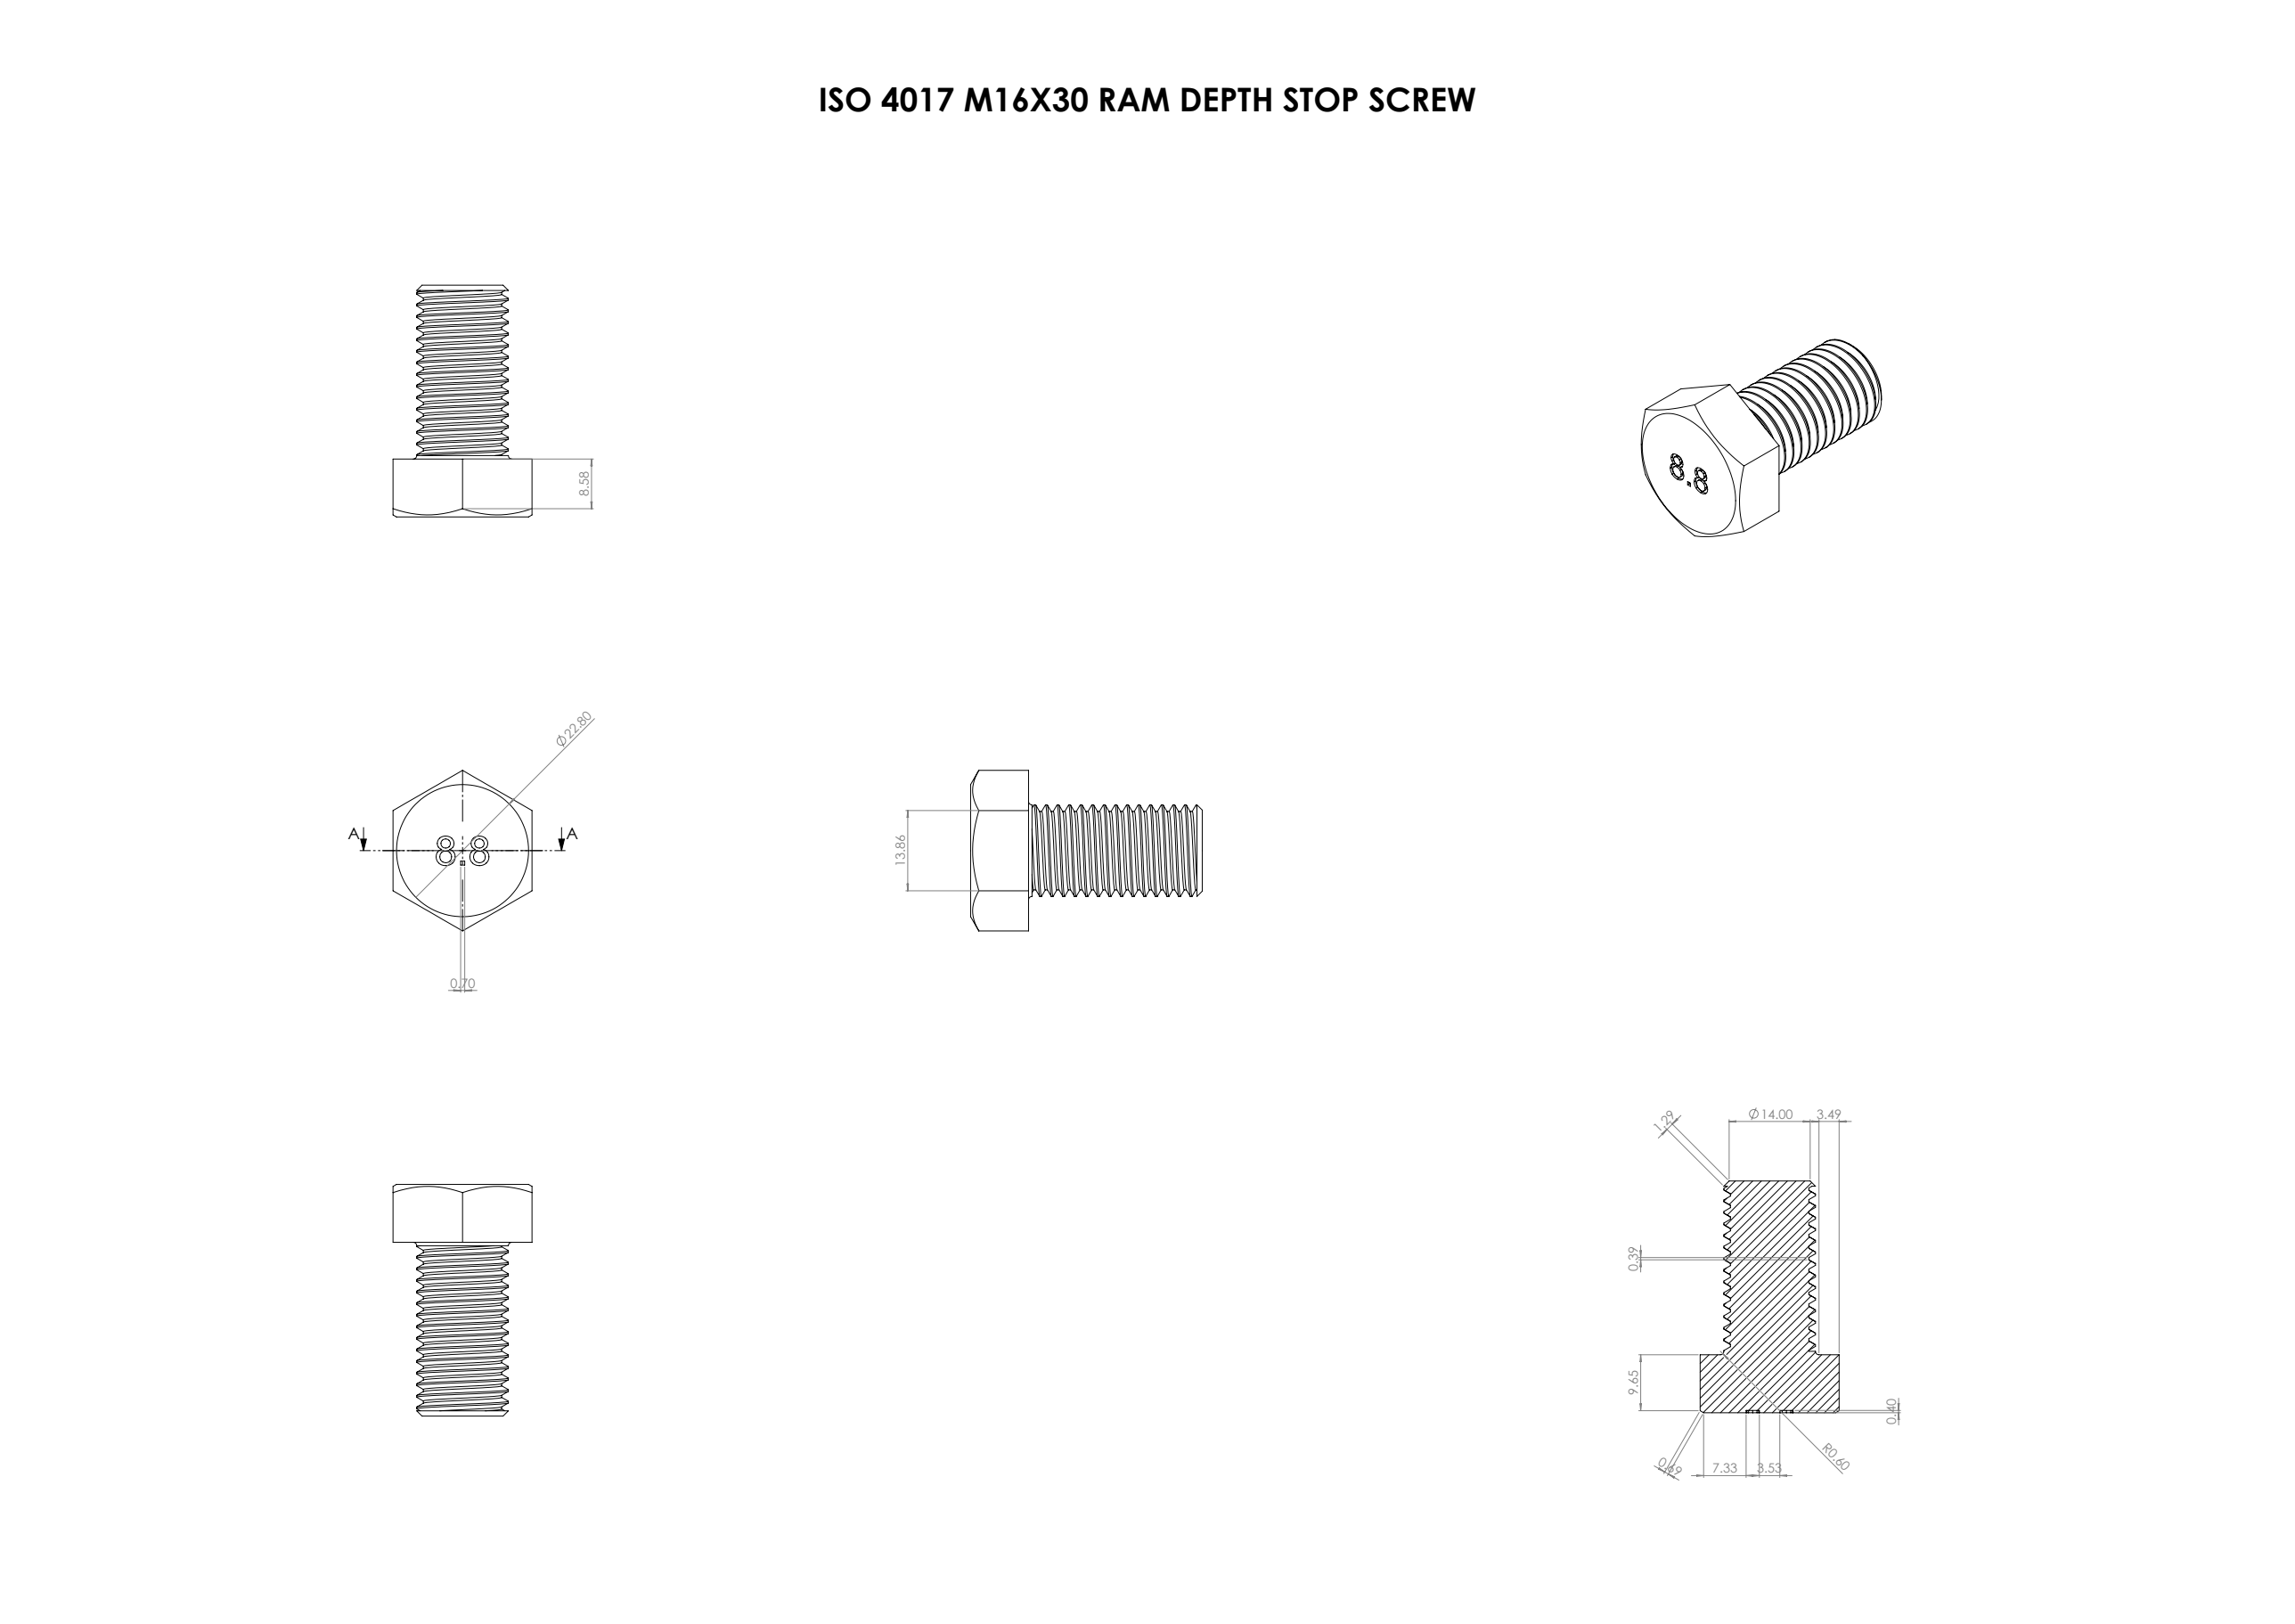
ISO-10303-21;
HEADER;
/* Generated by software containing ST-Developer
 * from STEP Tools, Inc. (www.steptools.com) 
 */

FILE_DESCRIPTION(
/* description */ (''),
/* implementation_level */ '2;1');

FILE_NAME(
/* name */ '13_ISO_4017_M16x30_Ram_Depth_Stop_Screw.step',
/* time_stamp */ '2026-10-19T23:58:09-07:00',
/* author */ (''),
/* organization */ (''),
/* preprocessor_version */ 'ST-DEVELOPER v20.2',
/* originating_system */ 'Autodesk Translation Framework v15.15.0.0',
/* authorisation */ '');

FILE_SCHEMA (('AP203_CONFIGURATION_CONTROLLED_3D_DESIGN_OF_MECHANICAL_PARTS_AND_ASSEMBLIES_MIM_LF { 1 0 10303 203 3 1 4 }',
'AUTOMOTIVE_DESIGN { 1 0 10303 214 3 1 1 }','INTEGRATED_CNC_SCHEMA','MODEL_BASED_INTEGRATED_MANUFACTURING_SCHEMA',
'PROCESS_PLANNING_SCHEMA','AP242_MANAGED_MODEL_BASED_3D_ENGINEERING_MIM_LF { 1 0 10303 442 3 1 4 }'));
ENDSEC;

DATA;
#10=MECHANICAL_DESIGN_GEOMETRIC_PRESENTATION_REPRESENTATION('',(#466),#70757);
#170=TOROIDAL_SURFACE('',#28944,0.8511,0.06);
#263=(
BOUNDED_CURVE()
B_SPLINE_CURVE(2,(#70654,#70655,#70656),.UNSPECIFIED.,.F.,.F.)
B_SPLINE_CURVE_WITH_KNOTS((3,3),(0.0830692064483412,1.5163968327409),
 .UNSPECIFIED.)
CURVE()
GEOMETRIC_REPRESENTATION_ITEM()
RATIONAL_B_SPLINE_CURVE((1.01933756729741,1.17702963774851,1.01933756729741))
REPRESENTATION_ITEM('')
);
#264=(
BOUNDED_CURVE()
B_SPLINE_CURVE(2,(#70658,#70659,#70660),.UNSPECIFIED.,.F.,.F.)
B_SPLINE_CURVE_WITH_KNOTS((3,3),(0.0830692064483407,1.5163968327409),
 .UNSPECIFIED.)
CURVE()
GEOMETRIC_REPRESENTATION_ITEM()
RATIONAL_B_SPLINE_CURVE((1.01933756729741,1.17702963774851,1.01933756729741))
REPRESENTATION_ITEM('')
);
#265=(
BOUNDED_CURVE()
B_SPLINE_CURVE(2,(#70662,#70663,#70664),.UNSPECIFIED.,.F.,.F.)
B_SPLINE_CURVE_WITH_KNOTS((3,3),(0.0830692064483414,1.5163968327409),
 .UNSPECIFIED.)
CURVE()
GEOMETRIC_REPRESENTATION_ITEM()
RATIONAL_B_SPLINE_CURVE((1.01933756729741,1.17702963774851,1.01933756729741))
REPRESENTATION_ITEM('')
);
#266=(
BOUNDED_CURVE()
B_SPLINE_CURVE(2,(#70666,#70667,#70668),.UNSPECIFIED.,.F.,.F.)
B_SPLINE_CURVE_WITH_KNOTS((3,3),(0.0830692064483412,1.5163968327409),
 .UNSPECIFIED.)
CURVE()
GEOMETRIC_REPRESENTATION_ITEM()
RATIONAL_B_SPLINE_CURVE((1.01933756729741,1.17702963774851,1.01933756729741))
REPRESENTATION_ITEM('')
);
#267=(
BOUNDED_CURVE()
B_SPLINE_CURVE(2,(#70670,#70671,#70672),.UNSPECIFIED.,.F.,.F.)
B_SPLINE_CURVE_WITH_KNOTS((3,3),(0.799733019594622,1.5163968327409),
 .UNSPECIFIED.)
CURVE()
GEOMETRIC_REPRESENTATION_ITEM()
RATIONAL_B_SPLINE_CURVE((1.09818360252296,1.09818360252296,1.01933756729741))
REPRESENTATION_ITEM('')
);
#268=(
BOUNDED_CURVE()
B_SPLINE_CURVE(2,(#70677,#70678,#70679),.UNSPECIFIED.,.F.,.F.)
B_SPLINE_CURVE_WITH_KNOTS((3,3),(0.083069206448341,0.799733019594622),
 .UNSPECIFIED.)
CURVE()
GEOMETRIC_REPRESENTATION_ITEM()
RATIONAL_B_SPLINE_CURVE((1.01933756729741,1.09818360252296,1.09818360252296))
REPRESENTATION_ITEM('')
);
#269=(
BOUNDED_CURVE()
B_SPLINE_CURVE(2,(#70680,#70681,#70682),.UNSPECIFIED.,.F.,.F.)
B_SPLINE_CURVE_WITH_KNOTS((3,3),(0.0830692064483408,1.5163968327409),
 .UNSPECIFIED.)
CURVE()
GEOMETRIC_REPRESENTATION_ITEM()
RATIONAL_B_SPLINE_CURVE((1.01933756729741,1.17702963774851,1.01933756729741))
REPRESENTATION_ITEM('')
);
#309=B_SPLINE_SURFACE_WITH_KNOTS('',2,1,((#67768,#67769),(#67770,#67771),
(#67772,#67773)),.UNSPECIFIED.,.F.,.F.,.F.,(3,3),(2,2),(0.,1.),(0.,0.04),
 .UNSPECIFIED.);
#310=B_SPLINE_SURFACE_WITH_KNOTS('',2,1,((#67786,#67787),(#67788,#67789),
(#67790,#67791)),.UNSPECIFIED.,.F.,.F.,.F.,(3,3),(2,2),(0.,1.),(0.,0.04),
 .UNSPECIFIED.);
#311=B_SPLINE_SURFACE_WITH_KNOTS('',2,1,((#67801,#67802),(#67803,#67804),
(#67805,#67806)),.UNSPECIFIED.,.F.,.F.,.F.,(3,3),(2,2),(0.,1.),(0.,0.04),
 .UNSPECIFIED.);
#312=B_SPLINE_SURFACE_WITH_KNOTS('',2,1,((#67816,#67817),(#67818,#67819),
(#67820,#67821)),.UNSPECIFIED.,.F.,.F.,.F.,(3,3),(2,2),(0.,1.),(0.,0.04),
 .UNSPECIFIED.);
#313=B_SPLINE_SURFACE_WITH_KNOTS('',2,1,((#67831,#67832),(#67833,#67834),
(#67835,#67836)),.UNSPECIFIED.,.F.,.F.,.F.,(3,3),(2,2),(0.,1.),(0.,0.04),
 .UNSPECIFIED.);
#314=B_SPLINE_SURFACE_WITH_KNOTS('',2,1,((#67846,#67847),(#67848,#67849),
(#67850,#67851)),.UNSPECIFIED.,.F.,.F.,.F.,(3,3),(2,2),(0.,1.),(0.,0.04),
 .UNSPECIFIED.);
#315=B_SPLINE_SURFACE_WITH_KNOTS('',2,1,((#67861,#67862),(#67863,#67864),
(#67865,#67866)),.UNSPECIFIED.,.F.,.F.,.F.,(3,3),(2,2),(0.,1.),(0.,0.04),
 .UNSPECIFIED.);
#316=B_SPLINE_SURFACE_WITH_KNOTS('',2,1,((#67876,#67877),(#67878,#67879),
(#67880,#67881)),.UNSPECIFIED.,.F.,.F.,.F.,(3,3),(2,2),(0.,1.),(0.,0.04),
 .UNSPECIFIED.);
#317=B_SPLINE_SURFACE_WITH_KNOTS('',2,1,((#67888,#67889),(#67890,#67891),
(#67892,#67893)),.UNSPECIFIED.,.F.,.F.,.F.,(3,3),(2,2),(0.,1.),(0.,0.04),
 .UNSPECIFIED.);
#318=B_SPLINE_SURFACE_WITH_KNOTS('',2,1,((#67906,#67907),(#67908,#67909),
(#67910,#67911)),.UNSPECIFIED.,.F.,.F.,.F.,(3,3),(2,2),(0.,1.),(0.,0.04),
 .UNSPECIFIED.);
#319=B_SPLINE_SURFACE_WITH_KNOTS('',2,1,((#67921,#67922),(#67923,#67924),
(#67925,#67926)),.UNSPECIFIED.,.F.,.F.,.F.,(3,3),(2,2),(0.,1.),(0.,0.04),
 .UNSPECIFIED.);
#320=B_SPLINE_SURFACE_WITH_KNOTS('',2,1,((#67936,#67937),(#67938,#67939),
(#67940,#67941)),.UNSPECIFIED.,.F.,.F.,.F.,(3,3),(2,2),(0.,1.),(0.,0.04),
 .UNSPECIFIED.);
#321=B_SPLINE_SURFACE_WITH_KNOTS('',2,1,((#67951,#67952),(#67953,#67954),
(#67955,#67956)),.UNSPECIFIED.,.F.,.F.,.F.,(3,3),(2,2),(0.,1.),(0.,0.04),
 .UNSPECIFIED.);
#322=B_SPLINE_SURFACE_WITH_KNOTS('',2,1,((#67966,#67967),(#67968,#67969),
(#67970,#67971)),.UNSPECIFIED.,.F.,.F.,.F.,(3,3),(2,2),(0.,1.),(0.,0.04),
 .UNSPECIFIED.);
#323=B_SPLINE_SURFACE_WITH_KNOTS('',2,1,((#67981,#67982),(#67983,#67984),
(#67985,#67986)),.UNSPECIFIED.,.F.,.F.,.F.,(3,3),(2,2),(0.,1.),(0.,0.04),
 .UNSPECIFIED.);
#324=B_SPLINE_SURFACE_WITH_KNOTS('',2,1,((#67996,#67997),(#67998,#67999),
(#68000,#68001)),.UNSPECIFIED.,.F.,.F.,.F.,(3,3),(2,2),(0.,1.),(0.,0.04),
 .UNSPECIFIED.);
#325=B_SPLINE_SURFACE_WITH_KNOTS('',2,1,((#68011,#68012),(#68013,#68014),
(#68015,#68016)),.UNSPECIFIED.,.F.,.F.,.F.,(3,3),(2,2),(0.,1.),(0.,0.04),
 .UNSPECIFIED.);
#326=B_SPLINE_SURFACE_WITH_KNOTS('',2,1,((#68023,#68024),(#68025,#68026),
(#68027,#68028)),.UNSPECIFIED.,.F.,.F.,.F.,(3,3),(2,2),(0.,1.),(0.,0.04),
 .UNSPECIFIED.);
#327=B_SPLINE_SURFACE_WITH_KNOTS('',2,1,((#68041,#68042),(#68043,#68044),
(#68045,#68046)),.UNSPECIFIED.,.F.,.F.,.F.,(3,3),(2,2),(0.,1.),(0.,0.04),
 .UNSPECIFIED.);
#328=B_SPLINE_SURFACE_WITH_KNOTS('',2,1,((#68056,#68057),(#68058,#68059),
(#68060,#68061)),.UNSPECIFIED.,.F.,.F.,.F.,(3,3),(2,2),(0.,1.),(0.,0.04),
 .UNSPECIFIED.);
#329=B_SPLINE_SURFACE_WITH_KNOTS('',2,1,((#68071,#68072),(#68073,#68074),
(#68075,#68076)),.UNSPECIFIED.,.F.,.F.,.F.,(3,3),(2,2),(0.,1.),(0.,0.04),
 .UNSPECIFIED.);
#330=B_SPLINE_SURFACE_WITH_KNOTS('',2,1,((#68086,#68087),(#68088,#68089),
(#68090,#68091)),.UNSPECIFIED.,.F.,.F.,.F.,(3,3),(2,2),(0.,1.),(0.,0.04),
 .UNSPECIFIED.);
#331=B_SPLINE_SURFACE_WITH_KNOTS('',2,1,((#68101,#68102),(#68103,#68104),
(#68105,#68106)),.UNSPECIFIED.,.F.,.F.,.F.,(3,3),(2,2),(0.,1.),(0.,0.04),
 .UNSPECIFIED.);
#332=B_SPLINE_SURFACE_WITH_KNOTS('',2,1,((#68116,#68117),(#68118,#68119),
(#68120,#68121)),.UNSPECIFIED.,.F.,.F.,.F.,(3,3),(2,2),(0.,1.),(0.,0.04),
 .UNSPECIFIED.);
#333=B_SPLINE_SURFACE_WITH_KNOTS('',2,1,((#68131,#68132),(#68133,#68134),
(#68135,#68136)),.UNSPECIFIED.,.F.,.F.,.F.,(3,3),(2,2),(0.,1.),(0.,0.04),
 .UNSPECIFIED.);
#334=B_SPLINE_SURFACE_WITH_KNOTS('',2,1,((#68146,#68147),(#68148,#68149),
(#68150,#68151)),.UNSPECIFIED.,.F.,.F.,.F.,(3,3),(2,2),(0.,1.),(0.,0.04),
 .UNSPECIFIED.);
#335=B_SPLINE_SURFACE_WITH_KNOTS('',2,1,((#68161,#68162),(#68163,#68164),
(#68165,#68166)),.UNSPECIFIED.,.F.,.F.,.F.,(3,3),(2,2),(0.,1.),(0.,0.04),
 .UNSPECIFIED.);
#336=B_SPLINE_SURFACE_WITH_KNOTS('',2,1,((#68176,#68177),(#68178,#68179),
(#68180,#68181)),.UNSPECIFIED.,.F.,.F.,.F.,(3,3),(2,2),(0.,1.),(0.,0.04),
 .UNSPECIFIED.);
#337=B_SPLINE_SURFACE_WITH_KNOTS('',2,1,((#68191,#68192),(#68193,#68194),
(#68195,#68196)),.UNSPECIFIED.,.F.,.F.,.F.,(3,3),(2,2),(0.,1.),(0.,0.04),
 .UNSPECIFIED.);
#338=B_SPLINE_SURFACE_WITH_KNOTS('',2,1,((#68206,#68207),(#68208,#68209),
(#68210,#68211)),.UNSPECIFIED.,.F.,.F.,.F.,(3,3),(2,2),(0.,1.),(0.,0.04),
 .UNSPECIFIED.);
#339=B_SPLINE_SURFACE_WITH_KNOTS('',2,1,((#68221,#68222),(#68223,#68224),
(#68225,#68226)),.UNSPECIFIED.,.F.,.F.,.F.,(3,3),(2,2),(0.,1.),(0.,0.04),
 .UNSPECIFIED.);
#340=B_SPLINE_SURFACE_WITH_KNOTS('',2,1,((#68236,#68237),(#68238,#68239),
(#68240,#68241)),.UNSPECIFIED.,.F.,.F.,.F.,(3,3),(2,2),(0.,1.),(0.,0.04),
 .UNSPECIFIED.);
#341=B_SPLINE_SURFACE_WITH_KNOTS('',2,1,((#68251,#68252),(#68253,#68254),
(#68255,#68256)),.UNSPECIFIED.,.F.,.F.,.F.,(3,3),(2,2),(0.,1.),(0.,0.04),
 .UNSPECIFIED.);
#342=B_SPLINE_SURFACE_WITH_KNOTS('',2,1,((#68289,#68290),(#68291,#68292),
(#68293,#68294)),.UNSPECIFIED.,.F.,.F.,.F.,(3,3),(2,2),(0.,1.),(0.,0.04),
 .UNSPECIFIED.);
#343=B_SPLINE_SURFACE_WITH_KNOTS('',2,1,((#68307,#68308),(#68309,#68310),
(#68311,#68312)),.UNSPECIFIED.,.F.,.F.,.F.,(3,3),(2,2),(0.,1.),(0.,0.04),
 .UNSPECIFIED.);
#344=B_SPLINE_SURFACE_WITH_KNOTS('',2,1,((#68322,#68323),(#68324,#68325),
(#68326,#68327)),.UNSPECIFIED.,.F.,.F.,.F.,(3,3),(2,2),(0.,1.),(0.,0.04),
 .UNSPECIFIED.);
#345=B_SPLINE_SURFACE_WITH_KNOTS('',2,1,((#68337,#68338),(#68339,#68340),
(#68341,#68342)),.UNSPECIFIED.,.F.,.F.,.F.,(3,3),(2,2),(0.,1.),(0.,0.04),
 .UNSPECIFIED.);
#346=B_SPLINE_SURFACE_WITH_KNOTS('',2,1,((#68352,#68353),(#68354,#68355),
(#68356,#68357)),.UNSPECIFIED.,.F.,.F.,.F.,(3,3),(2,2),(0.,1.),(0.,0.04),
 .UNSPECIFIED.);
#347=B_SPLINE_SURFACE_WITH_KNOTS('',2,1,((#68367,#68368),(#68369,#68370),
(#68371,#68372)),.UNSPECIFIED.,.F.,.F.,.F.,(3,3),(2,2),(0.,1.),(0.,0.04),
 .UNSPECIFIED.);
#348=B_SPLINE_SURFACE_WITH_KNOTS('',2,1,((#68382,#68383),(#68384,#68385),
(#68386,#68387)),.UNSPECIFIED.,.F.,.F.,.F.,(3,3),(2,2),(0.,1.),(0.,0.04),
 .UNSPECIFIED.);
#349=B_SPLINE_SURFACE_WITH_KNOTS('',2,1,((#68397,#68398),(#68399,#68400),
(#68401,#68402)),.UNSPECIFIED.,.F.,.F.,.F.,(3,3),(2,2),(0.,1.),(0.,0.04),
 .UNSPECIFIED.);
#350=B_SPLINE_SURFACE_WITH_KNOTS('',2,1,((#68409,#68410),(#68411,#68412),
(#68413,#68414)),.UNSPECIFIED.,.F.,.F.,.F.,(3,3),(2,2),(0.,1.),(0.,0.04),
 .UNSPECIFIED.);
#351=B_SPLINE_SURFACE_WITH_KNOTS('',2,1,((#68427,#68428),(#68429,#68430),
(#68431,#68432)),.UNSPECIFIED.,.F.,.F.,.F.,(3,3),(2,2),(0.,1.),(0.,0.04),
 .UNSPECIFIED.);
#352=B_SPLINE_SURFACE_WITH_KNOTS('',2,1,((#68442,#68443),(#68444,#68445),
(#68446,#68447)),.UNSPECIFIED.,.F.,.F.,.F.,(3,3),(2,2),(0.,1.),(0.,0.04),
 .UNSPECIFIED.);
#353=B_SPLINE_SURFACE_WITH_KNOTS('',2,1,((#68457,#68458),(#68459,#68460),
(#68461,#68462)),.UNSPECIFIED.,.F.,.F.,.F.,(3,3),(2,2),(0.,1.),(0.,0.04),
 .UNSPECIFIED.);
#354=B_SPLINE_SURFACE_WITH_KNOTS('',2,1,((#68472,#68473),(#68474,#68475),
(#68476,#68477)),.UNSPECIFIED.,.F.,.F.,.F.,(3,3),(2,2),(0.,1.),(0.,0.04),
 .UNSPECIFIED.);
#355=B_SPLINE_SURFACE_WITH_KNOTS('',2,1,((#68487,#68488),(#68489,#68490),
(#68491,#68492)),.UNSPECIFIED.,.F.,.F.,.F.,(3,3),(2,2),(0.,1.),(0.,0.04),
 .UNSPECIFIED.);
#356=B_SPLINE_SURFACE_WITH_KNOTS('',2,1,((#68502,#68503),(#68504,#68505),
(#68506,#68507)),.UNSPECIFIED.,.F.,.F.,.F.,(3,3),(2,2),(0.,1.),(0.,0.04),
 .UNSPECIFIED.);
#357=B_SPLINE_SURFACE_WITH_KNOTS('',2,1,((#68517,#68518),(#68519,#68520),
(#68521,#68522)),.UNSPECIFIED.,.F.,.F.,.F.,(3,3),(2,2),(0.,1.),(0.,0.04),
 .UNSPECIFIED.);
#358=B_SPLINE_SURFACE_WITH_KNOTS('',2,1,((#68532,#68533),(#68534,#68535),
(#68536,#68537)),.UNSPECIFIED.,.F.,.F.,.F.,(3,3),(2,2),(0.,1.),(0.,0.04),
 .UNSPECIFIED.);
#359=B_SPLINE_SURFACE_WITH_KNOTS('',2,1,((#68544,#68545),(#68546,#68547),
(#68548,#68549)),.UNSPECIFIED.,.F.,.F.,.F.,(3,3),(2,2),(0.,1.),(0.,0.04),
 .UNSPECIFIED.);
#360=B_SPLINE_SURFACE_WITH_KNOTS('',2,1,((#68562,#68563),(#68564,#68565),
(#68566,#68567)),.UNSPECIFIED.,.F.,.F.,.F.,(3,3),(2,2),(0.,1.),(0.,0.04),
 .UNSPECIFIED.);
#361=B_SPLINE_SURFACE_WITH_KNOTS('',2,1,((#68577,#68578),(#68579,#68580),
(#68581,#68582)),.UNSPECIFIED.,.F.,.F.,.F.,(3,3),(2,2),(0.,1.),(0.,0.04),
 .UNSPECIFIED.);
#362=B_SPLINE_SURFACE_WITH_KNOTS('',2,1,((#68592,#68593),(#68594,#68595),
(#68596,#68597)),.UNSPECIFIED.,.F.,.F.,.F.,(3,3),(2,2),(0.,1.),(0.,0.04),
 .UNSPECIFIED.);
#363=B_SPLINE_SURFACE_WITH_KNOTS('',2,1,((#68607,#68608),(#68609,#68610),
(#68611,#68612)),.UNSPECIFIED.,.F.,.F.,.F.,(3,3),(2,2),(0.,1.),(0.,0.04),
 .UNSPECIFIED.);
#364=B_SPLINE_SURFACE_WITH_KNOTS('',2,1,((#68622,#68623),(#68624,#68625),
(#68626,#68627)),.UNSPECIFIED.,.F.,.F.,.F.,(3,3),(2,2),(0.,1.),(0.,0.04),
 .UNSPECIFIED.);
#365=B_SPLINE_SURFACE_WITH_KNOTS('',2,1,((#68637,#68638),(#68639,#68640),
(#68641,#68642)),.UNSPECIFIED.,.F.,.F.,.F.,(3,3),(2,2),(0.,1.),(0.,0.04),
 .UNSPECIFIED.);
#366=B_SPLINE_SURFACE_WITH_KNOTS('',2,1,((#68652,#68653),(#68654,#68655),
(#68656,#68657)),.UNSPECIFIED.,.F.,.F.,.F.,(3,3),(2,2),(0.,1.),(0.,0.04),
 .UNSPECIFIED.);
#367=B_SPLINE_SURFACE_WITH_KNOTS('',2,1,((#68667,#68668),(#68669,#68670),
(#68671,#68672)),.UNSPECIFIED.,.F.,.F.,.F.,(3,3),(2,2),(0.,1.),(0.,0.04),
 .UNSPECIFIED.);
#368=B_SPLINE_SURFACE_WITH_KNOTS('',2,1,((#68682,#68683),(#68684,#68685),
(#68686,#68687)),.UNSPECIFIED.,.F.,.F.,.F.,(3,3),(2,2),(0.,1.),(0.,0.04),
 .UNSPECIFIED.);
#369=B_SPLINE_SURFACE_WITH_KNOTS('',2,1,((#68697,#68698),(#68699,#68700),
(#68701,#68702)),.UNSPECIFIED.,.F.,.F.,.F.,(3,3),(2,2),(0.,1.),(0.,0.04),
 .UNSPECIFIED.);
#370=B_SPLINE_SURFACE_WITH_KNOTS('',2,1,((#68712,#68713),(#68714,#68715),
(#68716,#68717)),.UNSPECIFIED.,.F.,.F.,.F.,(3,3),(2,2),(0.,1.),(0.,0.04),
 .UNSPECIFIED.);
#371=B_SPLINE_SURFACE_WITH_KNOTS('',2,1,((#68727,#68728),(#68729,#68730),
(#68731,#68732)),.UNSPECIFIED.,.F.,.F.,.F.,(3,3),(2,2),(0.,1.),(0.,0.04),
 .UNSPECIFIED.);
#372=B_SPLINE_SURFACE_WITH_KNOTS('',2,1,((#68742,#68743),(#68744,#68745),
(#68746,#68747)),.UNSPECIFIED.,.F.,.F.,.F.,(3,3),(2,2),(0.,1.),(0.,0.04),
 .UNSPECIFIED.);
#373=B_SPLINE_SURFACE_WITH_KNOTS('',2,1,((#68757,#68758),(#68759,#68760),
(#68761,#68762)),.UNSPECIFIED.,.F.,.F.,.F.,(3,3),(2,2),(0.,1.),(0.,0.04),
 .UNSPECIFIED.);
#374=B_SPLINE_SURFACE_WITH_KNOTS('',2,1,((#68772,#68773),(#68774,#68775),
(#68776,#68777)),.UNSPECIFIED.,.F.,.F.,.F.,(3,3),(2,2),(0.,1.),(0.,0.04),
 .UNSPECIFIED.);
#375=B_SPLINE_SURFACE_WITH_KNOTS('',3,3,((#68946,#68947,#68948,#68949,#68950,
#68951,#68952,#68953,#68954,#68955,#68956,#68957,#68958,#68959,#68960,#68961,
#68962,#68963,#68964,#68965,#68966,#68967,#68968,#68969,#68970,#68971,#68972,
#68973,#68974,#68975,#68976,#68977,#68978,#68979,#68980,#68981,#68982,#68983,
#68984,#68985,#68986,#68987,#68988,#68989,#68990,#68991,#68992,#68993,#68994,
#68995,#68996,#68997,#68998,#68999,#69000,#69001,#69002,#69003,#69004,#69005,
#69006,#69007,#69008,#69009,#69010,#69011,#69012,#69013,#69014,#69015,#69016,
#69017,#69018,#69019,#69020,#69021,#69022,#69023,#69024,#69025,#69026,#69027,
#69028,#69029,#69030,#69031,#69032,#69033,#69034,#69035,#69036,#69037,#69038,
#69039,#69040,#69041,#69042,#69043,#69044,#69045,#69046,#69047,#69048,#69049,
#69050,#69051,#69052,#69053,#69054,#69055,#69056,#69057,#69058,#69059,#69060,
#69061,#69062,#69063,#69064,#69065,#69066,#69067,#69068,#69069,#69070,#69071,
#69072,#69073,#69074,#69075,#69076,#69077,#69078,#69079,#69080,#69081,#69082,
#69083,#69084,#69085,#69086,#69087,#69088,#69089,#69090,#69091,#69092,#69093,
#69094,#69095,#69096,#69097,#69098,#69099,#69100,#69101,#69102,#69103,#69104,
#69105,#69106,#69107,#69108,#69109,#69110,#69111,#69112,#69113,#69114,#69115,
#69116,#69117,#69118,#69119,#69120,#69121,#69122,#69123,#69124,#69125,#69126,
#69127,#69128,#69129,#69130,#69131,#69132),(#69133,#69134,#69135,#69136,
#69137,#69138,#69139,#69140,#69141,#69142,#69143,#69144,#69145,#69146,#69147,
#69148,#69149,#69150,#69151,#69152,#69153,#69154,#69155,#69156,#69157,#69158,
#69159,#69160,#69161,#69162,#69163,#69164,#69165,#69166,#69167,#69168,#69169,
#69170,#69171,#69172,#69173,#69174,#69175,#69176,#69177,#69178,#69179,#69180,
#69181,#69182,#69183,#69184,#69185,#69186,#69187,#69188,#69189,#69190,#69191,
#69192,#69193,#69194,#69195,#69196,#69197,#69198,#69199,#69200,#69201,#69202,
#69203,#69204,#69205,#69206,#69207,#69208,#69209,#69210,#69211,#69212,#69213,
#69214,#69215,#69216,#69217,#69218,#69219,#69220,#69221,#69222,#69223,#69224,
#69225,#69226,#69227,#69228,#69229,#69230,#69231,#69232,#69233,#69234,#69235,
#69236,#69237,#69238,#69239,#69240,#69241,#69242,#69243,#69244,#69245,#69246,
#69247,#69248,#69249,#69250,#69251,#69252,#69253,#69254,#69255,#69256,#69257,
#69258,#69259,#69260,#69261,#69262,#69263,#69264,#69265,#69266,#69267,#69268,
#69269,#69270,#69271,#69272,#69273,#69274,#69275,#69276,#69277,#69278,#69279,
#69280,#69281,#69282,#69283,#69284,#69285,#69286,#69287,#69288,#69289,#69290,
#69291,#69292,#69293,#69294,#69295,#69296,#69297,#69298,#69299,#69300,#69301,
#69302,#69303,#69304,#69305,#69306,#69307,#69308,#69309,#69310,#69311,#69312,
#69313,#69314,#69315,#69316,#69317,#69318,#69319),(#69320,#69321,#69322,
#69323,#69324,#69325,#69326,#69327,#69328,#69329,#69330,#69331,#69332,#69333,
#69334,#69335,#69336,#69337,#69338,#69339,#69340,#69341,#69342,#69343,#69344,
#69345,#69346,#69347,#69348,#69349,#69350,#69351,#69352,#69353,#69354,#69355,
#69356,#69357,#69358,#69359,#69360,#69361,#69362,#69363,#69364,#69365,#69366,
#69367,#69368,#69369,#69370,#69371,#69372,#69373,#69374,#69375,#69376,#69377,
#69378,#69379,#69380,#69381,#69382,#69383,#69384,#69385,#69386,#69387,#69388,
#69389,#69390,#69391,#69392,#69393,#69394,#69395,#69396,#69397,#69398,#69399,
#69400,#69401,#69402,#69403,#69404,#69405,#69406,#69407,#69408,#69409,#69410,
#69411,#69412,#69413,#69414,#69415,#69416,#69417,#69418,#69419,#69420,#69421,
#69422,#69423,#69424,#69425,#69426,#69427,#69428,#69429,#69430,#69431,#69432,
#69433,#69434,#69435,#69436,#69437,#69438,#69439,#69440,#69441,#69442,#69443,
#69444,#69445,#69446,#69447,#69448,#69449,#69450,#69451,#69452,#69453,#69454,
#69455,#69456,#69457,#69458,#69459,#69460,#69461,#69462,#69463,#69464,#69465,
#69466,#69467,#69468,#69469,#69470,#69471,#69472,#69473,#69474,#69475,#69476,
#69477,#69478,#69479,#69480,#69481,#69482,#69483,#69484,#69485,#69486,#69487,
#69488,#69489,#69490,#69491,#69492,#69493,#69494,#69495,#69496,#69497,#69498,
#69499,#69500,#69501,#69502,#69503,#69504,#69505,#69506),(#69507,#69508,
#69509,#69510,#69511,#69512,#69513,#69514,#69515,#69516,#69517,#69518,#69519,
#69520,#69521,#69522,#69523,#69524,#69525,#69526,#69527,#69528,#69529,#69530,
#69531,#69532,#69533,#69534,#69535,#69536,#69537,#69538,#69539,#69540,#69541,
#69542,#69543,#69544,#69545,#69546,#69547,#69548,#69549,#69550,#69551,#69552,
#69553,#69554,#69555,#69556,#69557,#69558,#69559,#69560,#69561,#69562,#69563,
#69564,#69565,#69566,#69567,#69568,#69569,#69570,#69571,#69572,#69573,#69574,
#69575,#69576,#69577,#69578,#69579,#69580,#69581,#69582,#69583,#69584,#69585,
#69586,#69587,#69588,#69589,#69590,#69591,#69592,#69593,#69594,#69595,#69596,
#69597,#69598,#69599,#69600,#69601,#69602,#69603,#69604,#69605,#69606,#69607,
#69608,#69609,#69610,#69611,#69612,#69613,#69614,#69615,#69616,#69617,#69618,
#69619,#69620,#69621,#69622,#69623,#69624,#69625,#69626,#69627,#69628,#69629,
#69630,#69631,#69632,#69633,#69634,#69635,#69636,#69637,#69638,#69639,#69640,
#69641,#69642,#69643,#69644,#69645,#69646,#69647,#69648,#69649,#69650,#69651,
#69652,#69653,#69654,#69655,#69656,#69657,#69658,#69659,#69660,#69661,#69662,
#69663,#69664,#69665,#69666,#69667,#69668,#69669,#69670,#69671,#69672,#69673,
#69674,#69675,#69676,#69677,#69678,#69679,#69680,#69681,#69682,#69683,#69684,
#69685,#69686,#69687,#69688,#69689,#69690,#69691,#69692,#69693)),
 .UNSPECIFIED.,.F.,.F.,.F.,(4,4),(4,1,1,1,1,1,1,1,1,1,1,1,1,1,1,1,1,1,1,
1,1,1,1,1,1,1,1,1,1,1,1,1,1,1,1,1,1,1,1,1,1,1,1,1,1,1,1,1,1,1,1,1,1,1,1,
1,1,1,1,1,1,1,1,1,1,1,1,1,1,1,1,1,1,1,1,1,1,1,1,1,1,1,1,1,1,1,1,1,1,1,1,
1,1,1,1,1,1,1,1,1,1,1,1,1,1,1,1,1,1,1,1,1,1,1,1,1,1,1,1,1,1,1,1,1,1,1,1,
1,1,1,1,1,1,1,1,1,1,1,1,1,1,1,1,1,1,1,1,1,1,1,1,1,1,1,1,1,1,1,1,1,1,1,1,
1,1,1,1,1,1,1,1,1,1,1,1,1,1,1,1,1,1,1,1,1,4),(0.,0.132097741590586),(8.30112925462619,
8.79882392626099,9.29651859789579,9.79421326953059,10.2919079411654,10.7896026128002,
11.287297284435,11.7849919560698,12.2826866277046,12.7803812993394,13.2780759709742,
13.775770642609,14.2734653142438,14.7711599858786,15.2688546575134,15.7665493291482,
16.264244000783,16.7619386724178,17.2596333440526,17.7573280156874,18.2550226873222,
18.752717358957,19.2504120305918,19.7481067022266,20.2458013738614,20.7434960454962,
21.241190717131,21.7388853887658,22.2365800604006,22.7342747320354,23.2319694036702,
23.7296640753051,24.2273587469399,24.7250534185747,25.2227480902095,25.7204427618443,
26.2181374334791,26.7158321051139,27.2135267767487,27.7112214483835,28.2089161200183,
28.7066107916531,29.2043054632879,29.7020001349227,30.1996948065575,30.6973894781923,
31.1950841498271,31.6927788214619,32.1904734930967,32.6881681647315,33.1858628363663,
33.6835575080011,34.1812521796359,34.6789468512707,35.1766415229055,35.6743361945403,
36.1720308661751,36.6697255378099,37.1674202094447,37.6651148810795,38.1628095527143,
38.6605042243491,39.1581988959839,39.6558935676187,40.1535882392535,40.6512829108883,
41.1489775825231,41.6466722541579,42.1443669257927,42.6420615974275,43.1397562690623,
43.6374509406971,44.1351456123319,44.6328402839667,45.1305349556015,45.6282296272363,
46.1259242988711,46.6236189705059,47.1213136421407,47.6190083137756,48.1167029854104,
48.6143976570452,49.11209232868,49.6097870003148,50.1074816719496,50.6051763435844,
51.1028710152192,51.600565686854,52.0982603584888,52.5959550301236,53.0936497017584,
53.5913443733932,54.089039045028,54.5867337166628,55.0844283882976,55.5821230599324,
56.0798177315672,56.577512403202,57.0752070748368,57.5729017464716,58.0705964181064,
58.5682910897412,59.065985761376,59.5636804330108,60.0613751046456,60.5590697762804,
61.0567644479152,61.55445911955,62.0521537911848,62.5498484628196,63.0475431344544,
63.5452378060892,64.042932477724,64.5406271493588,65.0383218209936,65.5360164926284,
66.0337111642632,66.531405835898,67.0291005075328,67.5267951791676,68.0244898508024,
68.5221845224372,69.019879194072,69.5175738657069,70.0152685373416,70.5129632089764,
71.0106578806112,71.5083525522461,72.0060472238809,72.5037418955157,73.0014365671505,
73.4991312387853,73.9968259104201,74.4945205820549,74.9922152536897,75.4899099253245,
75.9876045969593,76.4852992685941,76.9829939402289,77.4806886118637,77.9783832834985,
78.4760779551333,78.9737726267681,79.4714672984029,79.9691619700377,80.4668566416725,
80.9645513133073,81.4622459849421,81.9599406565769,82.4576353282117,82.9553299998465,
83.4530246714813,83.9507193431161,84.4484140147509,84.9461086863857,85.4438033580205,
85.9414980296553,86.4391927012901,86.9368873729249,87.4345820445597,87.9322767161945,
88.4299713878293,88.9276660594641,89.4253607310989,89.9230554027337,90.4207500743685,
90.9184447460033,91.4161394176381,91.9138340892729,92.4115287609077,92.9092234325425,
93.4069181041774,93.9046127758121,94.4023074474469,94.9000021190817,95.3976967907166,
95.8953914623514,96.3930861339862,96.890780805621,97.3884754772558,97.8861701488906,
98.3838648205254,98.8815594921602,99.379254163795,99.8769488354298),
 .UNSPECIFIED.);
#376=B_SPLINE_SURFACE_WITH_KNOTS('',3,3,((#69884,#69885,#69886,#69887,#69888,
#69889,#69890,#69891,#69892,#69893,#69894,#69895,#69896,#69897,#69898,#69899,
#69900,#69901,#69902,#69903,#69904,#69905,#69906,#69907,#69908,#69909,#69910,
#69911,#69912,#69913,#69914,#69915,#69916,#69917,#69918,#69919,#69920,#69921,
#69922,#69923,#69924,#69925,#69926,#69927,#69928,#69929,#69930,#69931,#69932,
#69933,#69934,#69935,#69936,#69937,#69938,#69939,#69940,#69941,#69942,#69943,
#69944,#69945,#69946,#69947,#69948,#69949,#69950,#69951,#69952,#69953,#69954,
#69955,#69956,#69957,#69958,#69959,#69960,#69961,#69962,#69963,#69964,#69965,
#69966,#69967,#69968,#69969,#69970,#69971,#69972,#69973,#69974,#69975,#69976,
#69977,#69978,#69979,#69980,#69981,#69982,#69983,#69984,#69985,#69986,#69987,
#69988,#69989,#69990,#69991,#69992,#69993,#69994,#69995,#69996,#69997,#69998,
#69999,#70000,#70001,#70002,#70003,#70004,#70005,#70006,#70007,#70008,#70009,
#70010,#70011,#70012,#70013,#70014,#70015,#70016,#70017,#70018,#70019,#70020,
#70021,#70022,#70023,#70024,#70025,#70026,#70027,#70028,#70029,#70030,#70031,
#70032,#70033,#70034,#70035,#70036,#70037,#70038,#70039,#70040,#70041,#70042,
#70043,#70044,#70045,#70046,#70047,#70048,#70049,#70050,#70051,#70052,#70053,
#70054,#70055,#70056,#70057,#70058,#70059,#70060,#70061,#70062,#70063,#70064,
#70065,#70066,#70067,#70068,#70069,#70070),(#70071,#70072,#70073,#70074,
#70075,#70076,#70077,#70078,#70079,#70080,#70081,#70082,#70083,#70084,#70085,
#70086,#70087,#70088,#70089,#70090,#70091,#70092,#70093,#70094,#70095,#70096,
#70097,#70098,#70099,#70100,#70101,#70102,#70103,#70104,#70105,#70106,#70107,
#70108,#70109,#70110,#70111,#70112,#70113,#70114,#70115,#70116,#70117,#70118,
#70119,#70120,#70121,#70122,#70123,#70124,#70125,#70126,#70127,#70128,#70129,
#70130,#70131,#70132,#70133,#70134,#70135,#70136,#70137,#70138,#70139,#70140,
#70141,#70142,#70143,#70144,#70145,#70146,#70147,#70148,#70149,#70150,#70151,
#70152,#70153,#70154,#70155,#70156,#70157,#70158,#70159,#70160,#70161,#70162,
#70163,#70164,#70165,#70166,#70167,#70168,#70169,#70170,#70171,#70172,#70173,
#70174,#70175,#70176,#70177,#70178,#70179,#70180,#70181,#70182,#70183,#70184,
#70185,#70186,#70187,#70188,#70189,#70190,#70191,#70192,#70193,#70194,#70195,
#70196,#70197,#70198,#70199,#70200,#70201,#70202,#70203,#70204,#70205,#70206,
#70207,#70208,#70209,#70210,#70211,#70212,#70213,#70214,#70215,#70216,#70217,
#70218,#70219,#70220,#70221,#70222,#70223,#70224,#70225,#70226,#70227,#70228,
#70229,#70230,#70231,#70232,#70233,#70234,#70235,#70236,#70237,#70238,#70239,
#70240,#70241,#70242,#70243,#70244,#70245,#70246,#70247,#70248,#70249,#70250,
#70251,#70252,#70253,#70254,#70255,#70256,#70257),(#70258,#70259,#70260,
#70261,#70262,#70263,#70264,#70265,#70266,#70267,#70268,#70269,#70270,#70271,
#70272,#70273,#70274,#70275,#70276,#70277,#70278,#70279,#70280,#70281,#70282,
#70283,#70284,#70285,#70286,#70287,#70288,#70289,#70290,#70291,#70292,#70293,
#70294,#70295,#70296,#70297,#70298,#70299,#70300,#70301,#70302,#70303,#70304,
#70305,#70306,#70307,#70308,#70309,#70310,#70311,#70312,#70313,#70314,#70315,
#70316,#70317,#70318,#70319,#70320,#70321,#70322,#70323,#70324,#70325,#70326,
#70327,#70328,#70329,#70330,#70331,#70332,#70333,#70334,#70335,#70336,#70337,
#70338,#70339,#70340,#70341,#70342,#70343,#70344,#70345,#70346,#70347,#70348,
#70349,#70350,#70351,#70352,#70353,#70354,#70355,#70356,#70357,#70358,#70359,
#70360,#70361,#70362,#70363,#70364,#70365,#70366,#70367,#70368,#70369,#70370,
#70371,#70372,#70373,#70374,#70375,#70376,#70377,#70378,#70379,#70380,#70381,
#70382,#70383,#70384,#70385,#70386,#70387,#70388,#70389,#70390,#70391,#70392,
#70393,#70394,#70395,#70396,#70397,#70398,#70399,#70400,#70401,#70402,#70403,
#70404,#70405,#70406,#70407,#70408,#70409,#70410,#70411,#70412,#70413,#70414,
#70415,#70416,#70417,#70418,#70419,#70420,#70421,#70422,#70423,#70424,#70425,
#70426,#70427,#70428,#70429,#70430,#70431,#70432,#70433,#70434,#70435,#70436,
#70437,#70438,#70439,#70440,#70441,#70442,#70443,#70444),(#70445,#70446,
#70447,#70448,#70449,#70450,#70451,#70452,#70453,#70454,#70455,#70456,#70457,
#70458,#70459,#70460,#70461,#70462,#70463,#70464,#70465,#70466,#70467,#70468,
#70469,#70470,#70471,#70472,#70473,#70474,#70475,#70476,#70477,#70478,#70479,
#70480,#70481,#70482,#70483,#70484,#70485,#70486,#70487,#70488,#70489,#70490,
#70491,#70492,#70493,#70494,#70495,#70496,#70497,#70498,#70499,#70500,#70501,
#70502,#70503,#70504,#70505,#70506,#70507,#70508,#70509,#70510,#70511,#70512,
#70513,#70514,#70515,#70516,#70517,#70518,#70519,#70520,#70521,#70522,#70523,
#70524,#70525,#70526,#70527,#70528,#70529,#70530,#70531,#70532,#70533,#70534,
#70535,#70536,#70537,#70538,#70539,#70540,#70541,#70542,#70543,#70544,#70545,
#70546,#70547,#70548,#70549,#70550,#70551,#70552,#70553,#70554,#70555,#70556,
#70557,#70558,#70559,#70560,#70561,#70562,#70563,#70564,#70565,#70566,#70567,
#70568,#70569,#70570,#70571,#70572,#70573,#70574,#70575,#70576,#70577,#70578,
#70579,#70580,#70581,#70582,#70583,#70584,#70585,#70586,#70587,#70588,#70589,
#70590,#70591,#70592,#70593,#70594,#70595,#70596,#70597,#70598,#70599,#70600,
#70601,#70602,#70603,#70604,#70605,#70606,#70607,#70608,#70609,#70610,#70611,
#70612,#70613,#70614,#70615,#70616,#70617,#70618,#70619,#70620,#70621,#70622,
#70623,#70624,#70625,#70626,#70627,#70628,#70629,#70630,#70631)),
 .UNSPECIFIED.,.F.,.F.,.F.,(4,4),(4,1,1,1,1,1,1,1,1,1,1,1,1,1,1,1,1,1,1,
1,1,1,1,1,1,1,1,1,1,1,1,1,1,1,1,1,1,1,1,1,1,1,1,1,1,1,1,1,1,1,1,1,1,1,1,
1,1,1,1,1,1,1,1,1,1,1,1,1,1,1,1,1,1,1,1,1,1,1,1,1,1,1,1,1,1,1,1,1,1,1,1,
1,1,1,1,1,1,1,1,1,1,1,1,1,1,1,1,1,1,1,1,1,1,1,1,1,1,1,1,1,1,1,1,1,1,1,1,
1,1,1,1,1,1,1,1,1,1,1,1,1,1,1,1,1,1,1,1,1,1,1,1,1,1,1,1,1,1,1,1,1,1,1,1,
1,1,1,1,1,1,1,1,1,1,1,1,1,1,1,1,1,1,1,1,1,4),(0.,0.132097741590586),(11.6150328478182,
12.112727519453,12.6104221910878,13.1081168627226,13.6058115343574,14.1035062059922,
14.601200877627,15.0988955492618,15.5965902208966,16.0942848925314,16.5919795641662,
17.089674235801,17.5873689074358,18.0850635790706,18.5827582507054,19.0804529223402,
19.5781475939751,20.0758422656099,20.5735369372447,21.0712316088795,21.5689262805143,
22.0666209521491,22.5643156237839,23.0620102954187,23.5597049670535,24.0573996386883,
24.5550943103231,25.0527889819579,25.5504836535927,26.0481783252275,26.5458729968623,
27.0435676684971,27.5412623401319,28.0389570117667,28.5366516834015,29.0343463550363,
29.5320410266711,30.0297356983059,30.5274303699407,31.0251250415755,31.5228197132103,
32.0205143848451,32.5182090564799,33.0159037281147,33.5135983997495,34.0112930713843,
34.5089877430191,35.0066824146539,35.5043770862887,36.0020717579235,36.4997664295583,
36.9974611011931,37.4951557728279,37.9928504444627,38.4905451160975,38.9882397877323,
39.4859344593671,39.9836291310019,40.4813238026367,40.9790184742715,41.4767131459063,
41.9744078175411,42.472102489176,42.9697971608108,43.4674918324456,43.9651865040804,
44.4628811757152,44.96057584735,45.4582705189848,45.9559651906196,46.4536598622544,
46.9513545338892,47.449049205524,47.9467438771588,48.4444385487936,48.9421332204284,
49.4398278920632,49.937522563698,50.4352172353328,50.9329119069676,51.4306065786024,
51.9283012502372,52.425995921872,52.9236905935068,53.4213852651416,53.9190799367764,
54.4167746084112,54.914469280046,55.4121639516808,55.9098586233156,56.4075532949504,
56.9052479665852,57.40294263822,57.9006373098548,58.3983319814896,58.8960266531244,
59.3937213247592,59.891415996394,60.3891106680288,60.8868053396636,61.3845000112984,
61.8821946829332,62.379889354568,62.8775840262028,63.3752786978376,63.8729733694724,
64.3706680411072,64.868362712742,65.3660573843768,65.8637520560116,66.3614467276465,
66.8591413992813,67.3568360709161,67.8545307425508,68.3522254141857,68.8499200858205,
69.3476147574553,69.8453094290901,70.3430041007249,70.8406987723597,71.3383934439945,
71.8360881156293,72.3337827872641,72.8314774588989,73.3291721305337,73.8268668021685,
74.3245614738033,74.8222561454381,75.3199508170729,75.8176454887077,76.3153401603425,
76.8130348319773,77.3107295036121,77.8084241752469,78.3061188468817,78.8038135185165,
79.3015081901513,79.7992028617861,80.2968975334209,80.7945922050557,81.2922868766905,
81.7899815483253,82.2876762199601,82.7853708915949,83.2830655632297,83.7807602348645,
84.2784549064993,84.7761495781341,85.2738442497689,85.7715389214037,86.2692335930385,
86.7669282646733,87.2646229363081,87.7623176079429,88.2600122795777,88.7577069512125,
89.2554016228473,89.7530962944821,90.250790966117,90.7484856377518,91.2461803093866,
91.7438749810213,92.2415696526562,92.739264324291,93.2369589959258,93.7346536675606,
94.2323483391954,94.7300430108302,95.227737682465,95.7254323540998,96.2231270257346,
96.7208216973694,97.2185163690042,97.716211040639,98.2139057122738,98.7116003839086,
99.2092950555434,99.7069897271782,100.204684398813,100.702379070448,101.200073742083,
101.697768413717,102.195463085352,102.693157756987,103.190852428622),
 .UNSPECIFIED.);
#391=SHAPE_REPRESENTATION_RELATIONSHIP('SRR','None',#70832,#406);
#406=ADVANCED_BREP_SHAPE_REPRESENTATION('',(#481),#70756);
#466=STYLED_ITEM('',(#71054),#481);
#481=MANIFOLD_SOLID_BREP('Bolt',#26886);
#814=CYLINDRICAL_SURFACE('',#28893,0.7911);
#815=CYLINDRICAL_SURFACE('',#28895,0.7911);
#816=CYLINDRICAL_SURFACE('',#28896,0.7911);
#817=CYLINDRICAL_SURFACE('',#28897,0.7911);
#818=CYLINDRICAL_SURFACE('',#28898,0.7911);
#819=CYLINDRICAL_SURFACE('',#28899,0.7911);
#820=CYLINDRICAL_SURFACE('',#28900,0.7911);
#821=CYLINDRICAL_SURFACE('',#28901,0.7911);
#822=CYLINDRICAL_SURFACE('',#28902,0.7911);
#823=CYLINDRICAL_SURFACE('',#28903,0.7911);
#824=CYLINDRICAL_SURFACE('',#28904,0.7911);
#825=CYLINDRICAL_SURFACE('',#28905,0.7911);
#826=CYLINDRICAL_SURFACE('',#28906,0.7911);
#827=CYLINDRICAL_SURFACE('',#28907,0.7911);
#828=CYLINDRICAL_SURFACE('',#28908,0.7911);
#829=CYLINDRICAL_SURFACE('',#28910,0.6767);
#830=CYLINDRICAL_SURFACE('',#28912,0.6767);
#831=CYLINDRICAL_SURFACE('',#28913,0.6767);
#832=CYLINDRICAL_SURFACE('',#28914,0.6767);
#833=CYLINDRICAL_SURFACE('',#28915,0.6767);
#834=CYLINDRICAL_SURFACE('',#28916,0.6767);
#835=CYLINDRICAL_SURFACE('',#28917,0.6767);
#836=CYLINDRICAL_SURFACE('',#28918,0.6767);
#837=CYLINDRICAL_SURFACE('',#28919,0.6767);
#838=CYLINDRICAL_SURFACE('',#28920,0.6767);
#839=CYLINDRICAL_SURFACE('',#28921,0.6767);
#840=CYLINDRICAL_SURFACE('',#28922,0.6767);
#841=CYLINDRICAL_SURFACE('',#28923,0.6767);
#842=CYLINDRICAL_SURFACE('',#28924,0.6767);
#843=CYLINDRICAL_SURFACE('',#28943,0.6767);
#844=CYLINDRICAL_SURFACE('',#28949,0.7911);
#919=FACE_BOUND('',#5561,.T.);
#920=FACE_BOUND('',#5562,.T.);
#921=FACE_BOUND('',#5602,.T.);
#922=FACE_BOUND('',#5603,.T.);
#923=FACE_BOUND('',#5615,.T.);
#924=FACE_BOUND('',#5625,.T.);
#925=FACE_BOUND('',#5626,.T.);
#926=FACE_BOUND('',#5627,.T.);
#1483=B_SPLINE_CURVE_WITH_KNOTS('',3,(#66006,#66007,#66008,#66009,#66010,
#66011,#66012,#66013,#66014,#66015,#66016,#66017,#66018,#66019,#66020,#66021),
 .UNSPECIFIED.,.F.,.F.,(4,3,3,3,3,4),(-4.09293042013066,-3.98155737307842,
-3.48386270144362,-2.98616802980881,-2.48847335817401,-2.07498647268397),
 .UNSPECIFIED.);
#1484=B_SPLINE_CURVE_WITH_KNOTS('',3,(#66024,#66025,#66026,#66027,#66028,
#66029,#66030,#66031,#66032,#66033),.UNSPECIFIED.,.F.,.F.,(4,3,3,4),(0.,
0.497694671634796,0.995389343269607,1.12364870614303),.UNSPECIFIED.);
#1485=B_SPLINE_CURVE_WITH_KNOTS('',3,(#66038,#66039,#66040,#66041,#66042,
#66043,#66044,#66045,#66046,#66047,#66048,#66049,#66050,#66051,#66052,#66053,
#66054,#66055,#66056,#66057,#66058,#66059,#66060,#66061,#66062,#66063,#66064,
#66065,#66066,#66067,#66068,#66069,#66070,#66071,#66072,#66073,#66074,#66075,
#66076,#66077),.UNSPECIFIED.,.F.,.F.,(4,3,3,3,3,3,3,3,3,3,3,3,3,4),(-10.3761157273103,
-9.95389343269604,-9.45619876106124,-8.95850408942644,-8.46080941779164,
-7.96311474615684,-7.46542007452203,-6.96772540288723,-6.47003073125243,
-5.97233605961763,-5.47464138798282,-4.97694671634802,-4.47925204471322,
-4.09293042013066),.UNSPECIFIED.);
#1486=B_SPLINE_CURVE_WITH_KNOTS('',3,(#66078,#66079,#66080,#66081,#66082,
#66083,#66084,#66085,#66086,#66087,#66088,#66089,#66090,#66091,#66092,#66093,
#66094,#66095,#66096,#66097,#66098,#66099,#66100,#66101,#66102,#66103,#66104,
#66105,#66106,#66107,#66108,#66109,#66110,#66111,#66112,#66113,#66114,#66115,
#66116,#66117),.UNSPECIFIED.,.F.,.F.,(4,3,3,3,3,3,3,3,3,3,3,3,3,4),(1.12364870614303,
1.49308401490441,1.99077868653921,2.48847335817401,2.98616802980882,3.48386270144362,
3.98155737307842,4.47925204471322,4.97694671634802,5.47464138798283,5.97233605961763,
6.47003073125243,6.96772540288723,7.40683401332262),.UNSPECIFIED.);
#1487=B_SPLINE_CURVE_WITH_KNOTS('',3,(#66122,#66123,#66124,#66125,#66126,
#66127,#66128,#66129,#66130,#66131,#66132,#66133,#66134,#66135,#66136,#66137,
#66138,#66139,#66140,#66141,#66142,#66143,#66144,#66145,#66146,#66147,#66148,
#66149,#66150,#66151,#66152,#66153,#66154,#66155,#66156,#66157,#66158,#66159,
#66160,#66161,#66162,#66163,#66164),.UNSPECIFIED.,.F.,.F.,(4,3,3,3,3,3,
3,3,3,3,3,3,3,3,4),(-16.6593010344898,-16.4239241639485,-15.9262294923137,
-15.4285348206789,-14.9308401490441,-14.4331454774093,-13.9354508057745,
-13.4377561341397,-12.9400614625049,-12.4423667908701,-11.9446721192353,
-11.4469774476004,-10.9492827759657,-10.4515881043308,-10.3761157273103),
 .UNSPECIFIED.);
#1488=B_SPLINE_CURVE_WITH_KNOTS('',3,(#66165,#66166,#66167,#66168,#66169,
#66170,#66171,#66172,#66173,#66174,#66175,#66176,#66177,#66178,#66179,#66180,
#66181,#66182,#66183,#66184,#66185,#66186,#66187,#66188,#66189,#66190,#66191,
#66192,#66193,#66194,#66195,#66196,#66197,#66198,#66199,#66200,#66201,#66202,
#66203,#66204,#66205,#66206,#66207),.UNSPECIFIED.,.F.,.F.,(4,3,3,3,3,3,
3,3,3,3,3,3,3,3,4),(7.40683401332262,7.46542007452203,7.96311474615683,
8.46080941779163,8.95850408942644,9.45619876106124,9.95389343269604,10.4515881043308,
10.9492827759656,11.4469774476004,11.9446721192352,12.44236679087,12.9400614625048,
13.4377561341397,13.6900193205022),.UNSPECIFIED.);
#1489=B_SPLINE_CURVE_WITH_KNOTS('',3,(#66212,#66213,#66214,#66215,#66216,
#66217,#66218,#66219,#66220,#66221,#66222,#66223,#66224,#66225,#66226,#66227,
#66228,#66229,#66230,#66231,#66232,#66233,#66234,#66235,#66236,#66237,#66238,
#66239,#66240,#66241,#66242,#66243,#66244,#66245,#66246,#66247,#66248,#66249,
#66250,#66251,#66252,#66253,#66254),.UNSPECIFIED.,.F.,.F.,(4,3,3,3,3,3,
3,3,3,3,3,3,3,3,4),(-22.9424863416694,-22.8939548952009,-22.3962602235661,
-21.8985655519313,-21.4008708802965,-20.9031762086617,-20.4054815370269,
-19.9077868653921,-19.4100921937573,-18.9123975221225,-18.4147028504877,
-17.9170081788529,-17.4193135072181,-16.9216188355833,-16.6593010344898),
 .UNSPECIFIED.);
#1490=B_SPLINE_CURVE_WITH_KNOTS('',3,(#66255,#66256,#66257,#66258,#66259,
#66260,#66261,#66262,#66263,#66264,#66265,#66266,#66267,#66268,#66269,#66270,
#66271,#66272,#66273,#66274,#66275,#66276,#66277,#66278,#66279,#66280,#66281,
#66282,#66283,#66284,#66285,#66286,#66287,#66288,#66289,#66290,#66291,#66292,
#66293,#66294,#66295,#66296,#66297),.UNSPECIFIED.,.F.,.F.,(4,3,3,3,3,3,
3,3,3,3,3,3,3,3,4),(13.6900193205022,13.9354508057745,14.4331454774093,
14.9308401490441,15.4285348206789,15.9262294923137,16.4239241639485,16.9216188355833,
17.4193135072181,17.9170081788529,18.4147028504877,18.9123975221225,19.4100921937573,
19.9077868653921,19.9732046276818),.UNSPECIFIED.);
#1491=B_SPLINE_CURVE_WITH_KNOTS('',3,(#66302,#66303,#66304,#66305,#66306,
#66307,#66308,#66309,#66310,#66311,#66312,#66313,#66314,#66315,#66316,#66317,
#66318,#66319,#66320,#66321,#66322,#66323,#66324,#66325,#66326,#66327,#66328,
#66329,#66330,#66331,#66332,#66333,#66334,#66335,#66336,#66337,#66338,#66339,
#66340,#66341),.UNSPECIFIED.,.F.,.F.,(4,3,3,3,3,3,3,3,3,3,3,3,3,4),(-29.225671648849,
-28.8662909548185,-28.3685962831837,-27.8709016115489,-27.3732069399141,
-26.8755122682793,-26.3778175966445,-25.8801229250097,-25.3824282533749,
-24.8847335817401,-24.3870389101053,-23.8893442384705,-23.3916495668357,
-22.9424863416694),.UNSPECIFIED.);
#1492=B_SPLINE_CURVE_WITH_KNOTS('',3,(#66342,#66343,#66344,#66345,#66346,
#66347,#66348,#66349,#66350,#66351,#66352,#66353,#66354,#66355,#66356,#66357,
#66358,#66359,#66360,#66361,#66362,#66363,#66364,#66365,#66366,#66367,#66368,
#66369,#66370,#66371,#66372,#66373,#66374,#66375,#66376,#66377,#66378,#66379,
#66380,#66381),.UNSPECIFIED.,.F.,.F.,(4,3,3,3,3,3,3,3,3,3,3,3,3,4),(19.9732046276818,
20.4054815370269,20.9031762086617,21.4008708802965,21.8985655519313,22.3962602235661,
22.8939548952009,23.3916495668357,23.8893442384705,24.3870389101053,24.8847335817401,
25.3824282533749,25.8801229250097,26.2563899348614),.UNSPECIFIED.);
#1493=B_SPLINE_CURVE_WITH_KNOTS('',3,(#66386,#66387,#66388,#66389,#66390,
#66391,#66392,#66393,#66394,#66395,#66396,#66397,#66398,#66399,#66400,#66401,
#66402,#66403,#66404,#66405,#66406,#66407,#66408,#66409,#66410,#66411,#66412,
#66413,#66414,#66415,#66416,#66417,#66418,#66419,#66420,#66421,#66422,#66423,
#66424,#66425,#66426,#66427,#66428),.UNSPECIFIED.,.F.,.F.,(4,3,3,3,3,3,
3,3,3,3,3,3,3,3,4),(-35.5088569560286,-35.336321686071,-34.8386270144361,
-34.3409323428013,-33.8432376711666,-33.3455429995317,-32.8478483278969,
-32.3501536562621,-31.8524589846273,-31.3547643129925,-30.8570696413577,
-30.3593749697229,-29.8616802980881,-29.3639856264533,-29.225671648849),
 .UNSPECIFIED.);
#1494=B_SPLINE_CURVE_WITH_KNOTS('',3,(#66429,#66430,#66431,#66432,#66433,
#66434,#66435,#66436,#66437,#66438,#66439,#66440,#66441,#66442,#66443,#66444,
#66445,#66446,#66447,#66448,#66449,#66450,#66451,#66452,#66453,#66454,#66455,
#66456,#66457,#66458,#66459,#66460,#66461,#66462,#66463,#66464,#66465,#66466,
#66467,#66468,#66469,#66470,#66471),.UNSPECIFIED.,.F.,.F.,(4,3,3,3,3,3,
3,3,3,3,3,3,3,3,4),(26.2563899348614,26.3778175966445,26.8755122682793,
27.3732069399141,27.8709016115489,28.3685962831837,28.8662909548185,29.3639856264533,
29.8616802980881,30.3593749697229,30.8570696413577,31.3547643129925,31.8524589846273,
32.3501536562621,32.539575242041),.UNSPECIFIED.);
#1495=B_SPLINE_CURVE_WITH_KNOTS('',3,(#66476,#66477,#66478,#66479,#66480,
#66481,#66482,#66483,#66484,#66485,#66486,#66487,#66488,#66489,#66490,#66491,
#66492,#66493,#66494,#66495,#66496,#66497,#66498,#66499,#66500,#66501,#66502,
#66503,#66504,#66505,#66506,#66507,#66508,#66509,#66510,#66511,#66512,#66513,
#66514,#66515),.UNSPECIFIED.,.F.,.F.,(4,3,3,3,3,3,3,3,3,3,3,3,3,4),(-41.7920422632082,
-41.3086577456886,-40.8109630740538,-40.313268402419,-39.8155737307842,
-39.3178790591494,-38.8201843875146,-38.3224897158798,-37.824795044245,
-37.3271003726102,-36.8294057009754,-36.3317110293406,-35.8340163577058,
-35.5088569560286),.UNSPECIFIED.);
#1496=B_SPLINE_CURVE_WITH_KNOTS('',3,(#66516,#66517,#66518,#66519,#66520,
#66521,#66522,#66523,#66524,#66525,#66526,#66527,#66528,#66529,#66530,#66531,
#66532,#66533,#66534,#66535,#66536,#66537,#66538,#66539,#66540,#66541,#66542,
#66543,#66544,#66545,#66546,#66547,#66548,#66549,#66550,#66551,#66552,#66553,
#66554,#66555,#66556,#66557,#66558),.UNSPECIFIED.,.F.,.F.,(4,3,3,3,3,3,
3,3,3,3,3,3,3,3,4),(32.539575242041,32.8478483278969,33.3455429995317,33.8432376711665,
34.3409323428013,34.8386270144361,35.336321686071,35.8340163577058,36.3317110293406,
36.8294057009754,37.3271003726102,37.824795044245,38.3224897158798,38.8201843875146,
38.8227605492206),.UNSPECIFIED.);
#1497=B_SPLINE_CURVE_WITH_KNOTS('',3,(#66563,#66564,#66565,#66566,#66567,
#66568,#66569,#66570,#66571,#66572,#66573,#66574,#66575,#66576,#66577,#66578,
#66579,#66580,#66581,#66582,#66583,#66584,#66585,#66586,#66587,#66588,#66589,
#66590,#66591,#66592,#66593,#66594,#66595,#66596,#66597,#66598,#66599,#66600,
#66601,#66602,#66603,#66604,#66605),.UNSPECIFIED.,.F.,.F.,(4,3,3,3,3,3,
3,3,3,3,3,3,3,3,4),(-48.0752275703878,-47.778688476941,-47.2809938053062,
-46.7832991336714,-46.2856044620366,-45.7879097904018,-45.290215118767,
-44.7925204471322,-44.2948257754974,-43.7971311038626,-43.2994364322278,
-42.801741760593,-42.3040470889582,-41.8063524173234,-41.7920422632082),
 .UNSPECIFIED.);
#1498=B_SPLINE_CURVE_WITH_KNOTS('',3,(#66606,#66607,#66608,#66609,#66610,
#66611,#66612,#66613,#66614,#66615,#66616,#66617,#66618,#66619,#66620,#66621,
#66622,#66623,#66624,#66625,#66626,#66627,#66628,#66629,#66630,#66631,#66632,
#66633,#66634,#66635,#66636,#66637,#66638,#66639,#66640,#66641,#66642,#66643,
#66644,#66645),.UNSPECIFIED.,.F.,.F.,(4,3,3,3,3,3,3,3,3,3,3,3,3,4),(38.8227605492206,
39.3178790591494,39.8155737307842,40.313268402419,40.8109630740538,41.3086577456886,
41.8063524173234,42.3040470889582,42.801741760593,43.2994364322278,43.7971311038626,
44.2948257754974,44.7925204471322,45.1059458564002),.UNSPECIFIED.);
#1499=B_SPLINE_CURVE_WITH_KNOTS('',3,(#66650,#66651,#66652,#66653,#66654,
#66655,#66656,#66657,#66658,#66659,#66660,#66661,#66662,#66663,#66664,#66665,
#66666,#66667,#66668,#66669,#66670,#66671,#66672,#66673,#66674,#66675,#66676,
#66677,#66678,#66679,#66680,#66681,#66682,#66683,#66684,#66685,#66686,#66687,
#66688,#66689,#66690,#66691,#66692),.UNSPECIFIED.,.F.,.F.,(4,3,3,3,3,3,
3,3,3,3,3,3,3,3,4),(-54.3584128775674,-54.2487192081934,-53.7510245365586,
-53.2533298649238,-52.755635193289,-52.2579405216542,-51.7602458500194,
-51.2625511783846,-50.7648565067498,-50.267161835115,-49.7694671634802,
-49.2717724918454,-48.7740778202106,-48.2763831485758,-48.0752275703878),
 .UNSPECIFIED.);
#1500=B_SPLINE_CURVE_WITH_KNOTS('',3,(#66693,#66694,#66695,#66696,#66697,
#66698,#66699,#66700,#66701,#66702,#66703,#66704,#66705,#66706,#66707,#66708,
#66709,#66710,#66711,#66712,#66713,#66714,#66715,#66716,#66717,#66718,#66719,
#66720,#66721,#66722,#66723,#66724,#66725,#66726,#66727,#66728,#66729,#66730,
#66731,#66732,#66733,#66734,#66735),.UNSPECIFIED.,.F.,.F.,(4,3,3,3,3,3,
3,3,3,3,3,3,3,3,4),(45.1059458564002,45.290215118767,45.7879097904018,46.2856044620366,
46.7832991336714,47.2809938053062,47.778688476941,48.2763831485758,48.7740778202106,
49.2717724918454,49.7694671634802,50.267161835115,50.7648565067498,51.2625511783846,
51.3891311635797),.UNSPECIFIED.);
#1501=B_SPLINE_CURVE_WITH_KNOTS('',3,(#66740,#66741,#66742,#66743,#66744,
#66745,#66746,#66747,#66748,#66749,#66750,#66751,#66752,#66753,#66754,#66755,
#66756,#66757,#66758,#66759,#66760,#66761,#66762,#66763,#66764,#66765,#66766,
#66767,#66768,#66769,#66770,#66771,#66772,#66773,#66774,#66775,#66776,#66777,
#66778,#66779),.UNSPECIFIED.,.F.,.F.,(4,3,3,3,3,3,3,3,3,3,3,3,3,4),(-60.641598184747,
-60.2210552678111,-59.7233605961763,-59.2256659245415,-58.7279712529067,
-58.2302765812719,-57.732581909637,-57.2348872380022,-56.7371925663674,
-56.2394978947326,-55.7418032230978,-55.244108551463,-54.7464138798282,
-54.3584128775674),.UNSPECIFIED.);
#1502=B_SPLINE_CURVE_WITH_KNOTS('',3,(#66780,#66781,#66782,#66783,#66784,
#66785,#66786,#66787,#66788,#66789,#66790,#66791,#66792,#66793,#66794,#66795,
#66796,#66797,#66798,#66799,#66800,#66801,#66802,#66803,#66804,#66805,#66806,
#66807,#66808,#66809,#66810,#66811,#66812,#66813,#66814,#66815,#66816,#66817,
#66818,#66819),.UNSPECIFIED.,.F.,.F.,(4,3,3,3,3,3,3,3,3,3,3,3,3,4),(51.3891311635797,
51.7602458500194,52.2579405216542,52.755635193289,53.2533298649238,53.7510245365586,
54.2487192081934,54.7464138798282,55.244108551463,55.7418032230979,56.2394978947326,
56.7371925663674,57.2348872380022,57.6723164707593),.UNSPECIFIED.);
#1503=B_SPLINE_CURVE_WITH_KNOTS('',3,(#66824,#66825,#66826,#66827,#66828,
#66829,#66830,#66831,#66832,#66833,#66834,#66835,#66836,#66837,#66838,#66839,
#66840,#66841,#66842,#66843,#66844,#66845,#66846,#66847,#66848,#66849,#66850,
#66851,#66852,#66853,#66854,#66855,#66856,#66857,#66858,#66859,#66860,#66861,
#66862,#66863,#66864,#66865,#66866),.UNSPECIFIED.,.F.,.F.,(4,3,3,3,3,3,
3,3,3,3,3,3,3,3,4),(-66.9247834919266,-66.6910859990635,-66.1933913274287,
-65.6956966557939,-65.1980019841591,-64.7003073125243,-64.2026126408895,
-63.7049179692547,-63.2072232976199,-62.7095286259851,-62.2118339543503,
-61.7141392827155,-61.2164446110807,-60.7187499394459,-60.641598184747),
 .UNSPECIFIED.);
#1504=B_SPLINE_CURVE_WITH_KNOTS('',3,(#66867,#66868,#66869,#66870,#66871,
#66872,#66873,#66874,#66875,#66876,#66877,#66878,#66879,#66880,#66881,#66882,
#66883,#66884,#66885,#66886,#66887,#66888,#66889,#66890,#66891,#66892,#66893,
#66894,#66895,#66896,#66897,#66898,#66899,#66900,#66901,#66902,#66903,#66904,
#66905,#66906,#66907,#66908,#66909),.UNSPECIFIED.,.F.,.F.,(4,3,3,3,3,3,
3,3,3,3,3,3,3,3,4),(57.6723164707593,57.732581909637,58.2302765812718,58.7279712529066,
59.2256659245415,59.7233605961763,60.2210552678111,60.7187499394459,61.2164446110807,
61.7141392827155,62.2118339543503,62.7095286259851,63.2072232976199,63.7049179692547,
63.9555017779389),.UNSPECIFIED.);
#1505=B_SPLINE_CURVE_WITH_KNOTS('',3,(#66914,#66915,#66916,#66917,#66918,
#66919,#66920,#66921,#66922,#66923,#66924,#66925,#66926,#66927,#66928,#66929,
#66930,#66931,#66932,#66933,#66934,#66935,#66936,#66937,#66938,#66939,#66940,
#66941,#66942,#66943,#66944,#66945,#66946,#66947,#66948,#66949,#66950,#66951,
#66952,#66953,#66954,#66955,#66956),.UNSPECIFIED.,.F.,.F.,(4,3,3,3,3,3,
3,3,3,3,3,3,3,3,4),(-73.2079687991062,-73.1611167303159,-72.6634220586811,
-72.1657273870463,-71.6680327154115,-71.1703380437767,-70.6726433721419,
-70.1749487005071,-69.6772540288723,-69.1795593572375,-68.6818646856027,
-68.1841700139679,-67.6864753423331,-67.1887806706983,-66.9247834919266),
 .UNSPECIFIED.);
#1506=B_SPLINE_CURVE_WITH_KNOTS('',3,(#66957,#66958,#66959,#66960,#66961,
#66962,#66963,#66964,#66965,#66966,#66967,#66968,#66969,#66970,#66971,#66972,
#66973,#66974,#66975,#66976,#66977,#66978,#66979,#66980,#66981,#66982,#66983,
#66984,#66985,#66986,#66987,#66988,#66989,#66990,#66991,#66992,#66993,#66994,
#66995,#66996,#66997,#66998,#66999),.UNSPECIFIED.,.F.,.F.,(4,3,3,3,3,3,
3,3,3,3,3,3,3,3,4),(63.9555017779389,64.2026126408895,64.7003073125243,
65.1980019841591,65.6956966557939,66.1933913274287,66.6910859990635,67.1887806706983,
67.6864753423331,68.1841700139679,68.6818646856027,69.1795593572375,69.6772540288723,
70.1749487005071,70.2386870851185),.UNSPECIFIED.);
#1507=B_SPLINE_CURVE_WITH_KNOTS('',3,(#67004,#67005,#67006,#67007,#67008,
#67009,#67010,#67011,#67012,#67013,#67014,#67015,#67016,#67017,#67018,#67019,
#67020,#67021,#67022,#67023,#67024,#67025,#67026,#67027,#67028,#67029,#67030,
#67031,#67032,#67033,#67034,#67035,#67036,#67037,#67038,#67039,#67040,#67041,
#67042,#67043),.UNSPECIFIED.,.F.,.F.,(4,3,3,3,3,3,3,3,3,3,3,3,3,4),(-79.4911541062858,
-79.1334527899335,-78.6357581182987,-78.1380634466639,-77.6403687750291,
-77.1426741033943,-76.6449794317595,-76.1472847601247,-75.6495900884899,
-75.1518954168551,-74.6542007452203,-74.1565060735855,-73.6588114019507,
-73.2079687991062),.UNSPECIFIED.);
#1508=B_SPLINE_CURVE_WITH_KNOTS('',3,(#67044,#67045,#67046,#67047,#67048,
#67049,#67050,#67051,#67052,#67053,#67054,#67055,#67056,#67057,#67058,#67059,
#67060,#67061,#67062,#67063,#67064,#67065,#67066,#67067,#67068,#67069,#67070,
#67071,#67072,#67073,#67074,#67075,#67076,#67077,#67078,#67079,#67080,#67081,
#67082,#67083),.UNSPECIFIED.,.F.,.F.,(4,3,3,3,3,3,3,3,3,3,3,3,3,4),(70.2386870851185,
70.6726433721419,71.1703380437767,71.6680327154115,72.1657273870463,72.6634220586811,
73.1611167303159,73.6588114019507,74.1565060735855,74.6542007452203,75.1518954168551,
75.6495900884899,76.1472847601247,76.5218723922981),.UNSPECIFIED.);
#1509=B_SPLINE_CURVE_WITH_KNOTS('',3,(#67088,#67089,#67090,#67091,#67092,
#67093,#67094,#67095,#67096,#67097,#67098,#67099,#67100,#67101,#67102,#67103,
#67104,#67105,#67106,#67107,#67108,#67109,#67110,#67111,#67112,#67113,#67114,
#67115,#67116,#67117,#67118,#67119,#67120,#67121,#67122,#67123,#67124,#67125,
#67126,#67127,#67128,#67129,#67130),.UNSPECIFIED.,.F.,.F.,(4,3,3,3,3,3,
3,3,3,3,3,3,3,3,4),(-85.7743394134654,-85.603483521186,-85.1057888495512,
-84.6080941779164,-84.1103995062816,-83.6127048346468,-83.115010163012,
-82.6173154913772,-82.1196208197424,-81.6219261481075,-81.1242314764727,
-80.6265368048379,-80.1288421332031,-79.6311474615683,-79.4911541062858),
 .UNSPECIFIED.);
#1510=B_SPLINE_CURVE_WITH_KNOTS('',3,(#67131,#67132,#67133,#67134,#67135,
#67136,#67137,#67138,#67139,#67140,#67141,#67142,#67143,#67144,#67145,#67146,
#67147,#67148,#67149,#67150,#67151,#67152,#67153,#67154,#67155,#67156,#67157,
#67158,#67159,#67160,#67161,#67162,#67163,#67164,#67165,#67166,#67167,#67168,
#67169,#67170,#67171,#67172,#67173),.UNSPECIFIED.,.F.,.F.,(4,3,3,3,3,3,
3,3,3,3,3,3,3,3,4),(76.5218723922981,76.6449794317595,77.1426741033943,
77.6403687750291,78.1380634466639,78.6357581182987,79.1334527899335,79.6311474615683,
80.1288421332031,80.6265368048379,81.1242314764728,81.6219261481075,82.1196208197423,
82.6173154913771,82.8050576994777),.UNSPECIFIED.);
#1511=B_SPLINE_CURVE_WITH_KNOTS('',3,(#67180,#67181,#67182,#67183,#67184,
#67185,#67186,#67187,#67188,#67189,#67190,#67191,#67192,#67193,#67194,#67195,
#67196,#67197,#67198,#67199,#67200,#67201,#67202,#67203,#67204,#67205,#67206,
#67207,#67208,#67209,#67210,#67211,#67212,#67213,#67214,#67215,#67216),
 .UNSPECIFIED.,.F.,.F.,(4,3,3,3,3,3,3,3,3,3,3,3,4),(-91.5758195808036,-91.0781249091688,
-90.580430237534,-90.0827355658992,-89.5850408942644,-89.0873462226296,
-88.5896515509948,-88.09195687936,-87.5942622077252,-87.0965675360904,-86.5988728644556,
-86.1011781928208,-85.7743394134654),.UNSPECIFIED.);
#1512=B_SPLINE_CURVE_WITH_KNOTS('',3,(#67217,#67218,#67219,#67220,#67221,
#67222,#67223,#67224,#67225,#67226,#67227,#67228,#67229,#67230,#67231,#67232,
#67233,#67234,#67235,#67236,#67237,#67238,#67239,#67240,#67241,#67242,#67243,
#67244,#67245,#67246,#67247,#67248,#67249,#67250,#67251,#67252,#67253,#67254,
#67255,#67256),.UNSPECIFIED.,.F.,.F.,(4,3,3,3,3,3,3,3,3,3,3,3,3,4),(82.8050576994777,
83.1150101630119,83.6127048346467,84.1103995062816,84.6080941779164,85.1057888495512,
85.603483521186,86.1011781928208,86.5988728644556,87.0965675360904,87.5942622077252,
88.09195687936,88.5896515509948,89.0882430066573),.UNSPECIFIED.);
#1513=B_SPLINE_CURVE_WITH_KNOTS('',3,(#67262,#67263,#67264,#67265,#67266,
#67267,#67268,#67269,#67270,#67271,#67272),.UNSPECIFIED.,.F.,.F.,(4,1,1,
1,1,1,1,1,4),(97.3893722612836,97.716211040639,98.2139057122738,98.7116003839086,
99.2092950555434,99.7069897271782,100.204684398813,100.702379070448,101.115865955938),
 .UNSPECIFIED.);
#1514=B_SPLINE_CURVE_WITH_KNOTS('',3,(#67275,#67276,#67277,#67278,#67279,
#67280,#67281,#67282),.UNSPECIFIED.,.F.,.F.,(4,1,1,1,1,4),(97.3893722612836,
97.8861701488906,98.3838648205254,98.8815594921602,99.379254163795,99.8769488354298),
 .UNSPECIFIED.);
#1515=B_SPLINE_CURVE_WITH_KNOTS('',3,(#67287,#67288,#67289,#67290,#67291,
#67292,#67293,#67294,#67295,#67296,#67297,#67298,#67299,#67300,#67301,#67302,
#67303),.UNSPECIFIED.,.F.,.F.,(4,1,1,1,1,1,1,1,1,1,1,1,1,1,4),(91.106186954104,
91.2461803093866,91.7438749810213,92.2415696526562,92.739264324291,93.2369589959258,
93.7346536675606,94.2323483391954,94.7300430108302,95.227737682465,95.7254323540998,
96.2231270257346,96.7208216973694,97.2185163690042,97.3893722612836),
 .UNSPECIFIED.);
#1516=B_SPLINE_CURVE_WITH_KNOTS('',3,(#67304,#67305,#67306,#67307,#67308,
#67309,#67310,#67311,#67312,#67313,#67314,#67315,#67316,#67317,#67318,#67319,
#67320),.UNSPECIFIED.,.F.,.F.,(4,1,1,1,1,1,1,1,1,1,1,1,1,1,4),(91.106186954104,
91.4161394176381,91.9138340892729,92.4115287609077,92.9092234325425,93.4069181041774,
93.9046127758121,94.4023074474469,94.9000021190817,95.3976967907166,95.8953914623514,
96.3930861339862,96.890780805621,97.3884754772558,97.3893722612836),
 .UNSPECIFIED.);
#1517=B_SPLINE_CURVE_WITH_KNOTS('',3,(#67325,#67326,#67327,#67328,#67329,
#67330,#67331,#67332,#67333,#67334,#67335,#67336,#67337,#67338,#67339,#67340),
 .UNSPECIFIED.,.F.,.F.,(4,1,1,1,1,1,1,1,1,1,1,1,1,4),(84.8230016469244,
85.2738442497689,85.7715389214037,86.2692335930385,86.7669282646733,87.2646229363081,
87.7623176079429,88.2600122795777,88.7577069512125,89.2554016228473,89.7530962944821,
90.250790966117,90.7484856377518,91.106186954104),.UNSPECIFIED.);
#1518=B_SPLINE_CURVE_WITH_KNOTS('',3,(#67341,#67342,#67343,#67344,#67345,
#67346,#67347,#67348,#67349,#67350,#67351,#67352,#67353,#67354,#67355,#67356,
#67357),.UNSPECIFIED.,.F.,.F.,(4,1,1,1,1,1,1,1,1,1,1,1,1,1,4),(84.8230016469244,
84.9461086863857,85.4438033580205,85.9414980296553,86.4391927012901,86.9368873729249,
87.4345820445597,87.9322767161945,88.4299713878293,88.9276660594641,89.4253607310989,
89.9230554027337,90.4207500743685,90.9184447460033,91.106186954104),
 .UNSPECIFIED.);
#1519=B_SPLINE_CURVE_WITH_KNOTS('',3,(#67362,#67363,#67364,#67365,#67366,
#67367,#67368,#67369,#67370,#67371,#67372,#67373,#67374,#67375,#67376,#67377,
#67378),.UNSPECIFIED.,.F.,.F.,(4,1,1,1,1,1,1,1,1,1,1,1,1,1,4),(78.5398163397448,
78.8038135185165,79.3015081901513,79.7992028617861,80.2968975334209,80.7945922050557,
81.2922868766905,81.7899815483253,82.2876762199601,82.7853708915949,83.2830655632297,
83.7807602348645,84.2784549064993,84.7761495781341,84.8230016469244),
 .UNSPECIFIED.);
#1520=B_SPLINE_CURVE_WITH_KNOTS('',3,(#67379,#67380,#67381,#67382,#67383,
#67384,#67385,#67386,#67387,#67388,#67389,#67390,#67391,#67392,#67393,#67394),
 .UNSPECIFIED.,.F.,.F.,(4,1,1,1,1,1,1,1,1,1,1,1,1,4),(78.5398163397448,
78.9737726267681,79.4714672984029,79.9691619700377,80.4668566416725,80.9645513133073,
81.4622459849421,81.9599406565769,82.4576353282117,82.9553299998465,83.4530246714813,
83.9507193431161,84.4484140147509,84.8230016469244),.UNSPECIFIED.);
#1521=B_SPLINE_CURVE_WITH_KNOTS('',3,(#67399,#67400,#67401,#67402,#67403,
#67404,#67405,#67406,#67407,#67408,#67409,#67410,#67411,#67412,#67413,#67414,
#67415),.UNSPECIFIED.,.F.,.F.,(4,1,1,1,1,1,1,1,1,1,1,1,1,1,4),(72.2566310325652,
72.3337827872641,72.8314774588989,73.3291721305337,73.8268668021685,74.3245614738033,
74.8222561454381,75.3199508170729,75.8176454887077,76.3153401603425,76.8130348319773,
77.3107295036121,77.8084241752469,78.3061188468817,78.5398163397448),
 .UNSPECIFIED.);
#1522=B_SPLINE_CURVE_WITH_KNOTS('',3,(#67416,#67417,#67418,#67419,#67420,
#67421,#67422,#67423,#67424,#67425,#67426,#67427,#67428,#67429,#67430,#67431,
#67432),.UNSPECIFIED.,.F.,.F.,(4,1,1,1,1,1,1,1,1,1,1,1,1,1,4),(72.2566310325652,
72.5037418955157,73.0014365671505,73.4991312387853,73.9968259104201,74.4945205820549,
74.9922152536897,75.4899099253245,75.9876045969593,76.4852992685941,76.9829939402289,
77.4806886118637,77.9783832834985,78.4760779551333,78.5398163397448),
 .UNSPECIFIED.);
#1523=B_SPLINE_CURVE_WITH_KNOTS('',3,(#67437,#67438,#67439,#67440,#67441,
#67442,#67443,#67444,#67445,#67446,#67447,#67448,#67449,#67450,#67451,#67452),
 .UNSPECIFIED.,.F.,.F.,(4,1,1,1,1,1,1,1,1,1,1,1,1,4),(65.9734457253856,
66.3614467276465,66.8591413992813,67.3568360709161,67.8545307425508,68.3522254141857,
68.8499200858205,69.3476147574553,69.8453094290901,70.3430041007249,70.8406987723597,
71.3383934439945,71.8360881156293,72.2566310325652),.UNSPECIFIED.);
#1524=B_SPLINE_CURVE_WITH_KNOTS('',3,(#67453,#67454,#67455,#67456,#67457,
#67458,#67459,#67460,#67461,#67462,#67463,#67464,#67465,#67466,#67467,#67468,
#67469),.UNSPECIFIED.,.F.,.F.,(4,1,1,1,1,1,1,1,1,1,1,1,1,1,4),(65.9734457253856,
66.0337111642632,66.531405835898,67.0291005075328,67.5267951791676,68.0244898508024,
68.5221845224372,69.019879194072,69.5175738657069,70.0152685373416,70.5129632089764,
71.0106578806112,71.5083525522461,72.0060472238809,72.2566310325652),
 .UNSPECIFIED.);
#1525=B_SPLINE_CURVE_WITH_KNOTS('',3,(#67474,#67475,#67476,#67477,#67478,
#67479,#67480,#67481,#67482,#67483,#67484,#67485,#67486,#67487,#67488,#67489,
#67490),.UNSPECIFIED.,.F.,.F.,(4,1,1,1,1,1,1,1,1,1,1,1,1,1,4),(59.690260418206,
59.891415996394,60.3891106680288,60.8868053396636,61.3845000112984,61.8821946829332,
62.379889354568,62.8775840262028,63.3752786978376,63.8729733694724,64.3706680411072,
64.868362712742,65.3660573843768,65.8637520560116,65.9734457253856),
 .UNSPECIFIED.);
#1526=B_SPLINE_CURVE_WITH_KNOTS('',3,(#67491,#67492,#67493,#67494,#67495,
#67496,#67497,#67498,#67499,#67500,#67501,#67502,#67503,#67504,#67505,#67506),
 .UNSPECIFIED.,.F.,.F.,(4,1,1,1,1,1,1,1,1,1,1,1,1,4),(59.690260418206,60.0613751046456,
60.5590697762804,61.0567644479152,61.55445911955,62.0521537911848,62.5498484628196,
63.0475431344544,63.5452378060892,64.042932477724,64.5406271493588,65.0383218209936,
65.5360164926284,65.9734457253856),.UNSPECIFIED.);
#1527=B_SPLINE_CURVE_WITH_KNOTS('',3,(#67511,#67512,#67513,#67514,#67515,
#67516,#67517,#67518,#67519,#67520,#67521,#67522,#67523,#67524,#67525,#67526,
#67527),.UNSPECIFIED.,.F.,.F.,(4,1,1,1,1,1,1,1,1,1,1,1,1,1,4),(53.4070751110264,
53.4213852651416,53.9190799367764,54.4167746084112,54.914469280046,55.4121639516808,
55.9098586233156,56.4075532949504,56.9052479665852,57.40294263822,57.9006373098548,
58.3983319814896,58.8960266531244,59.3937213247592,59.690260418206),
 .UNSPECIFIED.);
#1528=B_SPLINE_CURVE_WITH_KNOTS('',3,(#67528,#67529,#67530,#67531,#67532,
#67533,#67534,#67535,#67536,#67537,#67538,#67539,#67540,#67541,#67542,#67543,
#67544),.UNSPECIFIED.,.F.,.F.,(4,1,1,1,1,1,1,1,1,1,1,1,1,1,4),(53.4070751110264,
53.5913443733932,54.089039045028,54.5867337166628,55.0844283882976,55.5821230599324,
56.0798177315672,56.577512403202,57.0752070748368,57.5729017464716,58.0705964181064,
58.5682910897412,59.065985761376,59.5636804330108,59.690260418206),
 .UNSPECIFIED.);
#1529=B_SPLINE_CURVE_WITH_KNOTS('',3,(#67549,#67550,#67551,#67552,#67553,
#67554,#67555,#67556,#67557,#67558,#67559,#67560,#67561,#67562,#67563,#67564),
 .UNSPECIFIED.,.F.,.F.,(4,1,1,1,1,1,1,1,1,1,1,1,1,4),(47.1238898038468,
47.449049205524,47.9467438771588,48.4444385487936,48.9421332204284,49.4398278920632,
49.937522563698,50.4352172353328,50.9329119069676,51.4306065786024,51.9283012502372,
52.425995921872,52.9236905935068,53.4070751110264),.UNSPECIFIED.);
#1530=B_SPLINE_CURVE_WITH_KNOTS('',3,(#67565,#67566,#67567,#67568,#67569,
#67570,#67571,#67572,#67573,#67574,#67575,#67576,#67577,#67578,#67579,#67580),
 .UNSPECIFIED.,.F.,.F.,(4,1,1,1,1,1,1,1,1,1,1,1,1,4),(47.1238898038468,
47.6190083137756,48.1167029854104,48.6143976570452,49.11209232868,49.6097870003148,
50.1074816719496,50.6051763435844,51.1028710152192,51.600565686854,52.0982603584888,
52.5959550301236,53.0936497017584,53.4070751110264),.UNSPECIFIED.);
#1531=B_SPLINE_CURVE_WITH_KNOTS('',3,(#67585,#67586,#67587,#67588,#67589,
#67590,#67591,#67592,#67593,#67594,#67595,#67596,#67597,#67598,#67599,#67600,
#67601),.UNSPECIFIED.,.F.,.F.,(4,1,1,1,1,1,1,1,1,1,1,1,1,1,4),(40.8407044966673,
40.9790184742715,41.4767131459063,41.9744078175411,42.472102489176,42.9697971608108,
43.4674918324456,43.9651865040804,44.4628811757152,44.96057584735,45.4582705189848,
45.9559651906196,46.4536598622544,46.9513545338892,47.1238898038468),
 .UNSPECIFIED.);
#1532=B_SPLINE_CURVE_WITH_KNOTS('',3,(#67602,#67603,#67604,#67605,#67606,
#67607,#67608,#67609,#67610,#67611,#67612,#67613,#67614,#67615,#67616,#67617,
#67618),.UNSPECIFIED.,.F.,.F.,(4,1,1,1,1,1,1,1,1,1,1,1,1,1,4),(40.8407044966672,
41.1489775825231,41.6466722541579,42.1443669257927,42.6420615974275,43.1397562690623,
43.6374509406971,44.1351456123319,44.6328402839667,45.1305349556015,45.6282296272363,
46.1259242988711,46.6236189705059,47.1213136421407,47.1238898038468),
 .UNSPECIFIED.);
#1533=B_SPLINE_CURVE_WITH_KNOTS('',3,(#67623,#67624,#67625,#67626,#67627,
#67628,#67629,#67630,#67631,#67632,#67633,#67634,#67635,#67636,#67637,#67638),
 .UNSPECIFIED.,.F.,.F.,(4,1,1,1,1,1,1,1,1,1,1,1,1,4),(34.5575191894877,
35.0066824146539,35.5043770862887,36.0020717579235,36.4997664295583,36.9974611011931,
37.4951557728279,37.9928504444627,38.4905451160975,38.9882397877323,39.4859344593671,
39.9836291310019,40.4813238026367,40.8407044966673),.UNSPECIFIED.);
#1534=B_SPLINE_CURVE_WITH_KNOTS('',3,(#67639,#67640,#67641,#67642,#67643,
#67644,#67645,#67646,#67647,#67648,#67649,#67650,#67651,#67652,#67653,#67654,
#67655),.UNSPECIFIED.,.F.,.F.,(4,1,1,1,1,1,1,1,1,1,1,1,1,1,4),(34.5575191894876,
34.6789468512707,35.1766415229055,35.6743361945403,36.1720308661751,36.6697255378099,
37.1674202094447,37.6651148810795,38.1628095527143,38.6605042243491,39.1581988959839,
39.6558935676187,40.1535882392535,40.6512829108883,40.8407044966672),
 .UNSPECIFIED.);
#1535=B_SPLINE_CURVE_WITH_KNOTS('',3,(#67660,#67661,#67662,#67663,#67664,
#67665,#67666,#67667,#67668,#67669,#67670,#67671,#67672,#67673,#67674,#67675,
#67676),.UNSPECIFIED.,.F.,.F.,(4,1,1,1,1,1,1,1,1,1,1,1,1,1,4),(28.2743338823081,
28.5366516834015,29.0343463550363,29.5320410266711,30.0297356983059,30.5274303699407,
31.0251250415755,31.5228197132103,32.0205143848451,32.5182090564799,33.0159037281147,
33.5135983997495,34.0112930713843,34.5089877430191,34.5575191894877),
 .UNSPECIFIED.);
#1536=B_SPLINE_CURVE_WITH_KNOTS('',3,(#67677,#67678,#67679,#67680,#67681,
#67682,#67683,#67684,#67685,#67686,#67687,#67688,#67689,#67690,#67691,#67692),
 .UNSPECIFIED.,.F.,.F.,(4,1,1,1,1,1,1,1,1,1,1,1,1,4),(28.2743338823081,
28.7066107916531,29.2043054632879,29.7020001349227,30.1996948065575,30.6973894781923,
31.1950841498271,31.6927788214619,32.1904734930967,32.6881681647315,33.1858628363663,
33.6835575080011,34.1812521796359,34.5575191894876),.UNSPECIFIED.);
#1537=B_SPLINE_CURVE_WITH_KNOTS('',3,(#67697,#67698,#67699,#67700,#67701,
#67702,#67703,#67704,#67705,#67706,#67707,#67708,#67709,#67710,#67711,#67712,
#67713),.UNSPECIFIED.,.F.,.F.,(4,1,1,1,1,1,1,1,1,1,1,1,1,1,4),(21.9911485751285,
22.0666209521491,22.5643156237839,23.0620102954187,23.5597049670535,24.0573996386883,
24.5550943103231,25.0527889819579,25.5504836535927,26.0481783252275,26.5458729968623,
27.0435676684971,27.5412623401319,28.0389570117667,28.2743338823081),
 .UNSPECIFIED.);
#1538=B_SPLINE_CURVE_WITH_KNOTS('',3,(#67714,#67715,#67716,#67717,#67718,
#67719,#67720,#67721,#67722,#67723,#67724,#67725,#67726,#67727,#67728,#67729,
#67730),.UNSPECIFIED.,.F.,.F.,(4,1,1,1,1,1,1,1,1,1,1,1,1,1,4),(21.9911485751285,
22.2365800604006,22.7342747320354,23.2319694036702,23.7296640753051,24.2273587469399,
24.7250534185747,25.2227480902095,25.7204427618443,26.2181374334791,26.7158321051139,
27.2135267767487,27.7112214483835,28.2089161200183,28.2743338823081),
 .UNSPECIFIED.);
#1539=B_SPLINE_CURVE_WITH_KNOTS('',3,(#67735,#67736,#67737,#67738,#67739,
#67740,#67741,#67742,#67743,#67744,#67745,#67746,#67747,#67748,#67749,#67750),
 .UNSPECIFIED.,.F.,.F.,(4,1,1,1,1,1,1,1,1,1,1,1,1,4),(15.7079632679489,
16.0942848925314,16.5919795641662,17.089674235801,17.5873689074358,18.0850635790706,
18.5827582507054,19.0804529223402,19.5781475939751,20.0758422656099,20.5735369372447,
21.0712316088795,21.5689262805143,21.9911485751285),.UNSPECIFIED.);
#1540=B_SPLINE_CURVE_WITH_KNOTS('',3,(#67751,#67752,#67753,#67754,#67755,
#67756,#67757,#67758,#67759,#67760,#67761,#67762,#67763,#67764,#67765,#67766,
#67767),.UNSPECIFIED.,.F.,.F.,(4,1,1,1,1,1,1,1,1,1,1,1,1,1,4),(15.7079632679489,
15.7665493291482,16.264244000783,16.7619386724178,17.2596333440526,17.7573280156874,
18.2550226873222,18.752717358957,19.2504120305918,19.7481067022266,20.2458013738614,
20.7434960454962,21.241190717131,21.7388853887658,21.9911485751285),
 .UNSPECIFIED.);
#1541=B_SPLINE_CURVE_WITH_KNOTS('',2,(#67776,#67777,#67778),
 .UNSPECIFIED.,.F.,.F.,(3,3),(0.,1.),.UNSPECIFIED.);
#1542=B_SPLINE_CURVE_WITH_KNOTS('',2,(#67782,#67783,#67784),
 .UNSPECIFIED.,.F.,.F.,(3,3),(0.,1.),.UNSPECIFIED.);
#1543=B_SPLINE_CURVE_WITH_KNOTS('',2,(#67793,#67794,#67795),
 .UNSPECIFIED.,.F.,.F.,(3,3),(0.,1.),.UNSPECIFIED.);
#1544=B_SPLINE_CURVE_WITH_KNOTS('',2,(#67798,#67799,#67800),
 .UNSPECIFIED.,.F.,.F.,(3,3),(0.,1.),.UNSPECIFIED.);
#1545=B_SPLINE_CURVE_WITH_KNOTS('',2,(#67808,#67809,#67810),
 .UNSPECIFIED.,.F.,.F.,(3,3),(0.,1.),.UNSPECIFIED.);
#1546=B_SPLINE_CURVE_WITH_KNOTS('',2,(#67813,#67814,#67815),
 .UNSPECIFIED.,.F.,.F.,(3,3),(0.,1.),.UNSPECIFIED.);
#1547=B_SPLINE_CURVE_WITH_KNOTS('',2,(#67823,#67824,#67825),
 .UNSPECIFIED.,.F.,.F.,(3,3),(0.,1.),.UNSPECIFIED.);
#1548=B_SPLINE_CURVE_WITH_KNOTS('',2,(#67828,#67829,#67830),
 .UNSPECIFIED.,.F.,.F.,(3,3),(0.,1.),.UNSPECIFIED.);
#1549=B_SPLINE_CURVE_WITH_KNOTS('',2,(#67838,#67839,#67840),
 .UNSPECIFIED.,.F.,.F.,(3,3),(0.,1.),.UNSPECIFIED.);
#1550=B_SPLINE_CURVE_WITH_KNOTS('',2,(#67843,#67844,#67845),
 .UNSPECIFIED.,.F.,.F.,(3,3),(0.,1.),.UNSPECIFIED.);
#1551=B_SPLINE_CURVE_WITH_KNOTS('',2,(#67853,#67854,#67855),
 .UNSPECIFIED.,.F.,.F.,(3,3),(0.,1.),.UNSPECIFIED.);
#1552=B_SPLINE_CURVE_WITH_KNOTS('',2,(#67858,#67859,#67860),
 .UNSPECIFIED.,.F.,.F.,(3,3),(0.,1.),.UNSPECIFIED.);
#1553=B_SPLINE_CURVE_WITH_KNOTS('',2,(#67868,#67869,#67870),
 .UNSPECIFIED.,.F.,.F.,(3,3),(0.,1.),.UNSPECIFIED.);
#1554=B_SPLINE_CURVE_WITH_KNOTS('',2,(#67873,#67874,#67875),
 .UNSPECIFIED.,.F.,.F.,(3,3),(0.,1.),.UNSPECIFIED.);
#1555=B_SPLINE_CURVE_WITH_KNOTS('',2,(#67882,#67883,#67884),
 .UNSPECIFIED.,.F.,.F.,(3,3),(0.,1.),.UNSPECIFIED.);
#1556=B_SPLINE_CURVE_WITH_KNOTS('',2,(#67885,#67886,#67887),
 .UNSPECIFIED.,.F.,.F.,(3,3),(0.,1.),.UNSPECIFIED.);
#1557=B_SPLINE_CURVE_WITH_KNOTS('',2,(#67896,#67897,#67898),
 .UNSPECIFIED.,.F.,.F.,(3,3),(0.,1.),.UNSPECIFIED.);
#1558=B_SPLINE_CURVE_WITH_KNOTS('',2,(#67902,#67903,#67904),
 .UNSPECIFIED.,.F.,.F.,(3,3),(0.,1.),.UNSPECIFIED.);
#1559=B_SPLINE_CURVE_WITH_KNOTS('',2,(#67913,#67914,#67915),
 .UNSPECIFIED.,.F.,.F.,(3,3),(0.,1.),.UNSPECIFIED.);
#1560=B_SPLINE_CURVE_WITH_KNOTS('',2,(#67918,#67919,#67920),
 .UNSPECIFIED.,.F.,.F.,(3,3),(0.,1.),.UNSPECIFIED.);
#1561=B_SPLINE_CURVE_WITH_KNOTS('',2,(#67928,#67929,#67930),
 .UNSPECIFIED.,.F.,.F.,(3,3),(0.,1.),.UNSPECIFIED.);
#1562=B_SPLINE_CURVE_WITH_KNOTS('',2,(#67933,#67934,#67935),
 .UNSPECIFIED.,.F.,.F.,(3,3),(0.,1.),.UNSPECIFIED.);
#1563=B_SPLINE_CURVE_WITH_KNOTS('',2,(#67943,#67944,#67945),
 .UNSPECIFIED.,.F.,.F.,(3,3),(0.,1.),.UNSPECIFIED.);
#1564=B_SPLINE_CURVE_WITH_KNOTS('',2,(#67948,#67949,#67950),
 .UNSPECIFIED.,.F.,.F.,(3,3),(0.,1.),.UNSPECIFIED.);
#1565=B_SPLINE_CURVE_WITH_KNOTS('',2,(#67958,#67959,#67960),
 .UNSPECIFIED.,.F.,.F.,(3,3),(0.,1.),.UNSPECIFIED.);
#1566=B_SPLINE_CURVE_WITH_KNOTS('',2,(#67963,#67964,#67965),
 .UNSPECIFIED.,.F.,.F.,(3,3),(0.,1.),.UNSPECIFIED.);
#1567=B_SPLINE_CURVE_WITH_KNOTS('',2,(#67973,#67974,#67975),
 .UNSPECIFIED.,.F.,.F.,(3,3),(0.,1.),.UNSPECIFIED.);
#1568=B_SPLINE_CURVE_WITH_KNOTS('',2,(#67978,#67979,#67980),
 .UNSPECIFIED.,.F.,.F.,(3,3),(0.,1.),.UNSPECIFIED.);
#1569=B_SPLINE_CURVE_WITH_KNOTS('',2,(#67988,#67989,#67990),
 .UNSPECIFIED.,.F.,.F.,(3,3),(0.,1.),.UNSPECIFIED.);
#1570=B_SPLINE_CURVE_WITH_KNOTS('',2,(#67993,#67994,#67995),
 .UNSPECIFIED.,.F.,.F.,(3,3),(0.,1.),.UNSPECIFIED.);
#1571=B_SPLINE_CURVE_WITH_KNOTS('',2,(#68003,#68004,#68005),
 .UNSPECIFIED.,.F.,.F.,(3,3),(0.,1.),.UNSPECIFIED.);
#1572=B_SPLINE_CURVE_WITH_KNOTS('',2,(#68008,#68009,#68010),
 .UNSPECIFIED.,.F.,.F.,(3,3),(0.,1.),.UNSPECIFIED.);
#1573=B_SPLINE_CURVE_WITH_KNOTS('',2,(#68017,#68018,#68019),
 .UNSPECIFIED.,.F.,.F.,(3,3),(0.,1.),.UNSPECIFIED.);
#1574=B_SPLINE_CURVE_WITH_KNOTS('',2,(#68020,#68021,#68022),
 .UNSPECIFIED.,.F.,.F.,(3,3),(0.,1.),.UNSPECIFIED.);
#1575=B_SPLINE_CURVE_WITH_KNOTS('',2,(#68031,#68032,#68033),
 .UNSPECIFIED.,.F.,.F.,(3,3),(0.,1.),.UNSPECIFIED.);
#1576=B_SPLINE_CURVE_WITH_KNOTS('',2,(#68037,#68038,#68039),
 .UNSPECIFIED.,.F.,.F.,(3,3),(0.,1.),.UNSPECIFIED.);
#1577=B_SPLINE_CURVE_WITH_KNOTS('',2,(#68048,#68049,#68050),
 .UNSPECIFIED.,.F.,.F.,(3,3),(0.,1.),.UNSPECIFIED.);
#1578=B_SPLINE_CURVE_WITH_KNOTS('',2,(#68053,#68054,#68055),
 .UNSPECIFIED.,.F.,.F.,(3,3),(0.,1.),.UNSPECIFIED.);
#1579=B_SPLINE_CURVE_WITH_KNOTS('',2,(#68063,#68064,#68065),
 .UNSPECIFIED.,.F.,.F.,(3,3),(0.,1.),.UNSPECIFIED.);
#1580=B_SPLINE_CURVE_WITH_KNOTS('',2,(#68068,#68069,#68070),
 .UNSPECIFIED.,.F.,.F.,(3,3),(0.,1.),.UNSPECIFIED.);
#1581=B_SPLINE_CURVE_WITH_KNOTS('',2,(#68078,#68079,#68080),
 .UNSPECIFIED.,.F.,.F.,(3,3),(0.,1.),.UNSPECIFIED.);
#1582=B_SPLINE_CURVE_WITH_KNOTS('',2,(#68083,#68084,#68085),
 .UNSPECIFIED.,.F.,.F.,(3,3),(0.,1.),.UNSPECIFIED.);
#1583=B_SPLINE_CURVE_WITH_KNOTS('',2,(#68093,#68094,#68095),
 .UNSPECIFIED.,.F.,.F.,(3,3),(0.,1.),.UNSPECIFIED.);
#1584=B_SPLINE_CURVE_WITH_KNOTS('',2,(#68098,#68099,#68100),
 .UNSPECIFIED.,.F.,.F.,(3,3),(0.,1.),.UNSPECIFIED.);
#1585=B_SPLINE_CURVE_WITH_KNOTS('',2,(#68108,#68109,#68110),
 .UNSPECIFIED.,.F.,.F.,(3,3),(0.,1.),.UNSPECIFIED.);
#1586=B_SPLINE_CURVE_WITH_KNOTS('',2,(#68113,#68114,#68115),
 .UNSPECIFIED.,.F.,.F.,(3,3),(0.,1.),.UNSPECIFIED.);
#1587=B_SPLINE_CURVE_WITH_KNOTS('',2,(#68123,#68124,#68125),
 .UNSPECIFIED.,.F.,.F.,(3,3),(0.,1.),.UNSPECIFIED.);
#1588=B_SPLINE_CURVE_WITH_KNOTS('',2,(#68128,#68129,#68130),
 .UNSPECIFIED.,.F.,.F.,(3,3),(0.,1.),.UNSPECIFIED.);
#1589=B_SPLINE_CURVE_WITH_KNOTS('',2,(#68138,#68139,#68140),
 .UNSPECIFIED.,.F.,.F.,(3,3),(0.,1.),.UNSPECIFIED.);
#1590=B_SPLINE_CURVE_WITH_KNOTS('',2,(#68143,#68144,#68145),
 .UNSPECIFIED.,.F.,.F.,(3,3),(0.,1.),.UNSPECIFIED.);
#1591=B_SPLINE_CURVE_WITH_KNOTS('',2,(#68153,#68154,#68155),
 .UNSPECIFIED.,.F.,.F.,(3,3),(0.,1.),.UNSPECIFIED.);
#1592=B_SPLINE_CURVE_WITH_KNOTS('',2,(#68158,#68159,#68160),
 .UNSPECIFIED.,.F.,.F.,(3,3),(0.,1.),.UNSPECIFIED.);
#1593=B_SPLINE_CURVE_WITH_KNOTS('',2,(#68168,#68169,#68170),
 .UNSPECIFIED.,.F.,.F.,(3,3),(0.,1.),.UNSPECIFIED.);
#1594=B_SPLINE_CURVE_WITH_KNOTS('',2,(#68173,#68174,#68175),
 .UNSPECIFIED.,.F.,.F.,(3,3),(0.,1.),.UNSPECIFIED.);
#1595=B_SPLINE_CURVE_WITH_KNOTS('',2,(#68183,#68184,#68185),
 .UNSPECIFIED.,.F.,.F.,(3,3),(0.,1.),.UNSPECIFIED.);
#1596=B_SPLINE_CURVE_WITH_KNOTS('',2,(#68188,#68189,#68190),
 .UNSPECIFIED.,.F.,.F.,(3,3),(0.,1.),.UNSPECIFIED.);
#1597=B_SPLINE_CURVE_WITH_KNOTS('',2,(#68198,#68199,#68200),
 .UNSPECIFIED.,.F.,.F.,(3,3),(0.,1.),.UNSPECIFIED.);
#1598=B_SPLINE_CURVE_WITH_KNOTS('',2,(#68203,#68204,#68205),
 .UNSPECIFIED.,.F.,.F.,(3,3),(0.,1.),.UNSPECIFIED.);
#1599=B_SPLINE_CURVE_WITH_KNOTS('',2,(#68213,#68214,#68215),
 .UNSPECIFIED.,.F.,.F.,(3,3),(0.,1.),.UNSPECIFIED.);
#1600=B_SPLINE_CURVE_WITH_KNOTS('',2,(#68218,#68219,#68220),
 .UNSPECIFIED.,.F.,.F.,(3,3),(0.,1.),.UNSPECIFIED.);
#1601=B_SPLINE_CURVE_WITH_KNOTS('',2,(#68228,#68229,#68230),
 .UNSPECIFIED.,.F.,.F.,(3,3),(0.,1.),.UNSPECIFIED.);
#1602=B_SPLINE_CURVE_WITH_KNOTS('',2,(#68233,#68234,#68235),
 .UNSPECIFIED.,.F.,.F.,(3,3),(0.,1.),.UNSPECIFIED.);
#1603=B_SPLINE_CURVE_WITH_KNOTS('',2,(#68243,#68244,#68245),
 .UNSPECIFIED.,.F.,.F.,(3,3),(0.,1.),.UNSPECIFIED.);
#1604=B_SPLINE_CURVE_WITH_KNOTS('',2,(#68248,#68249,#68250),
 .UNSPECIFIED.,.F.,.F.,(3,3),(0.,1.),.UNSPECIFIED.);
#1605=B_SPLINE_CURVE_WITH_KNOTS('',2,(#68257,#68258,#68259),
 .UNSPECIFIED.,.F.,.F.,(3,3),(0.,1.),.UNSPECIFIED.);
#1606=B_SPLINE_CURVE_WITH_KNOTS('',2,(#68260,#68261,#68262),
 .UNSPECIFIED.,.F.,.F.,(3,3),(0.,1.),.UNSPECIFIED.);
#1607=B_SPLINE_CURVE_WITH_KNOTS('',2,(#68297,#68298,#68299),
 .UNSPECIFIED.,.F.,.F.,(3,3),(0.,1.),.UNSPECIFIED.);
#1608=B_SPLINE_CURVE_WITH_KNOTS('',2,(#68303,#68304,#68305),
 .UNSPECIFIED.,.F.,.F.,(3,3),(0.,1.),.UNSPECIFIED.);
#1609=B_SPLINE_CURVE_WITH_KNOTS('',2,(#68314,#68315,#68316),
 .UNSPECIFIED.,.F.,.F.,(3,3),(0.,1.),.UNSPECIFIED.);
#1610=B_SPLINE_CURVE_WITH_KNOTS('',2,(#68319,#68320,#68321),
 .UNSPECIFIED.,.F.,.F.,(3,3),(0.,1.),.UNSPECIFIED.);
#1611=B_SPLINE_CURVE_WITH_KNOTS('',2,(#68329,#68330,#68331),
 .UNSPECIFIED.,.F.,.F.,(3,3),(0.,1.),.UNSPECIFIED.);
#1612=B_SPLINE_CURVE_WITH_KNOTS('',2,(#68334,#68335,#68336),
 .UNSPECIFIED.,.F.,.F.,(3,3),(0.,1.),.UNSPECIFIED.);
#1613=B_SPLINE_CURVE_WITH_KNOTS('',2,(#68344,#68345,#68346),
 .UNSPECIFIED.,.F.,.F.,(3,3),(0.,1.),.UNSPECIFIED.);
#1614=B_SPLINE_CURVE_WITH_KNOTS('',2,(#68349,#68350,#68351),
 .UNSPECIFIED.,.F.,.F.,(3,3),(0.,1.),.UNSPECIFIED.);
#1615=B_SPLINE_CURVE_WITH_KNOTS('',2,(#68359,#68360,#68361),
 .UNSPECIFIED.,.F.,.F.,(3,3),(0.,1.),.UNSPECIFIED.);
#1616=B_SPLINE_CURVE_WITH_KNOTS('',2,(#68364,#68365,#68366),
 .UNSPECIFIED.,.F.,.F.,(3,3),(0.,1.),.UNSPECIFIED.);
#1617=B_SPLINE_CURVE_WITH_KNOTS('',2,(#68374,#68375,#68376),
 .UNSPECIFIED.,.F.,.F.,(3,3),(0.,1.),.UNSPECIFIED.);
#1618=B_SPLINE_CURVE_WITH_KNOTS('',2,(#68379,#68380,#68381),
 .UNSPECIFIED.,.F.,.F.,(3,3),(0.,1.),.UNSPECIFIED.);
#1619=B_SPLINE_CURVE_WITH_KNOTS('',2,(#68389,#68390,#68391),
 .UNSPECIFIED.,.F.,.F.,(3,3),(0.,1.),.UNSPECIFIED.);
#1620=B_SPLINE_CURVE_WITH_KNOTS('',2,(#68394,#68395,#68396),
 .UNSPECIFIED.,.F.,.F.,(3,3),(0.,1.),.UNSPECIFIED.);
#1621=B_SPLINE_CURVE_WITH_KNOTS('',2,(#68403,#68404,#68405),
 .UNSPECIFIED.,.F.,.F.,(3,3),(0.,1.),.UNSPECIFIED.);
#1622=B_SPLINE_CURVE_WITH_KNOTS('',2,(#68406,#68407,#68408),
 .UNSPECIFIED.,.F.,.F.,(3,3),(0.,1.),.UNSPECIFIED.);
#1623=B_SPLINE_CURVE_WITH_KNOTS('',2,(#68417,#68418,#68419),
 .UNSPECIFIED.,.F.,.F.,(3,3),(0.,1.),.UNSPECIFIED.);
#1624=B_SPLINE_CURVE_WITH_KNOTS('',2,(#68423,#68424,#68425),
 .UNSPECIFIED.,.F.,.F.,(3,3),(0.,1.),.UNSPECIFIED.);
#1625=B_SPLINE_CURVE_WITH_KNOTS('',2,(#68434,#68435,#68436),
 .UNSPECIFIED.,.F.,.F.,(3,3),(0.,1.),.UNSPECIFIED.);
#1626=B_SPLINE_CURVE_WITH_KNOTS('',2,(#68439,#68440,#68441),
 .UNSPECIFIED.,.F.,.F.,(3,3),(0.,1.),.UNSPECIFIED.);
#1627=B_SPLINE_CURVE_WITH_KNOTS('',2,(#68449,#68450,#68451),
 .UNSPECIFIED.,.F.,.F.,(3,3),(0.,1.),.UNSPECIFIED.);
#1628=B_SPLINE_CURVE_WITH_KNOTS('',2,(#68454,#68455,#68456),
 .UNSPECIFIED.,.F.,.F.,(3,3),(0.,1.),.UNSPECIFIED.);
#1629=B_SPLINE_CURVE_WITH_KNOTS('',2,(#68464,#68465,#68466),
 .UNSPECIFIED.,.F.,.F.,(3,3),(0.,1.),.UNSPECIFIED.);
#1630=B_SPLINE_CURVE_WITH_KNOTS('',2,(#68469,#68470,#68471),
 .UNSPECIFIED.,.F.,.F.,(3,3),(0.,1.),.UNSPECIFIED.);
#1631=B_SPLINE_CURVE_WITH_KNOTS('',2,(#68479,#68480,#68481),
 .UNSPECIFIED.,.F.,.F.,(3,3),(0.,1.),.UNSPECIFIED.);
#1632=B_SPLINE_CURVE_WITH_KNOTS('',2,(#68484,#68485,#68486),
 .UNSPECIFIED.,.F.,.F.,(3,3),(0.,1.),.UNSPECIFIED.);
#1633=B_SPLINE_CURVE_WITH_KNOTS('',2,(#68494,#68495,#68496),
 .UNSPECIFIED.,.F.,.F.,(3,3),(0.,1.),.UNSPECIFIED.);
#1634=B_SPLINE_CURVE_WITH_KNOTS('',2,(#68499,#68500,#68501),
 .UNSPECIFIED.,.F.,.F.,(3,3),(0.,1.),.UNSPECIFIED.);
#1635=B_SPLINE_CURVE_WITH_KNOTS('',2,(#68509,#68510,#68511),
 .UNSPECIFIED.,.F.,.F.,(3,3),(0.,1.),.UNSPECIFIED.);
#1636=B_SPLINE_CURVE_WITH_KNOTS('',2,(#68514,#68515,#68516),
 .UNSPECIFIED.,.F.,.F.,(3,3),(0.,1.),.UNSPECIFIED.);
#1637=B_SPLINE_CURVE_WITH_KNOTS('',2,(#68524,#68525,#68526),
 .UNSPECIFIED.,.F.,.F.,(3,3),(0.,1.),.UNSPECIFIED.);
#1638=B_SPLINE_CURVE_WITH_KNOTS('',2,(#68529,#68530,#68531),
 .UNSPECIFIED.,.F.,.F.,(3,3),(0.,1.),.UNSPECIFIED.);
#1639=B_SPLINE_CURVE_WITH_KNOTS('',2,(#68538,#68539,#68540),
 .UNSPECIFIED.,.F.,.F.,(3,3),(0.,1.),.UNSPECIFIED.);
#1640=B_SPLINE_CURVE_WITH_KNOTS('',2,(#68541,#68542,#68543),
 .UNSPECIFIED.,.F.,.F.,(3,3),(0.,1.),.UNSPECIFIED.);
#1641=B_SPLINE_CURVE_WITH_KNOTS('',2,(#68552,#68553,#68554),
 .UNSPECIFIED.,.F.,.F.,(3,3),(0.,1.),.UNSPECIFIED.);
#1642=B_SPLINE_CURVE_WITH_KNOTS('',2,(#68558,#68559,#68560),
 .UNSPECIFIED.,.F.,.F.,(3,3),(0.,1.),.UNSPECIFIED.);
#1643=B_SPLINE_CURVE_WITH_KNOTS('',2,(#68569,#68570,#68571),
 .UNSPECIFIED.,.F.,.F.,(3,3),(0.,1.),.UNSPECIFIED.);
#1644=B_SPLINE_CURVE_WITH_KNOTS('',2,(#68574,#68575,#68576),
 .UNSPECIFIED.,.F.,.F.,(3,3),(0.,1.),.UNSPECIFIED.);
#1645=B_SPLINE_CURVE_WITH_KNOTS('',2,(#68584,#68585,#68586),
 .UNSPECIFIED.,.F.,.F.,(3,3),(0.,1.),.UNSPECIFIED.);
#1646=B_SPLINE_CURVE_WITH_KNOTS('',2,(#68589,#68590,#68591),
 .UNSPECIFIED.,.F.,.F.,(3,3),(0.,1.),.UNSPECIFIED.);
#1647=B_SPLINE_CURVE_WITH_KNOTS('',2,(#68599,#68600,#68601),
 .UNSPECIFIED.,.F.,.F.,(3,3),(0.,1.),.UNSPECIFIED.);
#1648=B_SPLINE_CURVE_WITH_KNOTS('',2,(#68604,#68605,#68606),
 .UNSPECIFIED.,.F.,.F.,(3,3),(0.,1.),.UNSPECIFIED.);
#1649=B_SPLINE_CURVE_WITH_KNOTS('',2,(#68614,#68615,#68616),
 .UNSPECIFIED.,.F.,.F.,(3,3),(0.,1.),.UNSPECIFIED.);
#1650=B_SPLINE_CURVE_WITH_KNOTS('',2,(#68619,#68620,#68621),
 .UNSPECIFIED.,.F.,.F.,(3,3),(0.,1.),.UNSPECIFIED.);
#1651=B_SPLINE_CURVE_WITH_KNOTS('',2,(#68629,#68630,#68631),
 .UNSPECIFIED.,.F.,.F.,(3,3),(0.,1.),.UNSPECIFIED.);
#1652=B_SPLINE_CURVE_WITH_KNOTS('',2,(#68634,#68635,#68636),
 .UNSPECIFIED.,.F.,.F.,(3,3),(0.,1.),.UNSPECIFIED.);
#1653=B_SPLINE_CURVE_WITH_KNOTS('',2,(#68644,#68645,#68646),
 .UNSPECIFIED.,.F.,.F.,(3,3),(0.,1.),.UNSPECIFIED.);
#1654=B_SPLINE_CURVE_WITH_KNOTS('',2,(#68649,#68650,#68651),
 .UNSPECIFIED.,.F.,.F.,(3,3),(0.,1.),.UNSPECIFIED.);
#1655=B_SPLINE_CURVE_WITH_KNOTS('',2,(#68659,#68660,#68661),
 .UNSPECIFIED.,.F.,.F.,(3,3),(0.,1.),.UNSPECIFIED.);
#1656=B_SPLINE_CURVE_WITH_KNOTS('',2,(#68664,#68665,#68666),
 .UNSPECIFIED.,.F.,.F.,(3,3),(0.,1.),.UNSPECIFIED.);
#1657=B_SPLINE_CURVE_WITH_KNOTS('',2,(#68674,#68675,#68676),
 .UNSPECIFIED.,.F.,.F.,(3,3),(0.,1.),.UNSPECIFIED.);
#1658=B_SPLINE_CURVE_WITH_KNOTS('',2,(#68679,#68680,#68681),
 .UNSPECIFIED.,.F.,.F.,(3,3),(0.,1.),.UNSPECIFIED.);
#1659=B_SPLINE_CURVE_WITH_KNOTS('',2,(#68689,#68690,#68691),
 .UNSPECIFIED.,.F.,.F.,(3,3),(0.,1.),.UNSPECIFIED.);
#1660=B_SPLINE_CURVE_WITH_KNOTS('',2,(#68694,#68695,#68696),
 .UNSPECIFIED.,.F.,.F.,(3,3),(0.,1.),.UNSPECIFIED.);
#1661=B_SPLINE_CURVE_WITH_KNOTS('',2,(#68704,#68705,#68706),
 .UNSPECIFIED.,.F.,.F.,(3,3),(0.,1.),.UNSPECIFIED.);
#1662=B_SPLINE_CURVE_WITH_KNOTS('',2,(#68709,#68710,#68711),
 .UNSPECIFIED.,.F.,.F.,(3,3),(0.,1.),.UNSPECIFIED.);
#1663=B_SPLINE_CURVE_WITH_KNOTS('',2,(#68719,#68720,#68721),
 .UNSPECIFIED.,.F.,.F.,(3,3),(0.,1.),.UNSPECIFIED.);
#1664=B_SPLINE_CURVE_WITH_KNOTS('',2,(#68724,#68725,#68726),
 .UNSPECIFIED.,.F.,.F.,(3,3),(0.,1.),.UNSPECIFIED.);
#1665=B_SPLINE_CURVE_WITH_KNOTS('',2,(#68734,#68735,#68736),
 .UNSPECIFIED.,.F.,.F.,(3,3),(0.,1.),.UNSPECIFIED.);
#1666=B_SPLINE_CURVE_WITH_KNOTS('',2,(#68739,#68740,#68741),
 .UNSPECIFIED.,.F.,.F.,(3,3),(0.,1.),.UNSPECIFIED.);
#1667=B_SPLINE_CURVE_WITH_KNOTS('',2,(#68749,#68750,#68751),
 .UNSPECIFIED.,.F.,.F.,(3,3),(0.,1.),.UNSPECIFIED.);
#1668=B_SPLINE_CURVE_WITH_KNOTS('',2,(#68754,#68755,#68756),
 .UNSPECIFIED.,.F.,.F.,(3,3),(0.,1.),.UNSPECIFIED.);
#1669=B_SPLINE_CURVE_WITH_KNOTS('',2,(#68764,#68765,#68766),
 .UNSPECIFIED.,.F.,.F.,(3,3),(0.,1.),.UNSPECIFIED.);
#1670=B_SPLINE_CURVE_WITH_KNOTS('',2,(#68769,#68770,#68771),
 .UNSPECIFIED.,.F.,.F.,(3,3),(0.,1.),.UNSPECIFIED.);
#1671=B_SPLINE_CURVE_WITH_KNOTS('',2,(#68778,#68779,#68780),
 .UNSPECIFIED.,.F.,.F.,(3,3),(0.,1.),.UNSPECIFIED.);
#1672=B_SPLINE_CURVE_WITH_KNOTS('',2,(#68781,#68782,#68783),
 .UNSPECIFIED.,.F.,.F.,(3,3),(0.,1.),.UNSPECIFIED.);
#1673=B_SPLINE_CURVE_WITH_KNOTS('',3,(#68790,#68791,#68792,#68793,#68794,
#68795,#68796,#68797,#68798,#68799,#68800,#68801,#68802,#68803,#68804,#68805,
#68806,#68807,#68808,#68809,#68810,#68811,#68812,#68813,#68814,#68815,#68816,
#68817,#68818,#68819,#68820,#68821,#68822,#68823,#68824,#68825,#68826,#68827,
#68828,#68829,#68830,#68831,#68832,#68833,#68834,#68835,#68836,#68837,#68838,
#68839,#68840,#68841,#68842,#68843,#68844,#68845,#68846,#68847,#68848,#68849,
#68850,#68851,#68852,#68853,#68854,#68855,#68856,#68857,#68858,#68859,#68860,
#68861,#68862),.UNSPECIFIED.,.F.,.F.,(4,3,3,3,3,3,3,3,3,3,3,3,3,3,3,3,3,
3,3,3,3,3,3,3,4),(-1.5337369924875,-1.47614434194274,-1.38903457285003,
-1.35939767545676,-1.33406695848438,-1.23088611202814,-1.19147645830862,
-1.16614958179783,-1.1277052655719,-1.02513486077225,-0.955412872192556,
-0.901872933084063,-0.873045820076336,-0.765171934991001,-0.671173342986202,
-0.616456444662515,-0.58488614612667,-0.476926645981598,-0.389177566971804,
-0.338395442046788,-0.310738024076525,-0.288566068862146,-0.179389393286242,
-0.0693222977829609,0.),.UNSPECIFIED.);
#1674=B_SPLINE_CURVE_WITH_KNOTS('',3,(#68867,#68868,#68869,#68870,#68871,
#68872,#68873,#68874,#68875,#68876,#68877,#68878,#68879,#68880,#68881,#68882,
#68883,#68884,#68885,#68886,#68887,#68888,#68889,#68890,#68891,#68892,#68893,
#68894,#68895,#68896,#68897,#68898,#68899,#68900,#68901,#68902,#68903,#68904,
#68905,#68906,#68907,#68908,#68909,#68910,#68911,#68912,#68913,#68914,#68915,
#68916,#68917,#68918,#68919,#68920,#68921,#68922,#68923,#68924,#68925,#68926,
#68927,#68928,#68929,#68930,#68931,#68932,#68933,#68934,#68935,#68936,#68937,
#68938,#68939,#68940,#68941,#68942,#68943,#68944,#68945),.UNSPECIFIED.,
 .F.,.F.,(4,3,3,3,3,3,3,3,3,3,3,3,3,3,3,3,3,3,3,3,3,3,3,3,3,3,4),(-1.52870610664513,
-1.46224068530639,-1.36596309804718,-1.32440296404387,-1.2951147317008,
-1.18612253398519,-1.14615032738057,-1.1200232336817,-1.0958154346986,-1.07713033626957,
-0.970210386711197,-0.864245604343508,-0.830831276447041,-0.810033160995986,
-0.704712885007061,-0.614931313624051,-0.566215947085015,-0.5441889725864,
-0.52276593090361,-0.420925957142934,-0.345586599475019,-0.297497915232979,
-0.271800404456334,-0.25273374406439,-0.152661671243804,-0.0544537748451435,
0.),.UNSPECIFIED.);
#1675=B_SPLINE_CURVE_WITH_KNOTS('',3,(#69694,#69695,#69696,#69697),
 .UNSPECIFIED.,.F.,.F.,(4,4),(89.0882430066573,89.5008331081196),
 .UNSPECIFIED.);
#1676=B_SPLINE_CURVE_WITH_KNOTS('',3,(#69699,#69700,#69701,#69702,#69703,
#69704,#69705,#69706,#69707,#69708,#69709,#69710,#69711,#69712,#69713,#69714,
#69715,#69716,#69717,#69718,#69719,#69720,#69721,#69722,#69723,#69724,#69725,
#69726,#69727,#69728,#69729,#69730,#69731,#69732,#69733,#69734,#69735,#69736,
#69737,#69738,#69739,#69740,#69741,#69742,#69743,#69744,#69745,#69746,#69747,
#69748,#69749,#69750,#69751,#69752,#69753,#69754,#69755,#69756,#69757,#69758,
#69759,#69760,#69761,#69762,#69763,#69764,#69765,#69766,#69767,#69768,#69769,
#69770,#69771),.UNSPECIFIED.,.F.,.F.,(4,3,3,3,3,3,3,3,3,3,3,3,3,3,3,3,3,
3,3,3,3,3,3,3,4),(-1.53373699248748,-1.47614434194271,-1.38903457285,-1.35939768361858,
-1.33406696685154,-1.23088611621171,-1.19147646127634,-1.16614958291887,
-1.12770526557188,-1.02513485497022,-0.955412885820892,-0.901872950742785,
-0.87304581950843,-0.765171934991016,-0.671173342986216,-0.616456453073865,
-0.584886146683686,-0.476926640886848,-0.389177566971813,-0.338395437911183,
-0.310738015345227,-0.288566061371844,-0.179389433105355,-0.0693223098585095,
0.),.UNSPECIFIED.);
#1677=B_SPLINE_CURVE_WITH_KNOTS('',3,(#69772,#69773,#69774,#69775,#69776,
#69777,#69778,#69779,#69780,#69781,#69782,#69783,#69784,#69785),
 .UNSPECIFIED.,.F.,.F.,(4,1,1,1,1,1,1,1,1,1,1,4),(10.3761157273101,10.7896026128002,
11.287297284435,11.7849919560698,12.2826866277046,12.7803812993394,13.2780759709742,
13.775770642609,14.2734653142438,14.7711599858786,15.2688546575134,15.7079632679489),
 .UNSPECIFIED.);
#1678=B_SPLINE_CURVE_WITH_KNOTS('',3,(#69791,#69792,#69793,#69794,#69795,
#69796,#69797,#69798,#69799,#69800,#69801,#69802,#69803,#69804,#69805,#69806,
#69807,#69808,#69809,#69810,#69811,#69812,#69813,#69814,#69815,#69816,#69817,
#69818,#69819,#69820,#69821,#69822,#69823,#69824,#69825,#69826,#69827,#69828,
#69829,#69830,#69831,#69832,#69833,#69834,#69835,#69836,#69837,#69838,#69839,
#69840,#69841,#69842,#69843,#69844,#69845,#69846,#69847,#69848,#69849,#69850,
#69851,#69852,#69853,#69854,#69855,#69856,#69857,#69858,#69859,#69860,#69861,
#69862,#69863,#69864,#69865,#69866,#69867,#69868,#69869),.UNSPECIFIED.,
 .F.,.F.,(4,3,3,3,3,3,3,3,3,3,3,3,3,3,3,3,3,3,3,3,3,3,3,3,3,3,4),(-1.52870610664512,
-1.46224068530633,-1.36596309804712,-1.32440295915268,-1.29511472974395,
-1.18612253300673,-1.1461503275642,-1.12002323492101,-1.09581543513247,
-1.07713033626952,-0.970210390750287,-0.864245635359953,-0.830831234316541,
-0.810033082630868,-0.70471288500701,-0.614931313624002,-0.566215946319255,
-0.544188965889431,-0.522765927890383,-0.4209259135058,-0.345586599474978,
-0.297497900017229,-0.271800352260087,-0.252733663988387,-0.15266159062613,
-0.0544537709407456,0.),.UNSPECIFIED.);
#1679=B_SPLINE_CURVE_WITH_KNOTS('',3,(#69872,#69873,#69874,#69875,#69876,
#69877,#69878,#69879,#69880,#69881,#69882,#69883),.UNSPECIFIED.,.F.,.F.,
(4,1,1,1,1,1,1,1,1,4),(11.6150328478182,12.112727519453,12.6104221910878,
13.1081168627226,13.6058115343574,14.1035062059922,14.601200877627,15.0988955492618,
15.5965902208966,15.7079632679489),.UNSPECIFIED.);
#2548=PLANE('',#28925);
#2549=PLANE('',#28926);
#2550=PLANE('',#28927);
#2551=PLANE('',#28928);
#2552=PLANE('',#28929);
#2553=PLANE('',#28930);
#2554=PLANE('',#28931);
#2555=PLANE('',#28932);
#2556=PLANE('',#28933);
#2557=PLANE('',#28934);
#2558=PLANE('',#28935);
#2559=PLANE('',#28936);
#2560=PLANE('',#28939);
#2561=PLANE('',#28948);
#2562=PLANE('',#28952);
#2563=PLANE('',#28953);
#2564=PLANE('',#28954);
#2565=PLANE('',#28955);
#2566=PLANE('',#28956);
#2567=PLANE('',#28957);
#2568=PLANE('',#28958);
#2569=PLANE('',#28959);
#3935=FACE_OUTER_BOUND('',#5498,.T.);
#3936=FACE_OUTER_BOUND('',#5499,.T.);
#3937=FACE_OUTER_BOUND('',#5500,.T.);
#3938=FACE_OUTER_BOUND('',#5501,.T.);
#3939=FACE_OUTER_BOUND('',#5502,.T.);
#3940=FACE_OUTER_BOUND('',#5503,.T.);
#3941=FACE_OUTER_BOUND('',#5504,.T.);
#3942=FACE_OUTER_BOUND('',#5505,.T.);
#3943=FACE_OUTER_BOUND('',#5506,.T.);
#3944=FACE_OUTER_BOUND('',#5507,.T.);
#3945=FACE_OUTER_BOUND('',#5508,.T.);
#3946=FACE_OUTER_BOUND('',#5509,.T.);
#3947=FACE_OUTER_BOUND('',#5510,.T.);
#3948=FACE_OUTER_BOUND('',#5511,.T.);
#3949=FACE_OUTER_BOUND('',#5512,.T.);
#3950=FACE_OUTER_BOUND('',#5513,.T.);
#3951=FACE_OUTER_BOUND('',#5514,.T.);
#3952=FACE_OUTER_BOUND('',#5515,.T.);
#3953=FACE_OUTER_BOUND('',#5516,.T.);
#3954=FACE_OUTER_BOUND('',#5517,.T.);
#3955=FACE_OUTER_BOUND('',#5518,.T.);
#3956=FACE_OUTER_BOUND('',#5519,.T.);
#3957=FACE_OUTER_BOUND('',#5520,.T.);
#3958=FACE_OUTER_BOUND('',#5521,.T.);
#3959=FACE_OUTER_BOUND('',#5522,.T.);
#3960=FACE_OUTER_BOUND('',#5523,.T.);
#3961=FACE_OUTER_BOUND('',#5524,.T.);
#3962=FACE_OUTER_BOUND('',#5525,.T.);
#3963=FACE_OUTER_BOUND('',#5526,.T.);
#3964=FACE_OUTER_BOUND('',#5527,.T.);
#3965=FACE_OUTER_BOUND('',#5528,.T.);
#3966=FACE_OUTER_BOUND('',#5529,.T.);
#3967=FACE_OUTER_BOUND('',#5530,.T.);
#3968=FACE_OUTER_BOUND('',#5531,.T.);
#3969=FACE_OUTER_BOUND('',#5532,.T.);
#3970=FACE_OUTER_BOUND('',#5533,.T.);
#3971=FACE_OUTER_BOUND('',#5534,.T.);
#3972=FACE_OUTER_BOUND('',#5535,.T.);
#3973=FACE_OUTER_BOUND('',#5536,.T.);
#3974=FACE_OUTER_BOUND('',#5537,.T.);
#3975=FACE_OUTER_BOUND('',#5538,.T.);
#3976=FACE_OUTER_BOUND('',#5539,.T.);
#3977=FACE_OUTER_BOUND('',#5540,.T.);
#3978=FACE_OUTER_BOUND('',#5541,.T.);
#3979=FACE_OUTER_BOUND('',#5542,.T.);
#3980=FACE_OUTER_BOUND('',#5543,.T.);
#3981=FACE_OUTER_BOUND('',#5544,.T.);
#3982=FACE_OUTER_BOUND('',#5545,.T.);
#3983=FACE_OUTER_BOUND('',#5546,.T.);
#3984=FACE_OUTER_BOUND('',#5547,.T.);
#3985=FACE_OUTER_BOUND('',#5548,.T.);
#3986=FACE_OUTER_BOUND('',#5549,.T.);
#3987=FACE_OUTER_BOUND('',#5550,.T.);
#3988=FACE_OUTER_BOUND('',#5551,.T.);
#3989=FACE_OUTER_BOUND('',#5552,.T.);
#3990=FACE_OUTER_BOUND('',#5553,.T.);
#3991=FACE_OUTER_BOUND('',#5554,.T.);
#3992=FACE_OUTER_BOUND('',#5555,.T.);
#3993=FACE_OUTER_BOUND('',#5556,.T.);
#3994=FACE_OUTER_BOUND('',#5557,.T.);
#3995=FACE_OUTER_BOUND('',#5558,.T.);
#3996=FACE_OUTER_BOUND('',#5559,.T.);
#3997=FACE_OUTER_BOUND('',#5560,.T.);
#3998=FACE_OUTER_BOUND('',#5563,.T.);
#3999=FACE_OUTER_BOUND('',#5564,.T.);
#4000=FACE_OUTER_BOUND('',#5565,.T.);
#4001=FACE_OUTER_BOUND('',#5566,.T.);
#4002=FACE_OUTER_BOUND('',#5567,.T.);
#4003=FACE_OUTER_BOUND('',#5568,.T.);
#4004=FACE_OUTER_BOUND('',#5569,.T.);
#4005=FACE_OUTER_BOUND('',#5570,.T.);
#4006=FACE_OUTER_BOUND('',#5571,.T.);
#4007=FACE_OUTER_BOUND('',#5572,.T.);
#4008=FACE_OUTER_BOUND('',#5573,.T.);
#4009=FACE_OUTER_BOUND('',#5574,.T.);
#4010=FACE_OUTER_BOUND('',#5575,.T.);
#4011=FACE_OUTER_BOUND('',#5576,.T.);
#4012=FACE_OUTER_BOUND('',#5577,.T.);
#4013=FACE_OUTER_BOUND('',#5578,.T.);
#4014=FACE_OUTER_BOUND('',#5579,.T.);
#4015=FACE_OUTER_BOUND('',#5580,.T.);
#4016=FACE_OUTER_BOUND('',#5581,.T.);
#4017=FACE_OUTER_BOUND('',#5582,.T.);
#4018=FACE_OUTER_BOUND('',#5583,.T.);
#4019=FACE_OUTER_BOUND('',#5584,.T.);
#4020=FACE_OUTER_BOUND('',#5585,.T.);
#4021=FACE_OUTER_BOUND('',#5586,.T.);
#4022=FACE_OUTER_BOUND('',#5587,.T.);
#4023=FACE_OUTER_BOUND('',#5588,.T.);
#4024=FACE_OUTER_BOUND('',#5589,.T.);
#4025=FACE_OUTER_BOUND('',#5590,.T.);
#4026=FACE_OUTER_BOUND('',#5591,.T.);
#4027=FACE_OUTER_BOUND('',#5592,.T.);
#4028=FACE_OUTER_BOUND('',#5593,.T.);
#4029=FACE_OUTER_BOUND('',#5594,.T.);
#4030=FACE_OUTER_BOUND('',#5595,.T.);
#4031=FACE_OUTER_BOUND('',#5596,.T.);
#4032=FACE_OUTER_BOUND('',#5597,.T.);
#4033=FACE_OUTER_BOUND('',#5598,.T.);
#4034=FACE_OUTER_BOUND('',#5599,.T.);
#4035=FACE_OUTER_BOUND('',#5600,.T.);
#4036=FACE_OUTER_BOUND('',#5601,.T.);
#4037=FACE_OUTER_BOUND('',#5604,.T.);
#4038=FACE_OUTER_BOUND('',#5605,.T.);
#4039=FACE_OUTER_BOUND('',#5606,.T.);
#4040=FACE_OUTER_BOUND('',#5607,.T.);
#4041=FACE_OUTER_BOUND('',#5608,.T.);
#4042=FACE_OUTER_BOUND('',#5609,.T.);
#4043=FACE_OUTER_BOUND('',#5610,.T.);
#4044=FACE_OUTER_BOUND('',#5611,.T.);
#4045=FACE_OUTER_BOUND('',#5612,.T.);
#4046=FACE_OUTER_BOUND('',#5613,.T.);
#4047=FACE_OUTER_BOUND('',#5614,.T.);
#4048=FACE_OUTER_BOUND('',#5616,.T.);
#4049=FACE_OUTER_BOUND('',#5617,.T.);
#4050=FACE_OUTER_BOUND('',#5618,.T.);
#4051=FACE_OUTER_BOUND('',#5619,.T.);
#4052=FACE_OUTER_BOUND('',#5620,.T.);
#4053=FACE_OUTER_BOUND('',#5621,.T.);
#4054=FACE_OUTER_BOUND('',#5622,.T.);
#4055=FACE_OUTER_BOUND('',#5623,.T.);
#4056=FACE_OUTER_BOUND('',#5624,.T.);
#4057=FACE_OUTER_BOUND('',#5628,.T.);
#4058=FACE_OUTER_BOUND('',#5629,.T.);
#5498=EDGE_LOOP('',(#24614,#24615,#24616,#24617));
#5499=EDGE_LOOP('',(#24618,#24619,#24620,#24621));
#5500=EDGE_LOOP('',(#24622,#24623,#24624,#24625));
#5501=EDGE_LOOP('',(#24626,#24627,#24628,#24629));
#5502=EDGE_LOOP('',(#24630,#24631,#24632,#24633));
#5503=EDGE_LOOP('',(#24634,#24635,#24636,#24637));
#5504=EDGE_LOOP('',(#24638,#24639,#24640,#24641));
#5505=EDGE_LOOP('',(#24642,#24643,#24644,#24645));
#5506=EDGE_LOOP('',(#24646,#24647,#24648,#24649));
#5507=EDGE_LOOP('',(#24650,#24651,#24652,#24653));
#5508=EDGE_LOOP('',(#24654,#24655,#24656,#24657));
#5509=EDGE_LOOP('',(#24658,#24659,#24660,#24661));
#5510=EDGE_LOOP('',(#24662,#24663,#24664,#24665));
#5511=EDGE_LOOP('',(#24666,#24667,#24668,#24669));
#5512=EDGE_LOOP('',(#24670,#24671,#24672,#24673,#24674));
#5513=EDGE_LOOP('',(#24675,#24676,#24677,#24678));
#5514=EDGE_LOOP('',(#24679,#24680,#24681,#24682));
#5515=EDGE_LOOP('',(#24683,#24684,#24685,#24686));
#5516=EDGE_LOOP('',(#24687,#24688,#24689,#24690));
#5517=EDGE_LOOP('',(#24691,#24692,#24693,#24694));
#5518=EDGE_LOOP('',(#24695,#24696,#24697,#24698));
#5519=EDGE_LOOP('',(#24699,#24700,#24701,#24702));
#5520=EDGE_LOOP('',(#24703,#24704,#24705,#24706));
#5521=EDGE_LOOP('',(#24707,#24708,#24709,#24710));
#5522=EDGE_LOOP('',(#24711,#24712,#24713,#24714));
#5523=EDGE_LOOP('',(#24715,#24716,#24717,#24718));
#5524=EDGE_LOOP('',(#24719,#24720,#24721,#24722));
#5525=EDGE_LOOP('',(#24723,#24724,#24725,#24726));
#5526=EDGE_LOOP('',(#24727,#24728,#24729,#24730));
#5527=EDGE_LOOP('',(#24731,#24732,#24733,#24734));
#5528=EDGE_LOOP('',(#24735,#24736,#24737,#24738));
#5529=EDGE_LOOP('',(#24739,#24740,#24741,#24742));
#5530=EDGE_LOOP('',(#24743,#24744,#24745,#24746));
#5531=EDGE_LOOP('',(#24747,#24748,#24749,#24750));
#5532=EDGE_LOOP('',(#24751,#24752,#24753,#24754));
#5533=EDGE_LOOP('',(#24755,#24756,#24757,#24758));
#5534=EDGE_LOOP('',(#24759,#24760,#24761,#24762));
#5535=EDGE_LOOP('',(#24763,#24764,#24765,#24766));
#5536=EDGE_LOOP('',(#24767,#24768,#24769,#24770));
#5537=EDGE_LOOP('',(#24771,#24772,#24773,#24774));
#5538=EDGE_LOOP('',(#24775,#24776,#24777,#24778));
#5539=EDGE_LOOP('',(#24779,#24780,#24781,#24782));
#5540=EDGE_LOOP('',(#24783,#24784,#24785,#24786));
#5541=EDGE_LOOP('',(#24787,#24788,#24789,#24790));
#5542=EDGE_LOOP('',(#24791,#24792,#24793,#24794));
#5543=EDGE_LOOP('',(#24795,#24796,#24797,#24798));
#5544=EDGE_LOOP('',(#24799,#24800,#24801,#24802));
#5545=EDGE_LOOP('',(#24803,#24804,#24805,#24806));
#5546=EDGE_LOOP('',(#24807,#24808,#24809,#24810));
#5547=EDGE_LOOP('',(#24811,#24812,#24813,#24814));
#5548=EDGE_LOOP('',(#24815,#24816,#24817,#24818));
#5549=EDGE_LOOP('',(#24819,#24820,#24821,#24822));
#5550=EDGE_LOOP('',(#24823,#24824,#24825,#24826));
#5551=EDGE_LOOP('',(#24827,#24828,#24829,#24830));
#5552=EDGE_LOOP('',(#24831,#24832,#24833,#24834));
#5553=EDGE_LOOP('',(#24835,#24836,#24837,#24838));
#5554=EDGE_LOOP('',(#24839,#24840,#24841,#24842));
#5555=EDGE_LOOP('',(#24843,#24844,#24845,#24846));
#5556=EDGE_LOOP('',(#24847,#24848,#24849,#24850));
#5557=EDGE_LOOP('',(#24851,#24852,#24853,#24854));
#5558=EDGE_LOOP('',(#24855,#24856,#24857,#24858));
#5559=EDGE_LOOP('',(#24859,#24860,#24861,#24862));
#5560=EDGE_LOOP('',(#24863,#24864,#24865,#24866,#24867,#24868,#24869,#24870,
#24871,#24872,#24873,#24874,#24875,#24876,#24877,#24878));
#5561=EDGE_LOOP('',(#24879,#24880,#24881,#24882,#24883,#24884,#24885,#24886,
#24887));
#5562=EDGE_LOOP('',(#24888,#24889,#24890,#24891,#24892,#24893,#24894,#24895));
#5563=EDGE_LOOP('',(#24896,#24897,#24898,#24899));
#5564=EDGE_LOOP('',(#24900,#24901,#24902,#24903));
#5565=EDGE_LOOP('',(#24904,#24905,#24906,#24907));
#5566=EDGE_LOOP('',(#24908,#24909,#24910,#24911));
#5567=EDGE_LOOP('',(#24912,#24913,#24914,#24915));
#5568=EDGE_LOOP('',(#24916,#24917,#24918,#24919));
#5569=EDGE_LOOP('',(#24920,#24921,#24922,#24923));
#5570=EDGE_LOOP('',(#24924,#24925,#24926,#24927));
#5571=EDGE_LOOP('',(#24928,#24929,#24930,#24931));
#5572=EDGE_LOOP('',(#24932,#24933,#24934,#24935));
#5573=EDGE_LOOP('',(#24936,#24937,#24938,#24939));
#5574=EDGE_LOOP('',(#24940,#24941,#24942,#24943));
#5575=EDGE_LOOP('',(#24944,#24945,#24946,#24947));
#5576=EDGE_LOOP('',(#24948,#24949,#24950,#24951));
#5577=EDGE_LOOP('',(#24952,#24953,#24954,#24955));
#5578=EDGE_LOOP('',(#24956,#24957,#24958,#24959));
#5579=EDGE_LOOP('',(#24960,#24961,#24962,#24963));
#5580=EDGE_LOOP('',(#24964,#24965,#24966,#24967));
#5581=EDGE_LOOP('',(#24968,#24969,#24970,#24971));
#5582=EDGE_LOOP('',(#24972,#24973,#24974,#24975));
#5583=EDGE_LOOP('',(#24976,#24977,#24978,#24979));
#5584=EDGE_LOOP('',(#24980,#24981,#24982,#24983));
#5585=EDGE_LOOP('',(#24984,#24985,#24986,#24987));
#5586=EDGE_LOOP('',(#24988,#24989,#24990,#24991));
#5587=EDGE_LOOP('',(#24992,#24993,#24994,#24995));
#5588=EDGE_LOOP('',(#24996,#24997,#24998,#24999));
#5589=EDGE_LOOP('',(#25000,#25001,#25002,#25003));
#5590=EDGE_LOOP('',(#25004,#25005,#25006,#25007));
#5591=EDGE_LOOP('',(#25008,#25009,#25010,#25011));
#5592=EDGE_LOOP('',(#25012,#25013,#25014,#25015));
#5593=EDGE_LOOP('',(#25016,#25017,#25018,#25019));
#5594=EDGE_LOOP('',(#25020,#25021,#25022,#25023));
#5595=EDGE_LOOP('',(#25024,#25025,#25026,#25027));
#5596=EDGE_LOOP('',(#25028,#25029,#25030,#25031));
#5597=EDGE_LOOP('',(#25032,#25033,#25034,#25035));
#5598=EDGE_LOOP('',(#25036,#25037,#25038,#25039));
#5599=EDGE_LOOP('',(#25040,#25041,#25042,#25043));
#5600=EDGE_LOOP('',(#25044,#25045,#25046,#25047));
#5601=EDGE_LOOP('',(#25048,#25049,#25050,#25051,#25052,#25053,#25054,#25055,
#25056,#25057,#25058,#25059,#25060,#25061,#25062,#25063));
#5602=EDGE_LOOP('',(#25064,#25065,#25066,#25067,#25068,#25069,#25070,#25071,
#25072));
#5603=EDGE_LOOP('',(#25073,#25074,#25075,#25076,#25077,#25078,#25079,#25080));
#5604=EDGE_LOOP('',(#25081,#25082,#25083,#25084,#25085,#25086,#25087,#25088,
#25089));
#5605=EDGE_LOOP('',(#25090,#25091,#25092,#25093,#25094,#25095,#25096,#25097));
#5606=EDGE_LOOP('',(#25098,#25099,#25100,#25101,#25102,#25103,#25104,#25105,
#25106));
#5607=EDGE_LOOP('',(#25107,#25108,#25109,#25110,#25111,#25112,#25113,#25114));
#5608=EDGE_LOOP('',(#25115,#25116,#25117,#25118,#25119));
#5609=EDGE_LOOP('',(#25120,#25121,#25122,#25123,#25124,#25125,#25126,#25127,
#25128,#25129,#25130,#25131,#25132,#25133,#25134,#25135,#25136,#25137,#25138,
#25139,#25140,#25141,#25142,#25143,#25144,#25145,#25146,#25147,#25148,#25149,
#25150,#25151,#25152));
#5610=EDGE_LOOP('',(#25153,#25154,#25155,#25156,#25157));
#5611=EDGE_LOOP('',(#25158,#25159,#25160,#25161));
#5612=EDGE_LOOP('',(#25162,#25163,#25164,#25165,#25166,#25167,#25168,#25169,
#25170,#25171,#25172,#25173,#25174,#25175,#25176,#25177,#25178,#25179,#25180,
#25181,#25182,#25183,#25184,#25185,#25186,#25187,#25188,#25189,#25190,#25191,
#25192,#25193));
#5613=EDGE_LOOP('',(#25194,#25195,#25196,#25197,#25198,#25199,#25200));
#5614=EDGE_LOOP('',(#25201,#25202,#25203,#25204,#25205,#25206));
#5615=EDGE_LOOP('',(#25207));
#5616=EDGE_LOOP('',(#25208,#25209,#25210));
#5617=EDGE_LOOP('',(#25211,#25212,#25213,#25214,#25215,#25216,#25217,#25218,
#25219,#25220));
#5618=EDGE_LOOP('',(#25221,#25222,#25223,#25224));
#5619=EDGE_LOOP('',(#25225,#25226,#25227,#25228));
#5620=EDGE_LOOP('',(#25229,#25230,#25231,#25232));
#5621=EDGE_LOOP('',(#25233,#25234,#25235,#25236));
#5622=EDGE_LOOP('',(#25237,#25238,#25239,#25240));
#5623=EDGE_LOOP('',(#25241,#25242,#25243,#25244,#25245));
#5624=EDGE_LOOP('',(#25246));
#5625=EDGE_LOOP('',(#25247,#25248,#25249,#25250,#25251,#25252,#25253,#25254,
#25255,#25256,#25257,#25258,#25259,#25260,#25261,#25262));
#5626=EDGE_LOOP('',(#25263,#25264,#25265,#25266));
#5627=EDGE_LOOP('',(#25267,#25268,#25269,#25270,#25271,#25272,#25273,#25274,
#25275,#25276,#25277,#25278,#25279,#25280,#25281,#25282));
#5628=EDGE_LOOP('',(#25283));
#5629=EDGE_LOOP('',(#25284,#25285,#25286,#25287,#25288,#25289));
#8006=LINE('',#66004,#10503);
#8007=LINE('',#66037,#10504);
#8008=LINE('',#66121,#10505);
#8009=LINE('',#66211,#10506);
#8010=LINE('',#66301,#10507);
#8011=LINE('',#66385,#10508);
#8012=LINE('',#66475,#10509);
#8013=LINE('',#66562,#10510);
#8014=LINE('',#66649,#10511);
#8015=LINE('',#66739,#10512);
#8016=LINE('',#66823,#10513);
#8017=LINE('',#66913,#10514);
#8018=LINE('',#67003,#10515);
#8019=LINE('',#67087,#10516);
#8020=LINE('',#67177,#10517);
#8021=LINE('',#67260,#10518);
#8022=LINE('',#67286,#10519);
#8023=LINE('',#67324,#10520);
#8024=LINE('',#67361,#10521);
#8025=LINE('',#67398,#10522);
#8026=LINE('',#67436,#10523);
#8027=LINE('',#67473,#10524);
#8028=LINE('',#67510,#10525);
#8029=LINE('',#67548,#10526);
#8030=LINE('',#67584,#10527);
#8031=LINE('',#67622,#10528);
#8032=LINE('',#67659,#10529);
#8033=LINE('',#67696,#10530);
#8034=LINE('',#67734,#10531);
#8035=LINE('',#67780,#10532);
#8036=LINE('',#67785,#10533);
#8037=LINE('',#67797,#10534);
#8038=LINE('',#67812,#10535);
#8039=LINE('',#67827,#10536);
#8040=LINE('',#67842,#10537);
#8041=LINE('',#67857,#10538);
#8042=LINE('',#67872,#10539);
#8043=LINE('',#67900,#10540);
#8044=LINE('',#67905,#10541);
#8045=LINE('',#67917,#10542);
#8046=LINE('',#67932,#10543);
#8047=LINE('',#67947,#10544);
#8048=LINE('',#67962,#10545);
#8049=LINE('',#67977,#10546);
#8050=LINE('',#67992,#10547);
#8051=LINE('',#68007,#10548);
#8052=LINE('',#68035,#10549);
#8053=LINE('',#68040,#10550);
#8054=LINE('',#68052,#10551);
#8055=LINE('',#68067,#10552);
#8056=LINE('',#68082,#10553);
#8057=LINE('',#68097,#10554);
#8058=LINE('',#68112,#10555);
#8059=LINE('',#68127,#10556);
#8060=LINE('',#68142,#10557);
#8061=LINE('',#68157,#10558);
#8062=LINE('',#68172,#10559);
#8063=LINE('',#68187,#10560);
#8064=LINE('',#68202,#10561);
#8065=LINE('',#68217,#10562);
#8066=LINE('',#68232,#10563);
#8067=LINE('',#68247,#10564);
#8068=LINE('',#68267,#10565);
#8069=LINE('',#68269,#10566);
#8070=LINE('',#68271,#10567);
#8071=LINE('',#68272,#10568);
#8072=LINE('',#68275,#10569);
#8073=LINE('',#68277,#10570);
#8074=LINE('',#68278,#10571);
#8075=LINE('',#68281,#10572);
#8076=LINE('',#68283,#10573);
#8077=LINE('',#68284,#10574);
#8078=LINE('',#68286,#10575);
#8079=LINE('',#68287,#10576);
#8080=LINE('',#68301,#10577);
#8081=LINE('',#68306,#10578);
#8082=LINE('',#68318,#10579);
#8083=LINE('',#68333,#10580);
#8084=LINE('',#68348,#10581);
#8085=LINE('',#68363,#10582);
#8086=LINE('',#68378,#10583);
#8087=LINE('',#68393,#10584);
#8088=LINE('',#68421,#10585);
#8089=LINE('',#68426,#10586);
#8090=LINE('',#68438,#10587);
#8091=LINE('',#68453,#10588);
#8092=LINE('',#68468,#10589);
#8093=LINE('',#68483,#10590);
#8094=LINE('',#68498,#10591);
#8095=LINE('',#68513,#10592);
#8096=LINE('',#68528,#10593);
#8097=LINE('',#68556,#10594);
#8098=LINE('',#68561,#10595);
#8099=LINE('',#68573,#10596);
#8100=LINE('',#68588,#10597);
#8101=LINE('',#68603,#10598);
#8102=LINE('',#68618,#10599);
#8103=LINE('',#68633,#10600);
#8104=LINE('',#68648,#10601);
#8105=LINE('',#68663,#10602);
#8106=LINE('',#68678,#10603);
#8107=LINE('',#68693,#10604);
#8108=LINE('',#68708,#10605);
#8109=LINE('',#68723,#10606);
#8110=LINE('',#68738,#10607);
#8111=LINE('',#68753,#10608);
#8112=LINE('',#68768,#10609);
#8113=LINE('',#70640,#10610);
#8114=LINE('',#70642,#10611);
#8115=LINE('',#70644,#10612);
#8116=LINE('',#70646,#10613);
#8117=LINE('',#70648,#10614);
#8118=LINE('',#70649,#10615);
#8119=LINE('',#70674,#10616);
#8120=LINE('',#70684,#10617);
#8121=LINE('',#70685,#10618);
#8122=LINE('',#70687,#10619);
#8123=LINE('',#70689,#10620);
#8124=LINE('',#70691,#10621);
#8125=LINE('',#70693,#10622);
#8126=LINE('',#70700,#10623);
#10503=VECTOR('',#35043,0.8);
#10504=VECTOR('',#35048,0.8);
#10505=VECTOR('',#35051,0.8);
#10506=VECTOR('',#35054,0.8);
#10507=VECTOR('',#35057,0.8);
#10508=VECTOR('',#35060,0.8);
#10509=VECTOR('',#35063,0.8);
#10510=VECTOR('',#35066,0.8);
#10511=VECTOR('',#35069,0.8);
#10512=VECTOR('',#35072,0.8);
#10513=VECTOR('',#35075,0.8);
#10514=VECTOR('',#35078,0.8);
#10515=VECTOR('',#35081,0.8);
#10516=VECTOR('',#35084,0.8);
#10517=VECTOR('',#35087,0.8);
#10518=VECTOR('',#35092,0.6767);
#10519=VECTOR('',#35097,0.6767);
#10520=VECTOR('',#35100,0.6767);
#10521=VECTOR('',#35103,0.6767);
#10522=VECTOR('',#35106,0.6767);
#10523=VECTOR('',#35109,0.6767);
#10524=VECTOR('',#35112,0.6767);
#10525=VECTOR('',#35115,0.6767);
#10526=VECTOR('',#35118,0.6767);
#10527=VECTOR('',#35121,0.6767);
#10528=VECTOR('',#35124,0.6767);
#10529=VECTOR('',#35127,0.6767);
#10530=VECTOR('',#35130,0.6767);
#10531=VECTOR('',#35133,0.6767);
#10532=VECTOR('',#35134,1.);
#10533=VECTOR('',#35135,1.);
#10534=VECTOR('',#35136,1.);
#10535=VECTOR('',#35137,1.);
#10536=VECTOR('',#35138,1.);
#10537=VECTOR('',#35139,1.);
#10538=VECTOR('',#35140,1.);
#10539=VECTOR('',#35141,1.);
#10540=VECTOR('',#35142,1.);
#10541=VECTOR('',#35143,1.);
#10542=VECTOR('',#35144,1.);
#10543=VECTOR('',#35145,1.);
#10544=VECTOR('',#35146,1.);
#10545=VECTOR('',#35147,1.);
#10546=VECTOR('',#35148,1.);
#10547=VECTOR('',#35149,1.);
#10548=VECTOR('',#35150,1.);
#10549=VECTOR('',#35151,1.);
#10550=VECTOR('',#35152,1.);
#10551=VECTOR('',#35153,1.);
#10552=VECTOR('',#35154,1.);
#10553=VECTOR('',#35155,1.);
#10554=VECTOR('',#35156,1.);
#10555=VECTOR('',#35157,1.);
#10556=VECTOR('',#35158,1.);
#10557=VECTOR('',#35159,1.);
#10558=VECTOR('',#35160,1.);
#10559=VECTOR('',#35161,1.);
#10560=VECTOR('',#35162,1.);
#10561=VECTOR('',#35163,1.);
#10562=VECTOR('',#35164,1.);
#10563=VECTOR('',#35165,1.);
#10564=VECTOR('',#35166,1.);
#10565=VECTOR('',#35171,1.);
#10566=VECTOR('',#35172,1.);
#10567=VECTOR('',#35173,1.);
#10568=VECTOR('',#35174,1.);
#10569=VECTOR('',#35177,1.);
#10570=VECTOR('',#35178,1.);
#10571=VECTOR('',#35179,1.);
#10572=VECTOR('',#35182,1.);
#10573=VECTOR('',#35183,1.);
#10574=VECTOR('',#35184,1.);
#10575=VECTOR('',#35187,1.);
#10576=VECTOR('',#35188,1.);
#10577=VECTOR('',#35191,1.);
#10578=VECTOR('',#35192,1.);
#10579=VECTOR('',#35193,1.);
#10580=VECTOR('',#35194,1.);
#10581=VECTOR('',#35195,1.);
#10582=VECTOR('',#35196,1.);
#10583=VECTOR('',#35197,1.);
#10584=VECTOR('',#35198,1.);
#10585=VECTOR('',#35199,1.);
#10586=VECTOR('',#35200,1.);
#10587=VECTOR('',#35201,1.);
#10588=VECTOR('',#35202,1.);
#10589=VECTOR('',#35203,1.);
#10590=VECTOR('',#35204,1.);
#10591=VECTOR('',#35205,1.);
#10592=VECTOR('',#35206,1.);
#10593=VECTOR('',#35207,1.);
#10594=VECTOR('',#35208,1.);
#10595=VECTOR('',#35209,1.);
#10596=VECTOR('',#35210,1.);
#10597=VECTOR('',#35211,1.);
#10598=VECTOR('',#35212,1.);
#10599=VECTOR('',#35213,1.);
#10600=VECTOR('',#35214,1.);
#10601=VECTOR('',#35215,1.);
#10602=VECTOR('',#35216,1.);
#10603=VECTOR('',#35217,1.);
#10604=VECTOR('',#35218,1.);
#10605=VECTOR('',#35219,1.);
#10606=VECTOR('',#35220,1.);
#10607=VECTOR('',#35221,1.);
#10608=VECTOR('',#35222,1.);
#10609=VECTOR('',#35223,1.);
#10610=VECTOR('',#35260,1.);
#10611=VECTOR('',#35261,1.);
#10612=VECTOR('',#35262,1.);
#10613=VECTOR('',#35263,1.);
#10614=VECTOR('',#35264,1.);
#10615=VECTOR('',#35265,1.);
#10616=VECTOR('',#35270,1.28782032302755);
#10617=VECTOR('',#35275,1.);
#10618=VECTOR('',#35276,1.);
#10619=VECTOR('',#35279,1.);
#10620=VECTOR('',#35282,1.);
#10621=VECTOR('',#35285,1.);
#10622=VECTOR('',#35288,1.);
#10623=VECTOR('',#35299,0.75);
#11126=CIRCLE('',#28894,0.7911);
#11127=CIRCLE('',#28909,0.7911);
#11128=CIRCLE('',#28911,0.6767);
#11129=CIRCLE('',#28937,0.7911);
#11130=CIRCLE('',#28938,0.7911);
#11131=CIRCLE('',#28940,0.7911);
#11132=CIRCLE('',#28941,0.7911);
#11133=CIRCLE('',#28942,0.6767);
#11134=CIRCLE('',#28945,0.8511);
#11135=CIRCLE('',#28946,0.06);
#11136=CIRCLE('',#28947,0.7911);
#11137=CIRCLE('',#28951,1.14);
#11138=CIRCLE('',#28960,0.7);
#13378=VERTEX_POINT('',#66002);
#13379=VERTEX_POINT('',#66003);
#13380=VERTEX_POINT('',#66005);
#13381=VERTEX_POINT('',#66022);
#13382=VERTEX_POINT('',#66035);
#13383=VERTEX_POINT('',#66036);
#13384=VERTEX_POINT('',#66119);
#13385=VERTEX_POINT('',#66120);
#13386=VERTEX_POINT('',#66209);
#13387=VERTEX_POINT('',#66210);
#13388=VERTEX_POINT('',#66299);
#13389=VERTEX_POINT('',#66300);
#13390=VERTEX_POINT('',#66383);
#13391=VERTEX_POINT('',#66384);
#13392=VERTEX_POINT('',#66473);
#13393=VERTEX_POINT('',#66474);
#13394=VERTEX_POINT('',#66560);
#13395=VERTEX_POINT('',#66561);
#13396=VERTEX_POINT('',#66647);
#13397=VERTEX_POINT('',#66648);
#13398=VERTEX_POINT('',#66737);
#13399=VERTEX_POINT('',#66738);
#13400=VERTEX_POINT('',#66821);
#13401=VERTEX_POINT('',#66822);
#13402=VERTEX_POINT('',#66911);
#13403=VERTEX_POINT('',#66912);
#13404=VERTEX_POINT('',#67001);
#13405=VERTEX_POINT('',#67002);
#13406=VERTEX_POINT('',#67085);
#13407=VERTEX_POINT('',#67086);
#13408=VERTEX_POINT('',#67175);
#13409=VERTEX_POINT('',#67176);
#13410=VERTEX_POINT('',#67178);
#13411=VERTEX_POINT('',#67258);
#13412=VERTEX_POINT('',#67259);
#13413=VERTEX_POINT('',#67261);
#13414=VERTEX_POINT('',#67273);
#13415=VERTEX_POINT('',#67284);
#13416=VERTEX_POINT('',#67285);
#13417=VERTEX_POINT('',#67322);
#13418=VERTEX_POINT('',#67323);
#13419=VERTEX_POINT('',#67359);
#13420=VERTEX_POINT('',#67360);
#13421=VERTEX_POINT('',#67396);
#13422=VERTEX_POINT('',#67397);
#13423=VERTEX_POINT('',#67434);
#13424=VERTEX_POINT('',#67435);
#13425=VERTEX_POINT('',#67471);
#13426=VERTEX_POINT('',#67472);
#13427=VERTEX_POINT('',#67508);
#13428=VERTEX_POINT('',#67509);
#13429=VERTEX_POINT('',#67546);
#13430=VERTEX_POINT('',#67547);
#13431=VERTEX_POINT('',#67582);
#13432=VERTEX_POINT('',#67583);
#13433=VERTEX_POINT('',#67620);
#13434=VERTEX_POINT('',#67621);
#13435=VERTEX_POINT('',#67657);
#13436=VERTEX_POINT('',#67658);
#13437=VERTEX_POINT('',#67694);
#13438=VERTEX_POINT('',#67695);
#13439=VERTEX_POINT('',#67732);
#13440=VERTEX_POINT('',#67733);
#13441=VERTEX_POINT('',#67774);
#13442=VERTEX_POINT('',#67775);
#13443=VERTEX_POINT('',#67779);
#13444=VERTEX_POINT('',#67781);
#13445=VERTEX_POINT('',#67792);
#13446=VERTEX_POINT('',#67796);
#13447=VERTEX_POINT('',#67807);
#13448=VERTEX_POINT('',#67811);
#13449=VERTEX_POINT('',#67822);
#13450=VERTEX_POINT('',#67826);
#13451=VERTEX_POINT('',#67837);
#13452=VERTEX_POINT('',#67841);
#13453=VERTEX_POINT('',#67852);
#13454=VERTEX_POINT('',#67856);
#13455=VERTEX_POINT('',#67867);
#13456=VERTEX_POINT('',#67871);
#13457=VERTEX_POINT('',#67894);
#13458=VERTEX_POINT('',#67895);
#13459=VERTEX_POINT('',#67899);
#13460=VERTEX_POINT('',#67901);
#13461=VERTEX_POINT('',#67912);
#13462=VERTEX_POINT('',#67916);
#13463=VERTEX_POINT('',#67927);
#13464=VERTEX_POINT('',#67931);
#13465=VERTEX_POINT('',#67942);
#13466=VERTEX_POINT('',#67946);
#13467=VERTEX_POINT('',#67957);
#13468=VERTEX_POINT('',#67961);
#13469=VERTEX_POINT('',#67972);
#13470=VERTEX_POINT('',#67976);
#13471=VERTEX_POINT('',#67987);
#13472=VERTEX_POINT('',#67991);
#13473=VERTEX_POINT('',#68002);
#13474=VERTEX_POINT('',#68006);
#13475=VERTEX_POINT('',#68029);
#13476=VERTEX_POINT('',#68030);
#13477=VERTEX_POINT('',#68034);
#13478=VERTEX_POINT('',#68036);
#13479=VERTEX_POINT('',#68047);
#13480=VERTEX_POINT('',#68051);
#13481=VERTEX_POINT('',#68062);
#13482=VERTEX_POINT('',#68066);
#13483=VERTEX_POINT('',#68077);
#13484=VERTEX_POINT('',#68081);
#13485=VERTEX_POINT('',#68092);
#13486=VERTEX_POINT('',#68096);
#13487=VERTEX_POINT('',#68107);
#13488=VERTEX_POINT('',#68111);
#13489=VERTEX_POINT('',#68122);
#13490=VERTEX_POINT('',#68126);
#13491=VERTEX_POINT('',#68137);
#13492=VERTEX_POINT('',#68141);
#13493=VERTEX_POINT('',#68152);
#13494=VERTEX_POINT('',#68156);
#13495=VERTEX_POINT('',#68167);
#13496=VERTEX_POINT('',#68171);
#13497=VERTEX_POINT('',#68182);
#13498=VERTEX_POINT('',#68186);
#13499=VERTEX_POINT('',#68197);
#13500=VERTEX_POINT('',#68201);
#13501=VERTEX_POINT('',#68212);
#13502=VERTEX_POINT('',#68216);
#13503=VERTEX_POINT('',#68227);
#13504=VERTEX_POINT('',#68231);
#13505=VERTEX_POINT('',#68242);
#13506=VERTEX_POINT('',#68246);
#13507=VERTEX_POINT('',#68265);
#13508=VERTEX_POINT('',#68266);
#13509=VERTEX_POINT('',#68268);
#13510=VERTEX_POINT('',#68270);
#13511=VERTEX_POINT('',#68274);
#13512=VERTEX_POINT('',#68276);
#13513=VERTEX_POINT('',#68280);
#13514=VERTEX_POINT('',#68282);
#13515=VERTEX_POINT('',#68295);
#13516=VERTEX_POINT('',#68296);
#13517=VERTEX_POINT('',#68300);
#13518=VERTEX_POINT('',#68302);
#13519=VERTEX_POINT('',#68313);
#13520=VERTEX_POINT('',#68317);
#13521=VERTEX_POINT('',#68328);
#13522=VERTEX_POINT('',#68332);
#13523=VERTEX_POINT('',#68343);
#13524=VERTEX_POINT('',#68347);
#13525=VERTEX_POINT('',#68358);
#13526=VERTEX_POINT('',#68362);
#13527=VERTEX_POINT('',#68373);
#13528=VERTEX_POINT('',#68377);
#13529=VERTEX_POINT('',#68388);
#13530=VERTEX_POINT('',#68392);
#13531=VERTEX_POINT('',#68415);
#13532=VERTEX_POINT('',#68416);
#13533=VERTEX_POINT('',#68420);
#13534=VERTEX_POINT('',#68422);
#13535=VERTEX_POINT('',#68433);
#13536=VERTEX_POINT('',#68437);
#13537=VERTEX_POINT('',#68448);
#13538=VERTEX_POINT('',#68452);
#13539=VERTEX_POINT('',#68463);
#13540=VERTEX_POINT('',#68467);
#13541=VERTEX_POINT('',#68478);
#13542=VERTEX_POINT('',#68482);
#13543=VERTEX_POINT('',#68493);
#13544=VERTEX_POINT('',#68497);
#13545=VERTEX_POINT('',#68508);
#13546=VERTEX_POINT('',#68512);
#13547=VERTEX_POINT('',#68523);
#13548=VERTEX_POINT('',#68527);
#13549=VERTEX_POINT('',#68550);
#13550=VERTEX_POINT('',#68551);
#13551=VERTEX_POINT('',#68555);
#13552=VERTEX_POINT('',#68557);
#13553=VERTEX_POINT('',#68568);
#13554=VERTEX_POINT('',#68572);
#13555=VERTEX_POINT('',#68583);
#13556=VERTEX_POINT('',#68587);
#13557=VERTEX_POINT('',#68598);
#13558=VERTEX_POINT('',#68602);
#13559=VERTEX_POINT('',#68613);
#13560=VERTEX_POINT('',#68617);
#13561=VERTEX_POINT('',#68628);
#13562=VERTEX_POINT('',#68632);
#13563=VERTEX_POINT('',#68643);
#13564=VERTEX_POINT('',#68647);
#13565=VERTEX_POINT('',#68658);
#13566=VERTEX_POINT('',#68662);
#13567=VERTEX_POINT('',#68673);
#13568=VERTEX_POINT('',#68677);
#13569=VERTEX_POINT('',#68688);
#13570=VERTEX_POINT('',#68692);
#13571=VERTEX_POINT('',#68703);
#13572=VERTEX_POINT('',#68707);
#13573=VERTEX_POINT('',#68718);
#13574=VERTEX_POINT('',#68722);
#13575=VERTEX_POINT('',#68733);
#13576=VERTEX_POINT('',#68737);
#13577=VERTEX_POINT('',#68748);
#13578=VERTEX_POINT('',#68752);
#13579=VERTEX_POINT('',#68763);
#13580=VERTEX_POINT('',#68767);
#13581=VERTEX_POINT('',#68863);
#13582=VERTEX_POINT('',#68865);
#13583=VERTEX_POINT('',#69698);
#13584=VERTEX_POINT('',#69787);
#13585=VERTEX_POINT('',#69790);
#13586=VERTEX_POINT('',#70633);
#13587=VERTEX_POINT('',#70638);
#13588=VERTEX_POINT('',#70639);
#13589=VERTEX_POINT('',#70641);
#13590=VERTEX_POINT('',#70643);
#13591=VERTEX_POINT('',#70645);
#13592=VERTEX_POINT('',#70647);
#13593=VERTEX_POINT('',#70652);
#13594=VERTEX_POINT('',#70653);
#13595=VERTEX_POINT('',#70657);
#13596=VERTEX_POINT('',#70661);
#13597=VERTEX_POINT('',#70665);
#13598=VERTEX_POINT('',#70669);
#13599=VERTEX_POINT('',#70673);
#13600=VERTEX_POINT('',#70676);
#13601=VERTEX_POINT('',#70697);
#17160=EDGE_CURVE('',#13378,#13379,#8006,.T.);
#17161=EDGE_CURVE('',#13378,#13380,#1483,.T.);
#17162=EDGE_CURVE('',#13380,#13381,#11126,.T.);
#17163=EDGE_CURVE('',#13381,#13379,#1484,.T.);
#17164=EDGE_CURVE('',#13382,#13383,#8007,.T.);
#17165=EDGE_CURVE('',#13382,#13378,#1485,.T.);
#17166=EDGE_CURVE('',#13379,#13383,#1486,.T.);
#17167=EDGE_CURVE('',#13384,#13385,#8008,.T.);
#17168=EDGE_CURVE('',#13384,#13382,#1487,.T.);
#17169=EDGE_CURVE('',#13383,#13385,#1488,.T.);
#17170=EDGE_CURVE('',#13386,#13387,#8009,.T.);
#17171=EDGE_CURVE('',#13386,#13384,#1489,.T.);
#17172=EDGE_CURVE('',#13385,#13387,#1490,.T.);
#17173=EDGE_CURVE('',#13388,#13389,#8010,.T.);
#17174=EDGE_CURVE('',#13388,#13386,#1491,.T.);
#17175=EDGE_CURVE('',#13387,#13389,#1492,.T.);
#17176=EDGE_CURVE('',#13390,#13391,#8011,.T.);
#17177=EDGE_CURVE('',#13390,#13388,#1493,.T.);
#17178=EDGE_CURVE('',#13389,#13391,#1494,.T.);
#17179=EDGE_CURVE('',#13392,#13393,#8012,.T.);
#17180=EDGE_CURVE('',#13392,#13390,#1495,.T.);
#17181=EDGE_CURVE('',#13391,#13393,#1496,.T.);
#17182=EDGE_CURVE('',#13394,#13395,#8013,.T.);
#17183=EDGE_CURVE('',#13394,#13392,#1497,.T.);
#17184=EDGE_CURVE('',#13393,#13395,#1498,.T.);
#17185=EDGE_CURVE('',#13396,#13397,#8014,.T.);
#17186=EDGE_CURVE('',#13396,#13394,#1499,.T.);
#17187=EDGE_CURVE('',#13395,#13397,#1500,.T.);
#17188=EDGE_CURVE('',#13398,#13399,#8015,.T.);
#17189=EDGE_CURVE('',#13398,#13396,#1501,.T.);
#17190=EDGE_CURVE('',#13397,#13399,#1502,.T.);
#17191=EDGE_CURVE('',#13400,#13401,#8016,.T.);
#17192=EDGE_CURVE('',#13400,#13398,#1503,.T.);
#17193=EDGE_CURVE('',#13399,#13401,#1504,.T.);
#17194=EDGE_CURVE('',#13402,#13403,#8017,.T.);
#17195=EDGE_CURVE('',#13402,#13400,#1505,.T.);
#17196=EDGE_CURVE('',#13401,#13403,#1506,.T.);
#17197=EDGE_CURVE('',#13404,#13405,#8018,.T.);
#17198=EDGE_CURVE('',#13404,#13402,#1507,.T.);
#17199=EDGE_CURVE('',#13403,#13405,#1508,.T.);
#17200=EDGE_CURVE('',#13406,#13407,#8019,.T.);
#17201=EDGE_CURVE('',#13406,#13404,#1509,.T.);
#17202=EDGE_CURVE('',#13405,#13407,#1510,.T.);
#17203=EDGE_CURVE('',#13408,#13409,#8020,.T.);
#17204=EDGE_CURVE('',#13410,#13408,#11127,.T.);
#17205=EDGE_CURVE('',#13410,#13406,#1511,.T.);
#17206=EDGE_CURVE('',#13407,#13409,#1512,.T.);
#17207=EDGE_CURVE('',#13411,#13412,#8021,.T.);
#17208=EDGE_CURVE('',#13411,#13413,#1513,.T.);
#17209=EDGE_CURVE('',#13414,#13413,#11128,.T.);
#17210=EDGE_CURVE('',#13412,#13414,#1514,.T.);
#17211=EDGE_CURVE('',#13415,#13416,#8022,.T.);
#17212=EDGE_CURVE('',#13415,#13411,#1515,.T.);
#17213=EDGE_CURVE('',#13416,#13412,#1516,.T.);
#17214=EDGE_CURVE('',#13417,#13418,#8023,.T.);
#17215=EDGE_CURVE('',#13417,#13415,#1517,.T.);
#17216=EDGE_CURVE('',#13418,#13416,#1518,.T.);
#17217=EDGE_CURVE('',#13419,#13420,#8024,.T.);
#17218=EDGE_CURVE('',#13419,#13417,#1519,.T.);
#17219=EDGE_CURVE('',#13420,#13418,#1520,.T.);
#17220=EDGE_CURVE('',#13421,#13422,#8025,.T.);
#17221=EDGE_CURVE('',#13421,#13419,#1521,.T.);
#17222=EDGE_CURVE('',#13422,#13420,#1522,.T.);
#17223=EDGE_CURVE('',#13423,#13424,#8026,.T.);
#17224=EDGE_CURVE('',#13423,#13421,#1523,.T.);
#17225=EDGE_CURVE('',#13424,#13422,#1524,.T.);
#17226=EDGE_CURVE('',#13425,#13426,#8027,.T.);
#17227=EDGE_CURVE('',#13425,#13423,#1525,.T.);
#17228=EDGE_CURVE('',#13426,#13424,#1526,.T.);
#17229=EDGE_CURVE('',#13427,#13428,#8028,.T.);
#17230=EDGE_CURVE('',#13427,#13425,#1527,.T.);
#17231=EDGE_CURVE('',#13428,#13426,#1528,.T.);
#17232=EDGE_CURVE('',#13429,#13430,#8029,.T.);
#17233=EDGE_CURVE('',#13429,#13427,#1529,.T.);
#17234=EDGE_CURVE('',#13430,#13428,#1530,.T.);
#17235=EDGE_CURVE('',#13431,#13432,#8030,.T.);
#17236=EDGE_CURVE('',#13431,#13429,#1531,.T.);
#17237=EDGE_CURVE('',#13432,#13430,#1532,.T.);
#17238=EDGE_CURVE('',#13433,#13434,#8031,.T.);
#17239=EDGE_CURVE('',#13433,#13431,#1533,.T.);
#17240=EDGE_CURVE('',#13434,#13432,#1534,.T.);
#17241=EDGE_CURVE('',#13435,#13436,#8032,.T.);
#17242=EDGE_CURVE('',#13435,#13433,#1535,.T.);
#17243=EDGE_CURVE('',#13436,#13434,#1536,.T.);
#17244=EDGE_CURVE('',#13437,#13438,#8033,.T.);
#17245=EDGE_CURVE('',#13437,#13435,#1537,.T.);
#17246=EDGE_CURVE('',#13438,#13436,#1538,.T.);
#17247=EDGE_CURVE('',#13439,#13440,#8034,.T.);
#17248=EDGE_CURVE('',#13439,#13437,#1539,.T.);
#17249=EDGE_CURVE('',#13440,#13438,#1540,.T.);
#17250=EDGE_CURVE('',#13441,#13442,#1541,.T.);
#17251=EDGE_CURVE('',#13441,#13443,#8035,.T.);
#17252=EDGE_CURVE('',#13443,#13444,#1542,.T.);
#17253=EDGE_CURVE('',#13442,#13444,#8036,.T.);
#17254=EDGE_CURVE('',#13445,#13441,#1543,.T.);
#17255=EDGE_CURVE('',#13445,#13446,#8037,.T.);
#17256=EDGE_CURVE('',#13446,#13443,#1544,.T.);
#17257=EDGE_CURVE('',#13447,#13445,#1545,.T.);
#17258=EDGE_CURVE('',#13447,#13448,#8038,.T.);
#17259=EDGE_CURVE('',#13448,#13446,#1546,.T.);
#17260=EDGE_CURVE('',#13449,#13447,#1547,.T.);
#17261=EDGE_CURVE('',#13449,#13450,#8039,.T.);
#17262=EDGE_CURVE('',#13450,#13448,#1548,.T.);
#17263=EDGE_CURVE('',#13451,#13449,#1549,.T.);
#17264=EDGE_CURVE('',#13451,#13452,#8040,.T.);
#17265=EDGE_CURVE('',#13452,#13450,#1550,.T.);
#17266=EDGE_CURVE('',#13453,#13451,#1551,.T.);
#17267=EDGE_CURVE('',#13453,#13454,#8041,.T.);
#17268=EDGE_CURVE('',#13454,#13452,#1552,.T.);
#17269=EDGE_CURVE('',#13455,#13453,#1553,.T.);
#17270=EDGE_CURVE('',#13455,#13456,#8042,.T.);
#17271=EDGE_CURVE('',#13456,#13454,#1554,.T.);
#17272=EDGE_CURVE('',#13442,#13455,#1555,.T.);
#17273=EDGE_CURVE('',#13444,#13456,#1556,.T.);
#17274=EDGE_CURVE('',#13457,#13458,#1557,.T.);
#17275=EDGE_CURVE('',#13457,#13459,#8043,.T.);
#17276=EDGE_CURVE('',#13459,#13460,#1558,.T.);
#17277=EDGE_CURVE('',#13458,#13460,#8044,.T.);
#17278=EDGE_CURVE('',#13461,#13457,#1559,.T.);
#17279=EDGE_CURVE('',#13461,#13462,#8045,.T.);
#17280=EDGE_CURVE('',#13462,#13459,#1560,.T.);
#17281=EDGE_CURVE('',#13463,#13461,#1561,.T.);
#17282=EDGE_CURVE('',#13463,#13464,#8046,.T.);
#17283=EDGE_CURVE('',#13464,#13462,#1562,.T.);
#17284=EDGE_CURVE('',#13465,#13463,#1563,.T.);
#17285=EDGE_CURVE('',#13465,#13466,#8047,.T.);
#17286=EDGE_CURVE('',#13466,#13464,#1564,.T.);
#17287=EDGE_CURVE('',#13467,#13465,#1565,.T.);
#17288=EDGE_CURVE('',#13467,#13468,#8048,.T.);
#17289=EDGE_CURVE('',#13468,#13466,#1566,.T.);
#17290=EDGE_CURVE('',#13469,#13467,#1567,.T.);
#17291=EDGE_CURVE('',#13469,#13470,#8049,.T.);
#17292=EDGE_CURVE('',#13470,#13468,#1568,.T.);
#17293=EDGE_CURVE('',#13471,#13469,#1569,.T.);
#17294=EDGE_CURVE('',#13471,#13472,#8050,.T.);
#17295=EDGE_CURVE('',#13472,#13470,#1570,.T.);
#17296=EDGE_CURVE('',#13473,#13471,#1571,.T.);
#17297=EDGE_CURVE('',#13473,#13474,#8051,.T.);
#17298=EDGE_CURVE('',#13474,#13472,#1572,.T.);
#17299=EDGE_CURVE('',#13458,#13473,#1573,.T.);
#17300=EDGE_CURVE('',#13460,#13474,#1574,.T.);
#17301=EDGE_CURVE('',#13475,#13476,#1575,.T.);
#17302=EDGE_CURVE('',#13475,#13477,#8052,.T.);
#17303=EDGE_CURVE('',#13477,#13478,#1576,.T.);
#17304=EDGE_CURVE('',#13476,#13478,#8053,.T.);
#17305=EDGE_CURVE('',#13479,#13475,#1577,.T.);
#17306=EDGE_CURVE('',#13479,#13480,#8054,.T.);
#17307=EDGE_CURVE('',#13480,#13477,#1578,.T.);
#17308=EDGE_CURVE('',#13481,#13479,#1579,.T.);
#17309=EDGE_CURVE('',#13481,#13482,#8055,.T.);
#17310=EDGE_CURVE('',#13482,#13480,#1580,.T.);
#17311=EDGE_CURVE('',#13483,#13481,#1581,.T.);
#17312=EDGE_CURVE('',#13483,#13484,#8056,.T.);
#17313=EDGE_CURVE('',#13484,#13482,#1582,.T.);
#17314=EDGE_CURVE('',#13485,#13483,#1583,.T.);
#17315=EDGE_CURVE('',#13485,#13486,#8057,.T.);
#17316=EDGE_CURVE('',#13486,#13484,#1584,.T.);
#17317=EDGE_CURVE('',#13487,#13485,#1585,.T.);
#17318=EDGE_CURVE('',#13487,#13488,#8058,.T.);
#17319=EDGE_CURVE('',#13488,#13486,#1586,.T.);
#17320=EDGE_CURVE('',#13489,#13487,#1587,.T.);
#17321=EDGE_CURVE('',#13489,#13490,#8059,.T.);
#17322=EDGE_CURVE('',#13490,#13488,#1588,.T.);
#17323=EDGE_CURVE('',#13491,#13489,#1589,.T.);
#17324=EDGE_CURVE('',#13491,#13492,#8060,.T.);
#17325=EDGE_CURVE('',#13492,#13490,#1590,.T.);
#17326=EDGE_CURVE('',#13493,#13491,#1591,.T.);
#17327=EDGE_CURVE('',#13493,#13494,#8061,.T.);
#17328=EDGE_CURVE('',#13494,#13492,#1592,.T.);
#17329=EDGE_CURVE('',#13495,#13493,#1593,.T.);
#17330=EDGE_CURVE('',#13495,#13496,#8062,.T.);
#17331=EDGE_CURVE('',#13496,#13494,#1594,.T.);
#17332=EDGE_CURVE('',#13497,#13495,#1595,.T.);
#17333=EDGE_CURVE('',#13497,#13498,#8063,.T.);
#17334=EDGE_CURVE('',#13498,#13496,#1596,.T.);
#17335=EDGE_CURVE('',#13499,#13497,#1597,.T.);
#17336=EDGE_CURVE('',#13499,#13500,#8064,.T.);
#17337=EDGE_CURVE('',#13500,#13498,#1598,.T.);
#17338=EDGE_CURVE('',#13501,#13499,#1599,.T.);
#17339=EDGE_CURVE('',#13501,#13502,#8065,.T.);
#17340=EDGE_CURVE('',#13502,#13500,#1600,.T.);
#17341=EDGE_CURVE('',#13503,#13501,#1601,.T.);
#17342=EDGE_CURVE('',#13503,#13504,#8066,.T.);
#17343=EDGE_CURVE('',#13504,#13502,#1602,.T.);
#17344=EDGE_CURVE('',#13505,#13503,#1603,.T.);
#17345=EDGE_CURVE('',#13505,#13506,#8067,.T.);
#17346=EDGE_CURVE('',#13506,#13504,#1604,.T.);
#17347=EDGE_CURVE('',#13476,#13505,#1605,.T.);
#17348=EDGE_CURVE('',#13478,#13506,#1606,.T.);
#17349=EDGE_CURVE('',#13507,#13508,#8068,.T.);
#17350=EDGE_CURVE('',#13507,#13509,#8069,.T.);
#17351=EDGE_CURVE('',#13509,#13510,#8070,.T.);
#17352=EDGE_CURVE('',#13508,#13510,#8071,.T.);
#17353=EDGE_CURVE('',#13511,#13507,#8072,.T.);
#17354=EDGE_CURVE('',#13511,#13512,#8073,.T.);
#17355=EDGE_CURVE('',#13512,#13509,#8074,.T.);
#17356=EDGE_CURVE('',#13513,#13511,#8075,.T.);
#17357=EDGE_CURVE('',#13513,#13514,#8076,.T.);
#17358=EDGE_CURVE('',#13514,#13512,#8077,.T.);
#17359=EDGE_CURVE('',#13508,#13513,#8078,.T.);
#17360=EDGE_CURVE('',#13510,#13514,#8079,.T.);
#17361=EDGE_CURVE('',#13515,#13516,#1607,.T.);
#17362=EDGE_CURVE('',#13515,#13517,#8080,.T.);
#17363=EDGE_CURVE('',#13517,#13518,#1608,.T.);
#17364=EDGE_CURVE('',#13516,#13518,#8081,.T.);
#17365=EDGE_CURVE('',#13519,#13515,#1609,.T.);
#17366=EDGE_CURVE('',#13519,#13520,#8082,.T.);
#17367=EDGE_CURVE('',#13520,#13517,#1610,.T.);
#17368=EDGE_CURVE('',#13521,#13519,#1611,.T.);
#17369=EDGE_CURVE('',#13521,#13522,#8083,.T.);
#17370=EDGE_CURVE('',#13522,#13520,#1612,.T.);
#17371=EDGE_CURVE('',#13523,#13521,#1613,.T.);
#17372=EDGE_CURVE('',#13523,#13524,#8084,.T.);
#17373=EDGE_CURVE('',#13524,#13522,#1614,.T.);
#17374=EDGE_CURVE('',#13525,#13523,#1615,.T.);
#17375=EDGE_CURVE('',#13525,#13526,#8085,.T.);
#17376=EDGE_CURVE('',#13526,#13524,#1616,.T.);
#17377=EDGE_CURVE('',#13527,#13525,#1617,.T.);
#17378=EDGE_CURVE('',#13527,#13528,#8086,.T.);
#17379=EDGE_CURVE('',#13528,#13526,#1618,.T.);
#17380=EDGE_CURVE('',#13529,#13527,#1619,.T.);
#17381=EDGE_CURVE('',#13529,#13530,#8087,.T.);
#17382=EDGE_CURVE('',#13530,#13528,#1620,.T.);
#17383=EDGE_CURVE('',#13516,#13529,#1621,.T.);
#17384=EDGE_CURVE('',#13518,#13530,#1622,.T.);
#17385=EDGE_CURVE('',#13531,#13532,#1623,.T.);
#17386=EDGE_CURVE('',#13531,#13533,#8088,.T.);
#17387=EDGE_CURVE('',#13533,#13534,#1624,.T.);
#17388=EDGE_CURVE('',#13532,#13534,#8089,.T.);
#17389=EDGE_CURVE('',#13535,#13531,#1625,.T.);
#17390=EDGE_CURVE('',#13535,#13536,#8090,.T.);
#17391=EDGE_CURVE('',#13536,#13533,#1626,.T.);
#17392=EDGE_CURVE('',#13537,#13535,#1627,.T.);
#17393=EDGE_CURVE('',#13537,#13538,#8091,.T.);
#17394=EDGE_CURVE('',#13538,#13536,#1628,.T.);
#17395=EDGE_CURVE('',#13539,#13537,#1629,.T.);
#17396=EDGE_CURVE('',#13539,#13540,#8092,.T.);
#17397=EDGE_CURVE('',#13540,#13538,#1630,.T.);
#17398=EDGE_CURVE('',#13541,#13539,#1631,.T.);
#17399=EDGE_CURVE('',#13541,#13542,#8093,.T.);
#17400=EDGE_CURVE('',#13542,#13540,#1632,.T.);
#17401=EDGE_CURVE('',#13543,#13541,#1633,.T.);
#17402=EDGE_CURVE('',#13543,#13544,#8094,.T.);
#17403=EDGE_CURVE('',#13544,#13542,#1634,.T.);
#17404=EDGE_CURVE('',#13545,#13543,#1635,.T.);
#17405=EDGE_CURVE('',#13545,#13546,#8095,.T.);
#17406=EDGE_CURVE('',#13546,#13544,#1636,.T.);
#17407=EDGE_CURVE('',#13547,#13545,#1637,.T.);
#17408=EDGE_CURVE('',#13547,#13548,#8096,.T.);
#17409=EDGE_CURVE('',#13548,#13546,#1638,.T.);
#17410=EDGE_CURVE('',#13532,#13547,#1639,.T.);
#17411=EDGE_CURVE('',#13534,#13548,#1640,.T.);
#17412=EDGE_CURVE('',#13549,#13550,#1641,.T.);
#17413=EDGE_CURVE('',#13549,#13551,#8097,.T.);
#17414=EDGE_CURVE('',#13551,#13552,#1642,.T.);
#17415=EDGE_CURVE('',#13550,#13552,#8098,.T.);
#17416=EDGE_CURVE('',#13553,#13549,#1643,.T.);
#17417=EDGE_CURVE('',#13553,#13554,#8099,.T.);
#17418=EDGE_CURVE('',#13554,#13551,#1644,.T.);
#17419=EDGE_CURVE('',#13555,#13553,#1645,.T.);
#17420=EDGE_CURVE('',#13555,#13556,#8100,.T.);
#17421=EDGE_CURVE('',#13556,#13554,#1646,.T.);
#17422=EDGE_CURVE('',#13557,#13555,#1647,.T.);
#17423=EDGE_CURVE('',#13557,#13558,#8101,.T.);
#17424=EDGE_CURVE('',#13558,#13556,#1648,.T.);
#17425=EDGE_CURVE('',#13559,#13557,#1649,.T.);
#17426=EDGE_CURVE('',#13559,#13560,#8102,.T.);
#17427=EDGE_CURVE('',#13560,#13558,#1650,.T.);
#17428=EDGE_CURVE('',#13561,#13559,#1651,.T.);
#17429=EDGE_CURVE('',#13561,#13562,#8103,.T.);
#17430=EDGE_CURVE('',#13562,#13560,#1652,.T.);
#17431=EDGE_CURVE('',#13563,#13561,#1653,.T.);
#17432=EDGE_CURVE('',#13563,#13564,#8104,.T.);
#17433=EDGE_CURVE('',#13564,#13562,#1654,.T.);
#17434=EDGE_CURVE('',#13565,#13563,#1655,.T.);
#17435=EDGE_CURVE('',#13565,#13566,#8105,.T.);
#17436=EDGE_CURVE('',#13566,#13564,#1656,.T.);
#17437=EDGE_CURVE('',#13567,#13565,#1657,.T.);
#17438=EDGE_CURVE('',#13567,#13568,#8106,.T.);
#17439=EDGE_CURVE('',#13568,#13566,#1658,.T.);
#17440=EDGE_CURVE('',#13569,#13567,#1659,.T.);
#17441=EDGE_CURVE('',#13569,#13570,#8107,.T.);
#17442=EDGE_CURVE('',#13570,#13568,#1660,.T.);
#17443=EDGE_CURVE('',#13571,#13569,#1661,.T.);
#17444=EDGE_CURVE('',#13571,#13572,#8108,.T.);
#17445=EDGE_CURVE('',#13572,#13570,#1662,.T.);
#17446=EDGE_CURVE('',#13573,#13571,#1663,.T.);
#17447=EDGE_CURVE('',#13573,#13574,#8109,.T.);
#17448=EDGE_CURVE('',#13574,#13572,#1664,.T.);
#17449=EDGE_CURVE('',#13575,#13573,#1665,.T.);
#17450=EDGE_CURVE('',#13575,#13576,#8110,.T.);
#17451=EDGE_CURVE('',#13576,#13574,#1666,.T.);
#17452=EDGE_CURVE('',#13577,#13575,#1667,.T.);
#17453=EDGE_CURVE('',#13577,#13578,#8111,.T.);
#17454=EDGE_CURVE('',#13578,#13576,#1668,.T.);
#17455=EDGE_CURVE('',#13579,#13577,#1669,.T.);
#17456=EDGE_CURVE('',#13579,#13580,#8112,.T.);
#17457=EDGE_CURVE('',#13580,#13578,#1670,.T.);
#17458=EDGE_CURVE('',#13550,#13579,#1671,.T.);
#17459=EDGE_CURVE('',#13552,#13580,#1672,.T.);
#17460=EDGE_CURVE('',#13413,#13410,#1673,.T.);
#17461=EDGE_CURVE('',#13581,#13410,#11129,.T.);
#17462=EDGE_CURVE('',#13582,#13581,#11130,.T.);
#17463=EDGE_CURVE('',#13582,#13414,#1674,.T.);
#17464=EDGE_CURVE('',#13409,#13582,#1675,.T.);
#17465=EDGE_CURVE('',#13583,#13381,#1676,.T.);
#17466=EDGE_CURVE('',#13583,#13440,#1677,.T.);
#17467=EDGE_CURVE('',#13381,#13584,#11131,.T.);
#17468=EDGE_CURVE('',#13584,#13380,#11132,.T.);
#17469=EDGE_CURVE('',#13380,#13585,#1678,.T.);
#17470=EDGE_CURVE('',#13585,#13583,#11133,.T.);
#17471=EDGE_CURVE('',#13585,#13439,#1679,.T.);
#17472=EDGE_CURVE('',#13586,#13586,#11134,.T.);
#17473=EDGE_CURVE('',#13586,#13581,#11135,.T.);
#17474=EDGE_CURVE('',#13408,#13582,#11136,.T.);
#17475=EDGE_CURVE('',#13587,#13588,#8113,.T.);
#17476=EDGE_CURVE('',#13589,#13587,#8114,.T.);
#17477=EDGE_CURVE('',#13590,#13589,#8115,.T.);
#17478=EDGE_CURVE('',#13591,#13590,#8116,.T.);
#17479=EDGE_CURVE('',#13592,#13591,#8117,.T.);
#17480=EDGE_CURVE('',#13588,#13592,#8118,.T.);
#17481=EDGE_CURVE('',#13593,#13594,#263,.T.);
#17482=EDGE_CURVE('',#13595,#13593,#264,.T.);
#17483=EDGE_CURVE('',#13596,#13595,#265,.T.);
#17484=EDGE_CURVE('',#13597,#13596,#266,.T.);
#17485=EDGE_CURVE('',#13598,#13597,#267,.T.);
#17486=EDGE_CURVE('',#13598,#13599,#8119,.T.);
#17487=EDGE_CURVE('',#13599,#13599,#11137,.T.);
#17488=EDGE_CURVE('',#13600,#13598,#268,.T.);
#17489=EDGE_CURVE('',#13594,#13600,#269,.T.);
#17490=EDGE_CURVE('',#13592,#13596,#8120,.T.);
#17491=EDGE_CURVE('',#13591,#13597,#8121,.T.);
#17492=EDGE_CURVE('',#13588,#13595,#8122,.T.);
#17493=EDGE_CURVE('',#13587,#13593,#8123,.T.);
#17494=EDGE_CURVE('',#13589,#13594,#8124,.T.);
#17495=EDGE_CURVE('',#13590,#13600,#8125,.T.);
#17496=EDGE_CURVE('',#13601,#13601,#11138,.T.);
#17497=EDGE_CURVE('',#13584,#13601,#8126,.T.);
#24614=ORIENTED_EDGE('',*,*,#17160,.F.);
#24615=ORIENTED_EDGE('',*,*,#17161,.T.);
#24616=ORIENTED_EDGE('',*,*,#17162,.T.);
#24617=ORIENTED_EDGE('',*,*,#17163,.T.);
#24618=ORIENTED_EDGE('',*,*,#17164,.F.);
#24619=ORIENTED_EDGE('',*,*,#17165,.T.);
#24620=ORIENTED_EDGE('',*,*,#17160,.T.);
#24621=ORIENTED_EDGE('',*,*,#17166,.T.);
#24622=ORIENTED_EDGE('',*,*,#17167,.F.);
#24623=ORIENTED_EDGE('',*,*,#17168,.T.);
#24624=ORIENTED_EDGE('',*,*,#17164,.T.);
#24625=ORIENTED_EDGE('',*,*,#17169,.T.);
#24626=ORIENTED_EDGE('',*,*,#17170,.F.);
#24627=ORIENTED_EDGE('',*,*,#17171,.T.);
#24628=ORIENTED_EDGE('',*,*,#17167,.T.);
#24629=ORIENTED_EDGE('',*,*,#17172,.T.);
#24630=ORIENTED_EDGE('',*,*,#17173,.F.);
#24631=ORIENTED_EDGE('',*,*,#17174,.T.);
#24632=ORIENTED_EDGE('',*,*,#17170,.T.);
#24633=ORIENTED_EDGE('',*,*,#17175,.T.);
#24634=ORIENTED_EDGE('',*,*,#17176,.F.);
#24635=ORIENTED_EDGE('',*,*,#17177,.T.);
#24636=ORIENTED_EDGE('',*,*,#17173,.T.);
#24637=ORIENTED_EDGE('',*,*,#17178,.T.);
#24638=ORIENTED_EDGE('',*,*,#17179,.F.);
#24639=ORIENTED_EDGE('',*,*,#17180,.T.);
#24640=ORIENTED_EDGE('',*,*,#17176,.T.);
#24641=ORIENTED_EDGE('',*,*,#17181,.T.);
#24642=ORIENTED_EDGE('',*,*,#17182,.F.);
#24643=ORIENTED_EDGE('',*,*,#17183,.T.);
#24644=ORIENTED_EDGE('',*,*,#17179,.T.);
#24645=ORIENTED_EDGE('',*,*,#17184,.T.);
#24646=ORIENTED_EDGE('',*,*,#17185,.F.);
#24647=ORIENTED_EDGE('',*,*,#17186,.T.);
#24648=ORIENTED_EDGE('',*,*,#17182,.T.);
#24649=ORIENTED_EDGE('',*,*,#17187,.T.);
#24650=ORIENTED_EDGE('',*,*,#17188,.F.);
#24651=ORIENTED_EDGE('',*,*,#17189,.T.);
#24652=ORIENTED_EDGE('',*,*,#17185,.T.);
#24653=ORIENTED_EDGE('',*,*,#17190,.T.);
#24654=ORIENTED_EDGE('',*,*,#17191,.F.);
#24655=ORIENTED_EDGE('',*,*,#17192,.T.);
#24656=ORIENTED_EDGE('',*,*,#17188,.T.);
#24657=ORIENTED_EDGE('',*,*,#17193,.T.);
#24658=ORIENTED_EDGE('',*,*,#17194,.F.);
#24659=ORIENTED_EDGE('',*,*,#17195,.T.);
#24660=ORIENTED_EDGE('',*,*,#17191,.T.);
#24661=ORIENTED_EDGE('',*,*,#17196,.T.);
#24662=ORIENTED_EDGE('',*,*,#17197,.F.);
#24663=ORIENTED_EDGE('',*,*,#17198,.T.);
#24664=ORIENTED_EDGE('',*,*,#17194,.T.);
#24665=ORIENTED_EDGE('',*,*,#17199,.T.);
#24666=ORIENTED_EDGE('',*,*,#17200,.F.);
#24667=ORIENTED_EDGE('',*,*,#17201,.T.);
#24668=ORIENTED_EDGE('',*,*,#17197,.T.);
#24669=ORIENTED_EDGE('',*,*,#17202,.T.);
#24670=ORIENTED_EDGE('',*,*,#17203,.F.);
#24671=ORIENTED_EDGE('',*,*,#17204,.F.);
#24672=ORIENTED_EDGE('',*,*,#17205,.T.);
#24673=ORIENTED_EDGE('',*,*,#17200,.T.);
#24674=ORIENTED_EDGE('',*,*,#17206,.T.);
#24675=ORIENTED_EDGE('',*,*,#17207,.F.);
#24676=ORIENTED_EDGE('',*,*,#17208,.T.);
#24677=ORIENTED_EDGE('',*,*,#17209,.F.);
#24678=ORIENTED_EDGE('',*,*,#17210,.F.);
#24679=ORIENTED_EDGE('',*,*,#17211,.F.);
#24680=ORIENTED_EDGE('',*,*,#17212,.T.);
#24681=ORIENTED_EDGE('',*,*,#17207,.T.);
#24682=ORIENTED_EDGE('',*,*,#17213,.F.);
#24683=ORIENTED_EDGE('',*,*,#17214,.F.);
#24684=ORIENTED_EDGE('',*,*,#17215,.T.);
#24685=ORIENTED_EDGE('',*,*,#17211,.T.);
#24686=ORIENTED_EDGE('',*,*,#17216,.F.);
#24687=ORIENTED_EDGE('',*,*,#17217,.F.);
#24688=ORIENTED_EDGE('',*,*,#17218,.T.);
#24689=ORIENTED_EDGE('',*,*,#17214,.T.);
#24690=ORIENTED_EDGE('',*,*,#17219,.F.);
#24691=ORIENTED_EDGE('',*,*,#17220,.F.);
#24692=ORIENTED_EDGE('',*,*,#17221,.T.);
#24693=ORIENTED_EDGE('',*,*,#17217,.T.);
#24694=ORIENTED_EDGE('',*,*,#17222,.F.);
#24695=ORIENTED_EDGE('',*,*,#17223,.F.);
#24696=ORIENTED_EDGE('',*,*,#17224,.T.);
#24697=ORIENTED_EDGE('',*,*,#17220,.T.);
#24698=ORIENTED_EDGE('',*,*,#17225,.F.);
#24699=ORIENTED_EDGE('',*,*,#17226,.F.);
#24700=ORIENTED_EDGE('',*,*,#17227,.T.);
#24701=ORIENTED_EDGE('',*,*,#17223,.T.);
#24702=ORIENTED_EDGE('',*,*,#17228,.F.);
#24703=ORIENTED_EDGE('',*,*,#17229,.F.);
#24704=ORIENTED_EDGE('',*,*,#17230,.T.);
#24705=ORIENTED_EDGE('',*,*,#17226,.T.);
#24706=ORIENTED_EDGE('',*,*,#17231,.F.);
#24707=ORIENTED_EDGE('',*,*,#17232,.F.);
#24708=ORIENTED_EDGE('',*,*,#17233,.T.);
#24709=ORIENTED_EDGE('',*,*,#17229,.T.);
#24710=ORIENTED_EDGE('',*,*,#17234,.F.);
#24711=ORIENTED_EDGE('',*,*,#17235,.F.);
#24712=ORIENTED_EDGE('',*,*,#17236,.T.);
#24713=ORIENTED_EDGE('',*,*,#17232,.T.);
#24714=ORIENTED_EDGE('',*,*,#17237,.F.);
#24715=ORIENTED_EDGE('',*,*,#17238,.F.);
#24716=ORIENTED_EDGE('',*,*,#17239,.T.);
#24717=ORIENTED_EDGE('',*,*,#17235,.T.);
#24718=ORIENTED_EDGE('',*,*,#17240,.F.);
#24719=ORIENTED_EDGE('',*,*,#17241,.F.);
#24720=ORIENTED_EDGE('',*,*,#17242,.T.);
#24721=ORIENTED_EDGE('',*,*,#17238,.T.);
#24722=ORIENTED_EDGE('',*,*,#17243,.F.);
#24723=ORIENTED_EDGE('',*,*,#17244,.F.);
#24724=ORIENTED_EDGE('',*,*,#17245,.T.);
#24725=ORIENTED_EDGE('',*,*,#17241,.T.);
#24726=ORIENTED_EDGE('',*,*,#17246,.F.);
#24727=ORIENTED_EDGE('',*,*,#17247,.F.);
#24728=ORIENTED_EDGE('',*,*,#17248,.T.);
#24729=ORIENTED_EDGE('',*,*,#17244,.T.);
#24730=ORIENTED_EDGE('',*,*,#17249,.F.);
#24731=ORIENTED_EDGE('',*,*,#17250,.F.);
#24732=ORIENTED_EDGE('',*,*,#17251,.T.);
#24733=ORIENTED_EDGE('',*,*,#17252,.T.);
#24734=ORIENTED_EDGE('',*,*,#17253,.F.);
#24735=ORIENTED_EDGE('',*,*,#17254,.F.);
#24736=ORIENTED_EDGE('',*,*,#17255,.T.);
#24737=ORIENTED_EDGE('',*,*,#17256,.T.);
#24738=ORIENTED_EDGE('',*,*,#17251,.F.);
#24739=ORIENTED_EDGE('',*,*,#17257,.F.);
#24740=ORIENTED_EDGE('',*,*,#17258,.T.);
#24741=ORIENTED_EDGE('',*,*,#17259,.T.);
#24742=ORIENTED_EDGE('',*,*,#17255,.F.);
#24743=ORIENTED_EDGE('',*,*,#17260,.F.);
#24744=ORIENTED_EDGE('',*,*,#17261,.T.);
#24745=ORIENTED_EDGE('',*,*,#17262,.T.);
#24746=ORIENTED_EDGE('',*,*,#17258,.F.);
#24747=ORIENTED_EDGE('',*,*,#17263,.F.);
#24748=ORIENTED_EDGE('',*,*,#17264,.T.);
#24749=ORIENTED_EDGE('',*,*,#17265,.T.);
#24750=ORIENTED_EDGE('',*,*,#17261,.F.);
#24751=ORIENTED_EDGE('',*,*,#17266,.F.);
#24752=ORIENTED_EDGE('',*,*,#17267,.T.);
#24753=ORIENTED_EDGE('',*,*,#17268,.T.);
#24754=ORIENTED_EDGE('',*,*,#17264,.F.);
#24755=ORIENTED_EDGE('',*,*,#17269,.F.);
#24756=ORIENTED_EDGE('',*,*,#17270,.T.);
#24757=ORIENTED_EDGE('',*,*,#17271,.T.);
#24758=ORIENTED_EDGE('',*,*,#17267,.F.);
#24759=ORIENTED_EDGE('',*,*,#17272,.F.);
#24760=ORIENTED_EDGE('',*,*,#17253,.T.);
#24761=ORIENTED_EDGE('',*,*,#17273,.T.);
#24762=ORIENTED_EDGE('',*,*,#17270,.F.);
#24763=ORIENTED_EDGE('',*,*,#17274,.F.);
#24764=ORIENTED_EDGE('',*,*,#17275,.T.);
#24765=ORIENTED_EDGE('',*,*,#17276,.T.);
#24766=ORIENTED_EDGE('',*,*,#17277,.F.);
#24767=ORIENTED_EDGE('',*,*,#17278,.F.);
#24768=ORIENTED_EDGE('',*,*,#17279,.T.);
#24769=ORIENTED_EDGE('',*,*,#17280,.T.);
#24770=ORIENTED_EDGE('',*,*,#17275,.F.);
#24771=ORIENTED_EDGE('',*,*,#17281,.F.);
#24772=ORIENTED_EDGE('',*,*,#17282,.T.);
#24773=ORIENTED_EDGE('',*,*,#17283,.T.);
#24774=ORIENTED_EDGE('',*,*,#17279,.F.);
#24775=ORIENTED_EDGE('',*,*,#17284,.F.);
#24776=ORIENTED_EDGE('',*,*,#17285,.T.);
#24777=ORIENTED_EDGE('',*,*,#17286,.T.);
#24778=ORIENTED_EDGE('',*,*,#17282,.F.);
#24779=ORIENTED_EDGE('',*,*,#17287,.F.);
#24780=ORIENTED_EDGE('',*,*,#17288,.T.);
#24781=ORIENTED_EDGE('',*,*,#17289,.T.);
#24782=ORIENTED_EDGE('',*,*,#17285,.F.);
#24783=ORIENTED_EDGE('',*,*,#17290,.F.);
#24784=ORIENTED_EDGE('',*,*,#17291,.T.);
#24785=ORIENTED_EDGE('',*,*,#17292,.T.);
#24786=ORIENTED_EDGE('',*,*,#17288,.F.);
#24787=ORIENTED_EDGE('',*,*,#17293,.F.);
#24788=ORIENTED_EDGE('',*,*,#17294,.T.);
#24789=ORIENTED_EDGE('',*,*,#17295,.T.);
#24790=ORIENTED_EDGE('',*,*,#17291,.F.);
#24791=ORIENTED_EDGE('',*,*,#17296,.F.);
#24792=ORIENTED_EDGE('',*,*,#17297,.T.);
#24793=ORIENTED_EDGE('',*,*,#17298,.T.);
#24794=ORIENTED_EDGE('',*,*,#17294,.F.);
#24795=ORIENTED_EDGE('',*,*,#17299,.F.);
#24796=ORIENTED_EDGE('',*,*,#17277,.T.);
#24797=ORIENTED_EDGE('',*,*,#17300,.T.);
#24798=ORIENTED_EDGE('',*,*,#17297,.F.);
#24799=ORIENTED_EDGE('',*,*,#17301,.F.);
#24800=ORIENTED_EDGE('',*,*,#17302,.T.);
#24801=ORIENTED_EDGE('',*,*,#17303,.T.);
#24802=ORIENTED_EDGE('',*,*,#17304,.F.);
#24803=ORIENTED_EDGE('',*,*,#17305,.F.);
#24804=ORIENTED_EDGE('',*,*,#17306,.T.);
#24805=ORIENTED_EDGE('',*,*,#17307,.T.);
#24806=ORIENTED_EDGE('',*,*,#17302,.F.);
#24807=ORIENTED_EDGE('',*,*,#17308,.F.);
#24808=ORIENTED_EDGE('',*,*,#17309,.T.);
#24809=ORIENTED_EDGE('',*,*,#17310,.T.);
#24810=ORIENTED_EDGE('',*,*,#17306,.F.);
#24811=ORIENTED_EDGE('',*,*,#17311,.F.);
#24812=ORIENTED_EDGE('',*,*,#17312,.T.);
#24813=ORIENTED_EDGE('',*,*,#17313,.T.);
#24814=ORIENTED_EDGE('',*,*,#17309,.F.);
#24815=ORIENTED_EDGE('',*,*,#17314,.F.);
#24816=ORIENTED_EDGE('',*,*,#17315,.T.);
#24817=ORIENTED_EDGE('',*,*,#17316,.T.);
#24818=ORIENTED_EDGE('',*,*,#17312,.F.);
#24819=ORIENTED_EDGE('',*,*,#17317,.F.);
#24820=ORIENTED_EDGE('',*,*,#17318,.T.);
#24821=ORIENTED_EDGE('',*,*,#17319,.T.);
#24822=ORIENTED_EDGE('',*,*,#17315,.F.);
#24823=ORIENTED_EDGE('',*,*,#17320,.F.);
#24824=ORIENTED_EDGE('',*,*,#17321,.T.);
#24825=ORIENTED_EDGE('',*,*,#17322,.T.);
#24826=ORIENTED_EDGE('',*,*,#17318,.F.);
#24827=ORIENTED_EDGE('',*,*,#17323,.F.);
#24828=ORIENTED_EDGE('',*,*,#17324,.T.);
#24829=ORIENTED_EDGE('',*,*,#17325,.T.);
#24830=ORIENTED_EDGE('',*,*,#17321,.F.);
#24831=ORIENTED_EDGE('',*,*,#17326,.F.);
#24832=ORIENTED_EDGE('',*,*,#17327,.T.);
#24833=ORIENTED_EDGE('',*,*,#17328,.T.);
#24834=ORIENTED_EDGE('',*,*,#17324,.F.);
#24835=ORIENTED_EDGE('',*,*,#17329,.F.);
#24836=ORIENTED_EDGE('',*,*,#17330,.T.);
#24837=ORIENTED_EDGE('',*,*,#17331,.T.);
#24838=ORIENTED_EDGE('',*,*,#17327,.F.);
#24839=ORIENTED_EDGE('',*,*,#17332,.F.);
#24840=ORIENTED_EDGE('',*,*,#17333,.T.);
#24841=ORIENTED_EDGE('',*,*,#17334,.T.);
#24842=ORIENTED_EDGE('',*,*,#17330,.F.);
#24843=ORIENTED_EDGE('',*,*,#17335,.F.);
#24844=ORIENTED_EDGE('',*,*,#17336,.T.);
#24845=ORIENTED_EDGE('',*,*,#17337,.T.);
#24846=ORIENTED_EDGE('',*,*,#17333,.F.);
#24847=ORIENTED_EDGE('',*,*,#17338,.F.);
#24848=ORIENTED_EDGE('',*,*,#17339,.T.);
#24849=ORIENTED_EDGE('',*,*,#17340,.T.);
#24850=ORIENTED_EDGE('',*,*,#17336,.F.);
#24851=ORIENTED_EDGE('',*,*,#17341,.F.);
#24852=ORIENTED_EDGE('',*,*,#17342,.T.);
#24853=ORIENTED_EDGE('',*,*,#17343,.T.);
#24854=ORIENTED_EDGE('',*,*,#17339,.F.);
#24855=ORIENTED_EDGE('',*,*,#17344,.F.);
#24856=ORIENTED_EDGE('',*,*,#17345,.T.);
#24857=ORIENTED_EDGE('',*,*,#17346,.T.);
#24858=ORIENTED_EDGE('',*,*,#17342,.F.);
#24859=ORIENTED_EDGE('',*,*,#17347,.F.);
#24860=ORIENTED_EDGE('',*,*,#17304,.T.);
#24861=ORIENTED_EDGE('',*,*,#17348,.T.);
#24862=ORIENTED_EDGE('',*,*,#17345,.F.);
#24863=ORIENTED_EDGE('',*,*,#17348,.F.);
#24864=ORIENTED_EDGE('',*,*,#17303,.F.);
#24865=ORIENTED_EDGE('',*,*,#17307,.F.);
#24866=ORIENTED_EDGE('',*,*,#17310,.F.);
#24867=ORIENTED_EDGE('',*,*,#17313,.F.);
#24868=ORIENTED_EDGE('',*,*,#17316,.F.);
#24869=ORIENTED_EDGE('',*,*,#17319,.F.);
#24870=ORIENTED_EDGE('',*,*,#17322,.F.);
#24871=ORIENTED_EDGE('',*,*,#17325,.F.);
#24872=ORIENTED_EDGE('',*,*,#17328,.F.);
#24873=ORIENTED_EDGE('',*,*,#17331,.F.);
#24874=ORIENTED_EDGE('',*,*,#17334,.F.);
#24875=ORIENTED_EDGE('',*,*,#17337,.F.);
#24876=ORIENTED_EDGE('',*,*,#17340,.F.);
#24877=ORIENTED_EDGE('',*,*,#17343,.F.);
#24878=ORIENTED_EDGE('',*,*,#17346,.F.);
#24879=ORIENTED_EDGE('',*,*,#17300,.F.);
#24880=ORIENTED_EDGE('',*,*,#17276,.F.);
#24881=ORIENTED_EDGE('',*,*,#17280,.F.);
#24882=ORIENTED_EDGE('',*,*,#17283,.F.);
#24883=ORIENTED_EDGE('',*,*,#17286,.F.);
#24884=ORIENTED_EDGE('',*,*,#17289,.F.);
#24885=ORIENTED_EDGE('',*,*,#17292,.F.);
#24886=ORIENTED_EDGE('',*,*,#17295,.F.);
#24887=ORIENTED_EDGE('',*,*,#17298,.F.);
#24888=ORIENTED_EDGE('',*,*,#17273,.F.);
#24889=ORIENTED_EDGE('',*,*,#17252,.F.);
#24890=ORIENTED_EDGE('',*,*,#17256,.F.);
#24891=ORIENTED_EDGE('',*,*,#17259,.F.);
#24892=ORIENTED_EDGE('',*,*,#17262,.F.);
#24893=ORIENTED_EDGE('',*,*,#17265,.F.);
#24894=ORIENTED_EDGE('',*,*,#17268,.F.);
#24895=ORIENTED_EDGE('',*,*,#17271,.F.);
#24896=ORIENTED_EDGE('',*,*,#17349,.F.);
#24897=ORIENTED_EDGE('',*,*,#17350,.T.);
#24898=ORIENTED_EDGE('',*,*,#17351,.T.);
#24899=ORIENTED_EDGE('',*,*,#17352,.F.);
#24900=ORIENTED_EDGE('',*,*,#17353,.F.);
#24901=ORIENTED_EDGE('',*,*,#17354,.T.);
#24902=ORIENTED_EDGE('',*,*,#17355,.T.);
#24903=ORIENTED_EDGE('',*,*,#17350,.F.);
#24904=ORIENTED_EDGE('',*,*,#17356,.F.);
#24905=ORIENTED_EDGE('',*,*,#17357,.T.);
#24906=ORIENTED_EDGE('',*,*,#17358,.T.);
#24907=ORIENTED_EDGE('',*,*,#17354,.F.);
#24908=ORIENTED_EDGE('',*,*,#17359,.F.);
#24909=ORIENTED_EDGE('',*,*,#17352,.T.);
#24910=ORIENTED_EDGE('',*,*,#17360,.T.);
#24911=ORIENTED_EDGE('',*,*,#17357,.F.);
#24912=ORIENTED_EDGE('',*,*,#17360,.F.);
#24913=ORIENTED_EDGE('',*,*,#17351,.F.);
#24914=ORIENTED_EDGE('',*,*,#17355,.F.);
#24915=ORIENTED_EDGE('',*,*,#17358,.F.);
#24916=ORIENTED_EDGE('',*,*,#17361,.F.);
#24917=ORIENTED_EDGE('',*,*,#17362,.T.);
#24918=ORIENTED_EDGE('',*,*,#17363,.T.);
#24919=ORIENTED_EDGE('',*,*,#17364,.F.);
#24920=ORIENTED_EDGE('',*,*,#17365,.F.);
#24921=ORIENTED_EDGE('',*,*,#17366,.T.);
#24922=ORIENTED_EDGE('',*,*,#17367,.T.);
#24923=ORIENTED_EDGE('',*,*,#17362,.F.);
#24924=ORIENTED_EDGE('',*,*,#17368,.F.);
#24925=ORIENTED_EDGE('',*,*,#17369,.T.);
#24926=ORIENTED_EDGE('',*,*,#17370,.T.);
#24927=ORIENTED_EDGE('',*,*,#17366,.F.);
#24928=ORIENTED_EDGE('',*,*,#17371,.F.);
#24929=ORIENTED_EDGE('',*,*,#17372,.T.);
#24930=ORIENTED_EDGE('',*,*,#17373,.T.);
#24931=ORIENTED_EDGE('',*,*,#17369,.F.);
#24932=ORIENTED_EDGE('',*,*,#17374,.F.);
#24933=ORIENTED_EDGE('',*,*,#17375,.T.);
#24934=ORIENTED_EDGE('',*,*,#17376,.T.);
#24935=ORIENTED_EDGE('',*,*,#17372,.F.);
#24936=ORIENTED_EDGE('',*,*,#17377,.F.);
#24937=ORIENTED_EDGE('',*,*,#17378,.T.);
#24938=ORIENTED_EDGE('',*,*,#17379,.T.);
#24939=ORIENTED_EDGE('',*,*,#17375,.F.);
#24940=ORIENTED_EDGE('',*,*,#17380,.F.);
#24941=ORIENTED_EDGE('',*,*,#17381,.T.);
#24942=ORIENTED_EDGE('',*,*,#17382,.T.);
#24943=ORIENTED_EDGE('',*,*,#17378,.F.);
#24944=ORIENTED_EDGE('',*,*,#17383,.F.);
#24945=ORIENTED_EDGE('',*,*,#17364,.T.);
#24946=ORIENTED_EDGE('',*,*,#17384,.T.);
#24947=ORIENTED_EDGE('',*,*,#17381,.F.);
#24948=ORIENTED_EDGE('',*,*,#17385,.F.);
#24949=ORIENTED_EDGE('',*,*,#17386,.T.);
#24950=ORIENTED_EDGE('',*,*,#17387,.T.);
#24951=ORIENTED_EDGE('',*,*,#17388,.F.);
#24952=ORIENTED_EDGE('',*,*,#17389,.F.);
#24953=ORIENTED_EDGE('',*,*,#17390,.T.);
#24954=ORIENTED_EDGE('',*,*,#17391,.T.);
#24955=ORIENTED_EDGE('',*,*,#17386,.F.);
#24956=ORIENTED_EDGE('',*,*,#17392,.F.);
#24957=ORIENTED_EDGE('',*,*,#17393,.T.);
#24958=ORIENTED_EDGE('',*,*,#17394,.T.);
#24959=ORIENTED_EDGE('',*,*,#17390,.F.);
#24960=ORIENTED_EDGE('',*,*,#17395,.F.);
#24961=ORIENTED_EDGE('',*,*,#17396,.T.);
#24962=ORIENTED_EDGE('',*,*,#17397,.T.);
#24963=ORIENTED_EDGE('',*,*,#17393,.F.);
#24964=ORIENTED_EDGE('',*,*,#17398,.F.);
#24965=ORIENTED_EDGE('',*,*,#17399,.T.);
#24966=ORIENTED_EDGE('',*,*,#17400,.T.);
#24967=ORIENTED_EDGE('',*,*,#17396,.F.);
#24968=ORIENTED_EDGE('',*,*,#17401,.F.);
#24969=ORIENTED_EDGE('',*,*,#17402,.T.);
#24970=ORIENTED_EDGE('',*,*,#17403,.T.);
#24971=ORIENTED_EDGE('',*,*,#17399,.F.);
#24972=ORIENTED_EDGE('',*,*,#17404,.F.);
#24973=ORIENTED_EDGE('',*,*,#17405,.T.);
#24974=ORIENTED_EDGE('',*,*,#17406,.T.);
#24975=ORIENTED_EDGE('',*,*,#17402,.F.);
#24976=ORIENTED_EDGE('',*,*,#17407,.F.);
#24977=ORIENTED_EDGE('',*,*,#17408,.T.);
#24978=ORIENTED_EDGE('',*,*,#17409,.T.);
#24979=ORIENTED_EDGE('',*,*,#17405,.F.);
#24980=ORIENTED_EDGE('',*,*,#17410,.F.);
#24981=ORIENTED_EDGE('',*,*,#17388,.T.);
#24982=ORIENTED_EDGE('',*,*,#17411,.T.);
#24983=ORIENTED_EDGE('',*,*,#17408,.F.);
#24984=ORIENTED_EDGE('',*,*,#17412,.F.);
#24985=ORIENTED_EDGE('',*,*,#17413,.T.);
#24986=ORIENTED_EDGE('',*,*,#17414,.T.);
#24987=ORIENTED_EDGE('',*,*,#17415,.F.);
#24988=ORIENTED_EDGE('',*,*,#17416,.F.);
#24989=ORIENTED_EDGE('',*,*,#17417,.T.);
#24990=ORIENTED_EDGE('',*,*,#17418,.T.);
#24991=ORIENTED_EDGE('',*,*,#17413,.F.);
#24992=ORIENTED_EDGE('',*,*,#17419,.F.);
#24993=ORIENTED_EDGE('',*,*,#17420,.T.);
#24994=ORIENTED_EDGE('',*,*,#17421,.T.);
#24995=ORIENTED_EDGE('',*,*,#17417,.F.);
#24996=ORIENTED_EDGE('',*,*,#17422,.F.);
#24997=ORIENTED_EDGE('',*,*,#17423,.T.);
#24998=ORIENTED_EDGE('',*,*,#17424,.T.);
#24999=ORIENTED_EDGE('',*,*,#17420,.F.);
#25000=ORIENTED_EDGE('',*,*,#17425,.F.);
#25001=ORIENTED_EDGE('',*,*,#17426,.T.);
#25002=ORIENTED_EDGE('',*,*,#17427,.T.);
#25003=ORIENTED_EDGE('',*,*,#17423,.F.);
#25004=ORIENTED_EDGE('',*,*,#17428,.F.);
#25005=ORIENTED_EDGE('',*,*,#17429,.T.);
#25006=ORIENTED_EDGE('',*,*,#17430,.T.);
#25007=ORIENTED_EDGE('',*,*,#17426,.F.);
#25008=ORIENTED_EDGE('',*,*,#17431,.F.);
#25009=ORIENTED_EDGE('',*,*,#17432,.T.);
#25010=ORIENTED_EDGE('',*,*,#17433,.T.);
#25011=ORIENTED_EDGE('',*,*,#17429,.F.);
#25012=ORIENTED_EDGE('',*,*,#17434,.F.);
#25013=ORIENTED_EDGE('',*,*,#17435,.T.);
#25014=ORIENTED_EDGE('',*,*,#17436,.T.);
#25015=ORIENTED_EDGE('',*,*,#17432,.F.);
#25016=ORIENTED_EDGE('',*,*,#17437,.F.);
#25017=ORIENTED_EDGE('',*,*,#17438,.T.);
#25018=ORIENTED_EDGE('',*,*,#17439,.T.);
#25019=ORIENTED_EDGE('',*,*,#17435,.F.);
#25020=ORIENTED_EDGE('',*,*,#17440,.F.);
#25021=ORIENTED_EDGE('',*,*,#17441,.T.);
#25022=ORIENTED_EDGE('',*,*,#17442,.T.);
#25023=ORIENTED_EDGE('',*,*,#17438,.F.);
#25024=ORIENTED_EDGE('',*,*,#17443,.F.);
#25025=ORIENTED_EDGE('',*,*,#17444,.T.);
#25026=ORIENTED_EDGE('',*,*,#17445,.T.);
#25027=ORIENTED_EDGE('',*,*,#17441,.F.);
#25028=ORIENTED_EDGE('',*,*,#17446,.F.);
#25029=ORIENTED_EDGE('',*,*,#17447,.T.);
#25030=ORIENTED_EDGE('',*,*,#17448,.T.);
#25031=ORIENTED_EDGE('',*,*,#17444,.F.);
#25032=ORIENTED_EDGE('',*,*,#17449,.F.);
#25033=ORIENTED_EDGE('',*,*,#17450,.T.);
#25034=ORIENTED_EDGE('',*,*,#17451,.T.);
#25035=ORIENTED_EDGE('',*,*,#17447,.F.);
#25036=ORIENTED_EDGE('',*,*,#17452,.F.);
#25037=ORIENTED_EDGE('',*,*,#17453,.T.);
#25038=ORIENTED_EDGE('',*,*,#17454,.T.);
#25039=ORIENTED_EDGE('',*,*,#17450,.F.);
#25040=ORIENTED_EDGE('',*,*,#17455,.F.);
#25041=ORIENTED_EDGE('',*,*,#17456,.T.);
#25042=ORIENTED_EDGE('',*,*,#17457,.T.);
#25043=ORIENTED_EDGE('',*,*,#17453,.F.);
#25044=ORIENTED_EDGE('',*,*,#17458,.F.);
#25045=ORIENTED_EDGE('',*,*,#17415,.T.);
#25046=ORIENTED_EDGE('',*,*,#17459,.T.);
#25047=ORIENTED_EDGE('',*,*,#17456,.F.);
#25048=ORIENTED_EDGE('',*,*,#17459,.F.);
#25049=ORIENTED_EDGE('',*,*,#17414,.F.);
#25050=ORIENTED_EDGE('',*,*,#17418,.F.);
#25051=ORIENTED_EDGE('',*,*,#17421,.F.);
#25052=ORIENTED_EDGE('',*,*,#17424,.F.);
#25053=ORIENTED_EDGE('',*,*,#17427,.F.);
#25054=ORIENTED_EDGE('',*,*,#17430,.F.);
#25055=ORIENTED_EDGE('',*,*,#17433,.F.);
#25056=ORIENTED_EDGE('',*,*,#17436,.F.);
#25057=ORIENTED_EDGE('',*,*,#17439,.F.);
#25058=ORIENTED_EDGE('',*,*,#17442,.F.);
#25059=ORIENTED_EDGE('',*,*,#17445,.F.);
#25060=ORIENTED_EDGE('',*,*,#17448,.F.);
#25061=ORIENTED_EDGE('',*,*,#17451,.F.);
#25062=ORIENTED_EDGE('',*,*,#17454,.F.);
#25063=ORIENTED_EDGE('',*,*,#17457,.F.);
#25064=ORIENTED_EDGE('',*,*,#17411,.F.);
#25065=ORIENTED_EDGE('',*,*,#17387,.F.);
#25066=ORIENTED_EDGE('',*,*,#17391,.F.);
#25067=ORIENTED_EDGE('',*,*,#17394,.F.);
#25068=ORIENTED_EDGE('',*,*,#17397,.F.);
#25069=ORIENTED_EDGE('',*,*,#17400,.F.);
#25070=ORIENTED_EDGE('',*,*,#17403,.F.);
#25071=ORIENTED_EDGE('',*,*,#17406,.F.);
#25072=ORIENTED_EDGE('',*,*,#17409,.F.);
#25073=ORIENTED_EDGE('',*,*,#17384,.F.);
#25074=ORIENTED_EDGE('',*,*,#17363,.F.);
#25075=ORIENTED_EDGE('',*,*,#17367,.F.);
#25076=ORIENTED_EDGE('',*,*,#17370,.F.);
#25077=ORIENTED_EDGE('',*,*,#17373,.F.);
#25078=ORIENTED_EDGE('',*,*,#17376,.F.);
#25079=ORIENTED_EDGE('',*,*,#17379,.F.);
#25080=ORIENTED_EDGE('',*,*,#17382,.F.);
#25081=ORIENTED_EDGE('',*,*,#17385,.T.);
#25082=ORIENTED_EDGE('',*,*,#17410,.T.);
#25083=ORIENTED_EDGE('',*,*,#17407,.T.);
#25084=ORIENTED_EDGE('',*,*,#17404,.T.);
#25085=ORIENTED_EDGE('',*,*,#17401,.T.);
#25086=ORIENTED_EDGE('',*,*,#17398,.T.);
#25087=ORIENTED_EDGE('',*,*,#17395,.T.);
#25088=ORIENTED_EDGE('',*,*,#17392,.T.);
#25089=ORIENTED_EDGE('',*,*,#17389,.T.);
#25090=ORIENTED_EDGE('',*,*,#17361,.T.);
#25091=ORIENTED_EDGE('',*,*,#17383,.T.);
#25092=ORIENTED_EDGE('',*,*,#17380,.T.);
#25093=ORIENTED_EDGE('',*,*,#17377,.T.);
#25094=ORIENTED_EDGE('',*,*,#17374,.T.);
#25095=ORIENTED_EDGE('',*,*,#17371,.T.);
#25096=ORIENTED_EDGE('',*,*,#17368,.T.);
#25097=ORIENTED_EDGE('',*,*,#17365,.T.);
#25098=ORIENTED_EDGE('',*,*,#17274,.T.);
#25099=ORIENTED_EDGE('',*,*,#17299,.T.);
#25100=ORIENTED_EDGE('',*,*,#17296,.T.);
#25101=ORIENTED_EDGE('',*,*,#17293,.T.);
#25102=ORIENTED_EDGE('',*,*,#17290,.T.);
#25103=ORIENTED_EDGE('',*,*,#17287,.T.);
#25104=ORIENTED_EDGE('',*,*,#17284,.T.);
#25105=ORIENTED_EDGE('',*,*,#17281,.T.);
#25106=ORIENTED_EDGE('',*,*,#17278,.T.);
#25107=ORIENTED_EDGE('',*,*,#17250,.T.);
#25108=ORIENTED_EDGE('',*,*,#17272,.T.);
#25109=ORIENTED_EDGE('',*,*,#17269,.T.);
#25110=ORIENTED_EDGE('',*,*,#17266,.T.);
#25111=ORIENTED_EDGE('',*,*,#17263,.T.);
#25112=ORIENTED_EDGE('',*,*,#17260,.T.);
#25113=ORIENTED_EDGE('',*,*,#17257,.T.);
#25114=ORIENTED_EDGE('',*,*,#17254,.T.);
#25115=ORIENTED_EDGE('',*,*,#17209,.T.);
#25116=ORIENTED_EDGE('',*,*,#17460,.T.);
#25117=ORIENTED_EDGE('',*,*,#17461,.F.);
#25118=ORIENTED_EDGE('',*,*,#17462,.F.);
#25119=ORIENTED_EDGE('',*,*,#17463,.T.);
#25120=ORIENTED_EDGE('',*,*,#17463,.F.);
#25121=ORIENTED_EDGE('',*,*,#17464,.F.);
#25122=ORIENTED_EDGE('',*,*,#17206,.F.);
#25123=ORIENTED_EDGE('',*,*,#17202,.F.);
#25124=ORIENTED_EDGE('',*,*,#17199,.F.);
#25125=ORIENTED_EDGE('',*,*,#17196,.F.);
#25126=ORIENTED_EDGE('',*,*,#17193,.F.);
#25127=ORIENTED_EDGE('',*,*,#17190,.F.);
#25128=ORIENTED_EDGE('',*,*,#17187,.F.);
#25129=ORIENTED_EDGE('',*,*,#17184,.F.);
#25130=ORIENTED_EDGE('',*,*,#17181,.F.);
#25131=ORIENTED_EDGE('',*,*,#17178,.F.);
#25132=ORIENTED_EDGE('',*,*,#17175,.F.);
#25133=ORIENTED_EDGE('',*,*,#17172,.F.);
#25134=ORIENTED_EDGE('',*,*,#17169,.F.);
#25135=ORIENTED_EDGE('',*,*,#17166,.F.);
#25136=ORIENTED_EDGE('',*,*,#17163,.F.);
#25137=ORIENTED_EDGE('',*,*,#17465,.F.);
#25138=ORIENTED_EDGE('',*,*,#17466,.T.);
#25139=ORIENTED_EDGE('',*,*,#17249,.T.);
#25140=ORIENTED_EDGE('',*,*,#17246,.T.);
#25141=ORIENTED_EDGE('',*,*,#17243,.T.);
#25142=ORIENTED_EDGE('',*,*,#17240,.T.);
#25143=ORIENTED_EDGE('',*,*,#17237,.T.);
#25144=ORIENTED_EDGE('',*,*,#17234,.T.);
#25145=ORIENTED_EDGE('',*,*,#17231,.T.);
#25146=ORIENTED_EDGE('',*,*,#17228,.T.);
#25147=ORIENTED_EDGE('',*,*,#17225,.T.);
#25148=ORIENTED_EDGE('',*,*,#17222,.T.);
#25149=ORIENTED_EDGE('',*,*,#17219,.T.);
#25150=ORIENTED_EDGE('',*,*,#17216,.T.);
#25151=ORIENTED_EDGE('',*,*,#17213,.T.);
#25152=ORIENTED_EDGE('',*,*,#17210,.T.);
#25153=ORIENTED_EDGE('',*,*,#17467,.T.);
#25154=ORIENTED_EDGE('',*,*,#17468,.T.);
#25155=ORIENTED_EDGE('',*,*,#17469,.T.);
#25156=ORIENTED_EDGE('',*,*,#17470,.T.);
#25157=ORIENTED_EDGE('',*,*,#17465,.T.);
#25158=ORIENTED_EDGE('',*,*,#17247,.T.);
#25159=ORIENTED_EDGE('',*,*,#17466,.F.);
#25160=ORIENTED_EDGE('',*,*,#17470,.F.);
#25161=ORIENTED_EDGE('',*,*,#17471,.T.);
#25162=ORIENTED_EDGE('',*,*,#17460,.F.);
#25163=ORIENTED_EDGE('',*,*,#17208,.F.);
#25164=ORIENTED_EDGE('',*,*,#17212,.F.);
#25165=ORIENTED_EDGE('',*,*,#17215,.F.);
#25166=ORIENTED_EDGE('',*,*,#17218,.F.);
#25167=ORIENTED_EDGE('',*,*,#17221,.F.);
#25168=ORIENTED_EDGE('',*,*,#17224,.F.);
#25169=ORIENTED_EDGE('',*,*,#17227,.F.);
#25170=ORIENTED_EDGE('',*,*,#17230,.F.);
#25171=ORIENTED_EDGE('',*,*,#17233,.F.);
#25172=ORIENTED_EDGE('',*,*,#17236,.F.);
#25173=ORIENTED_EDGE('',*,*,#17239,.F.);
#25174=ORIENTED_EDGE('',*,*,#17242,.F.);
#25175=ORIENTED_EDGE('',*,*,#17245,.F.);
#25176=ORIENTED_EDGE('',*,*,#17248,.F.);
#25177=ORIENTED_EDGE('',*,*,#17471,.F.);
#25178=ORIENTED_EDGE('',*,*,#17469,.F.);
#25179=ORIENTED_EDGE('',*,*,#17161,.F.);
#25180=ORIENTED_EDGE('',*,*,#17165,.F.);
#25181=ORIENTED_EDGE('',*,*,#17168,.F.);
#25182=ORIENTED_EDGE('',*,*,#17171,.F.);
#25183=ORIENTED_EDGE('',*,*,#17174,.F.);
#25184=ORIENTED_EDGE('',*,*,#17177,.F.);
#25185=ORIENTED_EDGE('',*,*,#17180,.F.);
#25186=ORIENTED_EDGE('',*,*,#17183,.F.);
#25187=ORIENTED_EDGE('',*,*,#17186,.F.);
#25188=ORIENTED_EDGE('',*,*,#17189,.F.);
#25189=ORIENTED_EDGE('',*,*,#17192,.F.);
#25190=ORIENTED_EDGE('',*,*,#17195,.F.);
#25191=ORIENTED_EDGE('',*,*,#17198,.F.);
#25192=ORIENTED_EDGE('',*,*,#17201,.F.);
#25193=ORIENTED_EDGE('',*,*,#17205,.F.);
#25194=ORIENTED_EDGE('',*,*,#17472,.T.);
#25195=ORIENTED_EDGE('',*,*,#17473,.T.);
#25196=ORIENTED_EDGE('',*,*,#17461,.T.);
#25197=ORIENTED_EDGE('',*,*,#17204,.T.);
#25198=ORIENTED_EDGE('',*,*,#17474,.T.);
#25199=ORIENTED_EDGE('',*,*,#17462,.T.);
#25200=ORIENTED_EDGE('',*,*,#17473,.F.);
#25201=ORIENTED_EDGE('',*,*,#17475,.F.);
#25202=ORIENTED_EDGE('',*,*,#17476,.F.);
#25203=ORIENTED_EDGE('',*,*,#17477,.F.);
#25204=ORIENTED_EDGE('',*,*,#17478,.F.);
#25205=ORIENTED_EDGE('',*,*,#17479,.F.);
#25206=ORIENTED_EDGE('',*,*,#17480,.F.);
#25207=ORIENTED_EDGE('',*,*,#17472,.F.);
#25208=ORIENTED_EDGE('',*,*,#17203,.T.);
#25209=ORIENTED_EDGE('',*,*,#17464,.T.);
#25210=ORIENTED_EDGE('',*,*,#17474,.F.);
#25211=ORIENTED_EDGE('',*,*,#17481,.F.);
#25212=ORIENTED_EDGE('',*,*,#17482,.F.);
#25213=ORIENTED_EDGE('',*,*,#17483,.F.);
#25214=ORIENTED_EDGE('',*,*,#17484,.F.);
#25215=ORIENTED_EDGE('',*,*,#17485,.F.);
#25216=ORIENTED_EDGE('',*,*,#17486,.T.);
#25217=ORIENTED_EDGE('',*,*,#17487,.F.);
#25218=ORIENTED_EDGE('',*,*,#17486,.F.);
#25219=ORIENTED_EDGE('',*,*,#17488,.F.);
#25220=ORIENTED_EDGE('',*,*,#17489,.F.);
#25221=ORIENTED_EDGE('',*,*,#17484,.T.);
#25222=ORIENTED_EDGE('',*,*,#17490,.F.);
#25223=ORIENTED_EDGE('',*,*,#17479,.T.);
#25224=ORIENTED_EDGE('',*,*,#17491,.T.);
#25225=ORIENTED_EDGE('',*,*,#17483,.T.);
#25226=ORIENTED_EDGE('',*,*,#17492,.F.);
#25227=ORIENTED_EDGE('',*,*,#17480,.T.);
#25228=ORIENTED_EDGE('',*,*,#17490,.T.);
#25229=ORIENTED_EDGE('',*,*,#17482,.T.);
#25230=ORIENTED_EDGE('',*,*,#17493,.F.);
#25231=ORIENTED_EDGE('',*,*,#17475,.T.);
#25232=ORIENTED_EDGE('',*,*,#17492,.T.);
#25233=ORIENTED_EDGE('',*,*,#17481,.T.);
#25234=ORIENTED_EDGE('',*,*,#17494,.F.);
#25235=ORIENTED_EDGE('',*,*,#17476,.T.);
#25236=ORIENTED_EDGE('',*,*,#17493,.T.);
#25237=ORIENTED_EDGE('',*,*,#17489,.T.);
#25238=ORIENTED_EDGE('',*,*,#17495,.F.);
#25239=ORIENTED_EDGE('',*,*,#17477,.T.);
#25240=ORIENTED_EDGE('',*,*,#17494,.T.);
#25241=ORIENTED_EDGE('',*,*,#17488,.T.);
#25242=ORIENTED_EDGE('',*,*,#17485,.T.);
#25243=ORIENTED_EDGE('',*,*,#17491,.F.);
#25244=ORIENTED_EDGE('',*,*,#17478,.T.);
#25245=ORIENTED_EDGE('',*,*,#17495,.T.);
#25246=ORIENTED_EDGE('',*,*,#17487,.T.);
#25247=ORIENTED_EDGE('',*,*,#17412,.T.);
#25248=ORIENTED_EDGE('',*,*,#17458,.T.);
#25249=ORIENTED_EDGE('',*,*,#17455,.T.);
#25250=ORIENTED_EDGE('',*,*,#17452,.T.);
#25251=ORIENTED_EDGE('',*,*,#17449,.T.);
#25252=ORIENTED_EDGE('',*,*,#17446,.T.);
#25253=ORIENTED_EDGE('',*,*,#17443,.T.);
#25254=ORIENTED_EDGE('',*,*,#17440,.T.);
#25255=ORIENTED_EDGE('',*,*,#17437,.T.);
#25256=ORIENTED_EDGE('',*,*,#17434,.T.);
#25257=ORIENTED_EDGE('',*,*,#17431,.T.);
#25258=ORIENTED_EDGE('',*,*,#17428,.T.);
#25259=ORIENTED_EDGE('',*,*,#17425,.T.);
#25260=ORIENTED_EDGE('',*,*,#17422,.T.);
#25261=ORIENTED_EDGE('',*,*,#17419,.T.);
#25262=ORIENTED_EDGE('',*,*,#17416,.T.);
#25263=ORIENTED_EDGE('',*,*,#17349,.T.);
#25264=ORIENTED_EDGE('',*,*,#17359,.T.);
#25265=ORIENTED_EDGE('',*,*,#17356,.T.);
#25266=ORIENTED_EDGE('',*,*,#17353,.T.);
#25267=ORIENTED_EDGE('',*,*,#17301,.T.);
#25268=ORIENTED_EDGE('',*,*,#17347,.T.);
#25269=ORIENTED_EDGE('',*,*,#17344,.T.);
#25270=ORIENTED_EDGE('',*,*,#17341,.T.);
#25271=ORIENTED_EDGE('',*,*,#17338,.T.);
#25272=ORIENTED_EDGE('',*,*,#17335,.T.);
#25273=ORIENTED_EDGE('',*,*,#17332,.T.);
#25274=ORIENTED_EDGE('',*,*,#17329,.T.);
#25275=ORIENTED_EDGE('',*,*,#17326,.T.);
#25276=ORIENTED_EDGE('',*,*,#17323,.T.);
#25277=ORIENTED_EDGE('',*,*,#17320,.T.);
#25278=ORIENTED_EDGE('',*,*,#17317,.T.);
#25279=ORIENTED_EDGE('',*,*,#17314,.T.);
#25280=ORIENTED_EDGE('',*,*,#17311,.T.);
#25281=ORIENTED_EDGE('',*,*,#17308,.T.);
#25282=ORIENTED_EDGE('',*,*,#17305,.T.);
#25283=ORIENTED_EDGE('',*,*,#17496,.F.);
#25284=ORIENTED_EDGE('',*,*,#17467,.F.);
#25285=ORIENTED_EDGE('',*,*,#17162,.F.);
#25286=ORIENTED_EDGE('',*,*,#17468,.F.);
#25287=ORIENTED_EDGE('',*,*,#17497,.T.);
#25288=ORIENTED_EDGE('',*,*,#17496,.T.);
#25289=ORIENTED_EDGE('',*,*,#17497,.F.);
#25381=CONICAL_SURFACE('',#28950,1.28782032302755,1.0471975511966);
#25382=CONICAL_SURFACE('',#28961,0.75,0.785398163397448);
#26748=ADVANCED_FACE('',(#3935),#814,.T.);
#26749=ADVANCED_FACE('',(#3936),#815,.T.);
#26750=ADVANCED_FACE('',(#3937),#816,.T.);
#26751=ADVANCED_FACE('',(#3938),#817,.T.);
#26752=ADVANCED_FACE('',(#3939),#818,.T.);
#26753=ADVANCED_FACE('',(#3940),#819,.T.);
#26754=ADVANCED_FACE('',(#3941),#820,.T.);
#26755=ADVANCED_FACE('',(#3942),#821,.T.);
#26756=ADVANCED_FACE('',(#3943),#822,.T.);
#26757=ADVANCED_FACE('',(#3944),#823,.T.);
#26758=ADVANCED_FACE('',(#3945),#824,.T.);
#26759=ADVANCED_FACE('',(#3946),#825,.T.);
#26760=ADVANCED_FACE('',(#3947),#826,.T.);
#26761=ADVANCED_FACE('',(#3948),#827,.T.);
#26762=ADVANCED_FACE('',(#3949),#828,.T.);
#26763=ADVANCED_FACE('',(#3950),#829,.T.);
#26764=ADVANCED_FACE('',(#3951),#830,.T.);
#26765=ADVANCED_FACE('',(#3952),#831,.T.);
#26766=ADVANCED_FACE('',(#3953),#832,.T.);
#26767=ADVANCED_FACE('',(#3954),#833,.T.);
#26768=ADVANCED_FACE('',(#3955),#834,.T.);
#26769=ADVANCED_FACE('',(#3956),#835,.T.);
#26770=ADVANCED_FACE('',(#3957),#836,.T.);
#26771=ADVANCED_FACE('',(#3958),#837,.T.);
#26772=ADVANCED_FACE('',(#3959),#838,.T.);
#26773=ADVANCED_FACE('',(#3960),#839,.T.);
#26774=ADVANCED_FACE('',(#3961),#840,.T.);
#26775=ADVANCED_FACE('',(#3962),#841,.T.);
#26776=ADVANCED_FACE('',(#3963),#842,.T.);
#26777=ADVANCED_FACE('',(#3964),#309,.F.);
#26778=ADVANCED_FACE('',(#3965),#310,.F.);
#26779=ADVANCED_FACE('',(#3966),#311,.F.);
#26780=ADVANCED_FACE('',(#3967),#312,.F.);
#26781=ADVANCED_FACE('',(#3968),#313,.F.);
#26782=ADVANCED_FACE('',(#3969),#314,.F.);
#26783=ADVANCED_FACE('',(#3970),#315,.F.);
#26784=ADVANCED_FACE('',(#3971),#316,.F.);
#26785=ADVANCED_FACE('',(#3972),#317,.F.);
#26786=ADVANCED_FACE('',(#3973),#318,.F.);
#26787=ADVANCED_FACE('',(#3974),#319,.F.);
#26788=ADVANCED_FACE('',(#3975),#320,.F.);
#26789=ADVANCED_FACE('',(#3976),#321,.F.);
#26790=ADVANCED_FACE('',(#3977),#322,.F.);
#26791=ADVANCED_FACE('',(#3978),#323,.F.);
#26792=ADVANCED_FACE('',(#3979),#324,.F.);
#26793=ADVANCED_FACE('',(#3980),#325,.F.);
#26794=ADVANCED_FACE('',(#3981),#326,.F.);
#26795=ADVANCED_FACE('',(#3982),#327,.F.);
#26796=ADVANCED_FACE('',(#3983),#328,.F.);
#26797=ADVANCED_FACE('',(#3984),#329,.F.);
#26798=ADVANCED_FACE('',(#3985),#330,.F.);
#26799=ADVANCED_FACE('',(#3986),#331,.F.);
#26800=ADVANCED_FACE('',(#3987),#332,.F.);
#26801=ADVANCED_FACE('',(#3988),#333,.F.);
#26802=ADVANCED_FACE('',(#3989),#334,.F.);
#26803=ADVANCED_FACE('',(#3990),#335,.F.);
#26804=ADVANCED_FACE('',(#3991),#336,.F.);
#26805=ADVANCED_FACE('',(#3992),#337,.F.);
#26806=ADVANCED_FACE('',(#3993),#338,.F.);
#26807=ADVANCED_FACE('',(#3994),#339,.F.);
#26808=ADVANCED_FACE('',(#3995),#340,.F.);
#26809=ADVANCED_FACE('',(#3996),#341,.F.);
#26810=ADVANCED_FACE('',(#3997,#919,#920),#2548,.T.);
#26811=ADVANCED_FACE('',(#3998),#2549,.F.);
#26812=ADVANCED_FACE('',(#3999),#2550,.F.);
#26813=ADVANCED_FACE('',(#4000),#2551,.F.);
#26814=ADVANCED_FACE('',(#4001),#2552,.F.);
#26815=ADVANCED_FACE('',(#4002),#2553,.F.);
#26816=ADVANCED_FACE('',(#4003),#342,.F.);
#26817=ADVANCED_FACE('',(#4004),#343,.F.);
#26818=ADVANCED_FACE('',(#4005),#344,.F.);
#26819=ADVANCED_FACE('',(#4006),#345,.F.);
#26820=ADVANCED_FACE('',(#4007),#346,.F.);
#26821=ADVANCED_FACE('',(#4008),#347,.F.);
#26822=ADVANCED_FACE('',(#4009),#348,.F.);
#26823=ADVANCED_FACE('',(#4010),#349,.F.);
#26824=ADVANCED_FACE('',(#4011),#350,.F.);
#26825=ADVANCED_FACE('',(#4012),#351,.F.);
#26826=ADVANCED_FACE('',(#4013),#352,.F.);
#26827=ADVANCED_FACE('',(#4014),#353,.F.);
#26828=ADVANCED_FACE('',(#4015),#354,.F.);
#26829=ADVANCED_FACE('',(#4016),#355,.F.);
#26830=ADVANCED_FACE('',(#4017),#356,.F.);
#26831=ADVANCED_FACE('',(#4018),#357,.F.);
#26832=ADVANCED_FACE('',(#4019),#358,.F.);
#26833=ADVANCED_FACE('',(#4020),#359,.F.);
#26834=ADVANCED_FACE('',(#4021),#360,.F.);
#26835=ADVANCED_FACE('',(#4022),#361,.F.);
#26836=ADVANCED_FACE('',(#4023),#362,.F.);
#26837=ADVANCED_FACE('',(#4024),#363,.F.);
#26838=ADVANCED_FACE('',(#4025),#364,.F.);
#26839=ADVANCED_FACE('',(#4026),#365,.F.);
#26840=ADVANCED_FACE('',(#4027),#366,.F.);
#26841=ADVANCED_FACE('',(#4028),#367,.F.);
#26842=ADVANCED_FACE('',(#4029),#368,.F.);
#26843=ADVANCED_FACE('',(#4030),#369,.F.);
#26844=ADVANCED_FACE('',(#4031),#370,.F.);
#26845=ADVANCED_FACE('',(#4032),#371,.F.);
#26846=ADVANCED_FACE('',(#4033),#372,.F.);
#26847=ADVANCED_FACE('',(#4034),#373,.F.);
#26848=ADVANCED_FACE('',(#4035),#374,.F.);
#26849=ADVANCED_FACE('',(#4036,#921,#922),#2554,.T.);
#26850=ADVANCED_FACE('',(#4037),#2555,.T.);
#26851=ADVANCED_FACE('',(#4038),#2556,.T.);
#26852=ADVANCED_FACE('',(#4039),#2557,.T.);
#26853=ADVANCED_FACE('',(#4040),#2558,.T.);
#26854=ADVANCED_FACE('',(#4041),#2559,.F.);
#26855=ADVANCED_FACE('',(#4042),#375,.F.);
#26856=ADVANCED_FACE('',(#4043),#2560,.T.);
#26857=ADVANCED_FACE('',(#4044),#843,.T.);
#26858=ADVANCED_FACE('',(#4045),#376,.F.);
#26859=ADVANCED_FACE('',(#4046),#170,.F.);
#26860=ADVANCED_FACE('',(#4047,#923),#2561,.F.);
#26861=ADVANCED_FACE('',(#4048),#844,.T.);
#26862=ADVANCED_FACE('',(#4049),#25381,.T.);
#26863=ADVANCED_FACE('',(#4050),#2562,.T.);
#26864=ADVANCED_FACE('',(#4051),#2563,.T.);
#26865=ADVANCED_FACE('',(#4052),#2564,.T.);
#26866=ADVANCED_FACE('',(#4053),#2565,.T.);
#26867=ADVANCED_FACE('',(#4054),#2566,.T.);
#26868=ADVANCED_FACE('',(#4055),#2567,.T.);
#26869=ADVANCED_FACE('',(#4056,#924,#925,#926),#2568,.T.);
#26870=ADVANCED_FACE('',(#4057),#2569,.T.);
#26871=ADVANCED_FACE('',(#4058),#25382,.T.);
#26886=CLOSED_SHELL('',(#26748,#26749,#26750,#26751,#26752,#26753,#26754,
#26755,#26756,#26757,#26758,#26759,#26760,#26761,#26762,#26763,#26764,#26765,
#26766,#26767,#26768,#26769,#26770,#26771,#26772,#26773,#26774,#26775,#26776,
#26777,#26778,#26779,#26780,#26781,#26782,#26783,#26784,#26785,#26786,#26787,
#26788,#26789,#26790,#26791,#26792,#26793,#26794,#26795,#26796,#26797,#26798,
#26799,#26800,#26801,#26802,#26803,#26804,#26805,#26806,#26807,#26808,#26809,
#26810,#26811,#26812,#26813,#26814,#26815,#26816,#26817,#26818,#26819,#26820,
#26821,#26822,#26823,#26824,#26825,#26826,#26827,#26828,#26829,#26830,#26831,
#26832,#26833,#26834,#26835,#26836,#26837,#26838,#26839,#26840,#26841,#26842,
#26843,#26844,#26845,#26846,#26847,#26848,#26849,#26850,#26851,#26852,#26853,
#26854,#26855,#26856,#26857,#26858,#26859,#26860,#26861,#26862,#26863,#26864,
#26865,#26866,#26867,#26868,#26869,#26870,#26871));
#28892=AXIS2_PLACEMENT_3D('',#66000,#35039,#35040);
#28893=AXIS2_PLACEMENT_3D('',#66001,#35041,#35042);
#28894=AXIS2_PLACEMENT_3D('',#66023,#35044,#35045);
#28895=AXIS2_PLACEMENT_3D('',#66034,#35046,#35047);
#28896=AXIS2_PLACEMENT_3D('',#66118,#35049,#35050);
#28897=AXIS2_PLACEMENT_3D('',#66208,#35052,#35053);
#28898=AXIS2_PLACEMENT_3D('',#66298,#35055,#35056);
#28899=AXIS2_PLACEMENT_3D('',#66382,#35058,#35059);
#28900=AXIS2_PLACEMENT_3D('',#66472,#35061,#35062);
#28901=AXIS2_PLACEMENT_3D('',#66559,#35064,#35065);
#28902=AXIS2_PLACEMENT_3D('',#66646,#35067,#35068);
#28903=AXIS2_PLACEMENT_3D('',#66736,#35070,#35071);
#28904=AXIS2_PLACEMENT_3D('',#66820,#35073,#35074);
#28905=AXIS2_PLACEMENT_3D('',#66910,#35076,#35077);
#28906=AXIS2_PLACEMENT_3D('',#67000,#35079,#35080);
#28907=AXIS2_PLACEMENT_3D('',#67084,#35082,#35083);
#28908=AXIS2_PLACEMENT_3D('',#67174,#35085,#35086);
#28909=AXIS2_PLACEMENT_3D('',#67179,#35088,#35089);
#28910=AXIS2_PLACEMENT_3D('',#67257,#35090,#35091);
#28911=AXIS2_PLACEMENT_3D('',#67274,#35093,#35094);
#28912=AXIS2_PLACEMENT_3D('',#67283,#35095,#35096);
#28913=AXIS2_PLACEMENT_3D('',#67321,#35098,#35099);
#28914=AXIS2_PLACEMENT_3D('',#67358,#35101,#35102);
#28915=AXIS2_PLACEMENT_3D('',#67395,#35104,#35105);
#28916=AXIS2_PLACEMENT_3D('',#67433,#35107,#35108);
#28917=AXIS2_PLACEMENT_3D('',#67470,#35110,#35111);
#28918=AXIS2_PLACEMENT_3D('',#67507,#35113,#35114);
#28919=AXIS2_PLACEMENT_3D('',#67545,#35116,#35117);
#28920=AXIS2_PLACEMENT_3D('',#67581,#35119,#35120);
#28921=AXIS2_PLACEMENT_3D('',#67619,#35122,#35123);
#28922=AXIS2_PLACEMENT_3D('',#67656,#35125,#35126);
#28923=AXIS2_PLACEMENT_3D('',#67693,#35128,#35129);
#28924=AXIS2_PLACEMENT_3D('',#67731,#35131,#35132);
#28925=AXIS2_PLACEMENT_3D('',#68263,#35167,#35168);
#28926=AXIS2_PLACEMENT_3D('',#68264,#35169,#35170);
#28927=AXIS2_PLACEMENT_3D('',#68273,#35175,#35176);
#28928=AXIS2_PLACEMENT_3D('',#68279,#35180,#35181);
#28929=AXIS2_PLACEMENT_3D('',#68285,#35185,#35186);
#28930=AXIS2_PLACEMENT_3D('',#68288,#35189,#35190);
#28931=AXIS2_PLACEMENT_3D('',#68784,#35224,#35225);
#28932=AXIS2_PLACEMENT_3D('',#68785,#35226,#35227);
#28933=AXIS2_PLACEMENT_3D('',#68786,#35228,#35229);
#28934=AXIS2_PLACEMENT_3D('',#68787,#35230,#35231);
#28935=AXIS2_PLACEMENT_3D('',#68788,#35232,#35233);
#28936=AXIS2_PLACEMENT_3D('',#68789,#35234,#35235);
#28937=AXIS2_PLACEMENT_3D('',#68864,#35236,#35237);
#28938=AXIS2_PLACEMENT_3D('',#68866,#35238,#35239);
#28939=AXIS2_PLACEMENT_3D('',#69786,#35240,#35241);
#28940=AXIS2_PLACEMENT_3D('',#69788,#35242,#35243);
#28941=AXIS2_PLACEMENT_3D('',#69789,#35244,#35245);
#28942=AXIS2_PLACEMENT_3D('',#69870,#35246,#35247);
#28943=AXIS2_PLACEMENT_3D('',#69871,#35248,#35249);
#28944=AXIS2_PLACEMENT_3D('',#70632,#35250,#35251);
#28945=AXIS2_PLACEMENT_3D('',#70634,#35252,#35253);
#28946=AXIS2_PLACEMENT_3D('',#70635,#35254,#35255);
#28947=AXIS2_PLACEMENT_3D('',#70636,#35256,#35257);
#28948=AXIS2_PLACEMENT_3D('',#70637,#35258,#35259);
#28949=AXIS2_PLACEMENT_3D('',#70650,#35266,#35267);
#28950=AXIS2_PLACEMENT_3D('',#70651,#35268,#35269);
#28951=AXIS2_PLACEMENT_3D('',#70675,#35271,#35272);
#28952=AXIS2_PLACEMENT_3D('',#70683,#35273,#35274);
#28953=AXIS2_PLACEMENT_3D('',#70686,#35277,#35278);
#28954=AXIS2_PLACEMENT_3D('',#70688,#35280,#35281);
#28955=AXIS2_PLACEMENT_3D('',#70690,#35283,#35284);
#28956=AXIS2_PLACEMENT_3D('',#70692,#35286,#35287);
#28957=AXIS2_PLACEMENT_3D('',#70694,#35289,#35290);
#28958=AXIS2_PLACEMENT_3D('',#70695,#35291,#35292);
#28959=AXIS2_PLACEMENT_3D('',#70696,#35293,#35294);
#28960=AXIS2_PLACEMENT_3D('',#70698,#35295,#35296);
#28961=AXIS2_PLACEMENT_3D('',#70699,#35297,#35298);
#35039=DIRECTION('axis',(0.,0.,1.));
#35040=DIRECTION('refdir',(1.,0.,0.));
#35041=DIRECTION('center_axis',(0.,0.,1.));
#35042=DIRECTION('ref_axis',(1.,0.,0.));
#35043=DIRECTION('',(0.,0.,-1.));
#35044=DIRECTION('center_axis',(0.,0.,1.));
#35045=DIRECTION('ref_axis',(1.,0.,0.));
#35046=DIRECTION('center_axis',(0.,0.,1.));
#35047=DIRECTION('ref_axis',(1.,0.,0.));
#35048=DIRECTION('',(0.,0.,-1.));
#35049=DIRECTION('center_axis',(0.,0.,1.));
#35050=DIRECTION('ref_axis',(1.,0.,0.));
#35051=DIRECTION('',(0.,0.,-1.));
#35052=DIRECTION('center_axis',(0.,0.,1.));
#35053=DIRECTION('ref_axis',(1.,0.,0.));
#35054=DIRECTION('',(0.,0.,-1.));
#35055=DIRECTION('center_axis',(0.,0.,1.));
#35056=DIRECTION('ref_axis',(1.,0.,0.));
#35057=DIRECTION('',(0.,0.,-1.));
#35058=DIRECTION('center_axis',(0.,0.,1.));
#35059=DIRECTION('ref_axis',(1.,0.,0.));
#35060=DIRECTION('',(0.,0.,-1.));
#35061=DIRECTION('center_axis',(0.,0.,1.));
#35062=DIRECTION('ref_axis',(1.,0.,0.));
#35063=DIRECTION('',(0.,0.,-1.));
#35064=DIRECTION('center_axis',(0.,0.,1.));
#35065=DIRECTION('ref_axis',(1.,0.,0.));
#35066=DIRECTION('',(0.,0.,-1.));
#35067=DIRECTION('center_axis',(0.,0.,1.));
#35068=DIRECTION('ref_axis',(1.,0.,0.));
#35069=DIRECTION('',(0.,0.,-1.));
#35070=DIRECTION('center_axis',(0.,0.,1.));
#35071=DIRECTION('ref_axis',(1.,0.,0.));
#35072=DIRECTION('',(0.,0.,-1.));
#35073=DIRECTION('center_axis',(0.,0.,1.));
#35074=DIRECTION('ref_axis',(1.,0.,0.));
#35075=DIRECTION('',(0.,0.,-1.));
#35076=DIRECTION('center_axis',(0.,0.,1.));
#35077=DIRECTION('ref_axis',(1.,0.,0.));
#35078=DIRECTION('',(0.,0.,-1.));
#35079=DIRECTION('center_axis',(0.,0.,1.));
#35080=DIRECTION('ref_axis',(1.,0.,0.));
#35081=DIRECTION('',(0.,0.,-1.));
#35082=DIRECTION('center_axis',(0.,0.,1.));
#35083=DIRECTION('ref_axis',(1.,0.,0.));
#35084=DIRECTION('',(0.,0.,-1.));
#35085=DIRECTION('center_axis',(0.,0.,1.));
#35086=DIRECTION('ref_axis',(1.,0.,0.));
#35087=DIRECTION('',(0.,0.,-1.));
#35088=DIRECTION('center_axis',(0.,0.,1.));
#35089=DIRECTION('ref_axis',(1.,0.,0.));
#35090=DIRECTION('center_axis',(0.,0.,1.));
#35091=DIRECTION('ref_axis',(0.288300159963205,-0.957540086766706,0.));
#35092=DIRECTION('',(0.,0.,1.));
#35093=DIRECTION('center_axis',(0.,0.,1.));
#35094=DIRECTION('ref_axis',(1.,9.16593808558309E-14,0.));
#35095=DIRECTION('center_axis',(0.,0.,1.));
#35096=DIRECTION('ref_axis',(1.,9.16593808558309E-14,0.));
#35097=DIRECTION('',(0.,0.,1.));
#35098=DIRECTION('center_axis',(0.,0.,1.));
#35099=DIRECTION('ref_axis',(1.,9.16593808558309E-14,0.));
#35100=DIRECTION('',(0.,0.,1.));
#35101=DIRECTION('center_axis',(0.,0.,1.));
#35102=DIRECTION('ref_axis',(1.,9.16593808558309E-14,0.));
#35103=DIRECTION('',(0.,0.,1.));
#35104=DIRECTION('center_axis',(0.,0.,1.));
#35105=DIRECTION('ref_axis',(1.,9.16593808558309E-14,0.));
#35106=DIRECTION('',(0.,0.,1.));
#35107=DIRECTION('center_axis',(0.,0.,1.));
#35108=DIRECTION('ref_axis',(1.,9.16593808558309E-14,0.));
#35109=DIRECTION('',(0.,0.,1.));
#35110=DIRECTION('center_axis',(0.,0.,1.));
#35111=DIRECTION('ref_axis',(1.,9.16593808558309E-14,0.));
#35112=DIRECTION('',(0.,0.,1.));
#35113=DIRECTION('center_axis',(0.,0.,1.));
#35114=DIRECTION('ref_axis',(1.,9.16593808558309E-14,0.));
#35115=DIRECTION('',(0.,0.,1.));
#35116=DIRECTION('center_axis',(0.,0.,1.));
#35117=DIRECTION('ref_axis',(1.,9.16593808558309E-14,0.));
#35118=DIRECTION('',(0.,0.,1.));
#35119=DIRECTION('center_axis',(0.,0.,1.));
#35120=DIRECTION('ref_axis',(1.,9.16593808558309E-14,0.));
#35121=DIRECTION('',(0.,0.,1.));
#35122=DIRECTION('center_axis',(0.,0.,1.));
#35123=DIRECTION('ref_axis',(1.,9.16593808558309E-14,0.));
#35124=DIRECTION('',(0.,0.,1.));
#35125=DIRECTION('center_axis',(0.,0.,1.));
#35126=DIRECTION('ref_axis',(1.,9.16593808558309E-14,0.));
#35127=DIRECTION('',(0.,0.,1.));
#35128=DIRECTION('center_axis',(0.,0.,1.));
#35129=DIRECTION('ref_axis',(1.,9.16593808558309E-14,0.));
#35130=DIRECTION('',(0.,0.,1.));
#35131=DIRECTION('center_axis',(0.,0.,1.));
#35132=DIRECTION('ref_axis',(1.,9.16593808558309E-14,0.));
#35133=DIRECTION('',(0.,0.,1.));
#35134=DIRECTION('',(0.,0.,-1.));
#35135=DIRECTION('',(0.,0.,-1.));
#35136=DIRECTION('',(0.,0.,-1.));
#35137=DIRECTION('',(0.,0.,-1.));
#35138=DIRECTION('',(0.,0.,-1.));
#35139=DIRECTION('',(0.,0.,-1.));
#35140=DIRECTION('',(0.,0.,-1.));
#35141=DIRECTION('',(0.,0.,-1.));
#35142=DIRECTION('',(0.,0.,-1.));
#35143=DIRECTION('',(0.,0.,-1.));
#35144=DIRECTION('',(0.,0.,-1.));
#35145=DIRECTION('',(0.,0.,-1.));
#35146=DIRECTION('',(0.,0.,-1.));
#35147=DIRECTION('',(0.,0.,-1.));
#35148=DIRECTION('',(0.,0.,-1.));
#35149=DIRECTION('',(0.,0.,-1.));
#35150=DIRECTION('',(0.,0.,-1.));
#35151=DIRECTION('',(0.,0.,-1.));
#35152=DIRECTION('',(0.,0.,-1.));
#35153=DIRECTION('',(0.,0.,-1.));
#35154=DIRECTION('',(0.,0.,-1.));
#35155=DIRECTION('',(0.,0.,-1.));
#35156=DIRECTION('',(0.,0.,-1.));
#35157=DIRECTION('',(0.,0.,-1.));
#35158=DIRECTION('',(0.,0.,-1.));
#35159=DIRECTION('',(0.,0.,-1.));
#35160=DIRECTION('',(0.,0.,-1.));
#35161=DIRECTION('',(0.,0.,-1.));
#35162=DIRECTION('',(0.,0.,-1.));
#35163=DIRECTION('',(0.,0.,-1.));
#35164=DIRECTION('',(0.,0.,-1.));
#35165=DIRECTION('',(0.,0.,-1.));
#35166=DIRECTION('',(0.,0.,-1.));
#35167=DIRECTION('center_axis',(0.,0.,1.));
#35168=DIRECTION('ref_axis',(1.,0.,0.));
#35169=DIRECTION('center_axis',(0.,1.,0.));
#35170=DIRECTION('ref_axis',(1.,0.,0.));
#35171=DIRECTION('',(1.,0.,0.));
#35172=DIRECTION('',(0.,0.,-1.));
#35173=DIRECTION('',(1.,0.,0.));
#35174=DIRECTION('',(0.,0.,-1.));
#35175=DIRECTION('center_axis',(-1.,0.,0.));
#35176=DIRECTION('ref_axis',(0.,1.,0.));
#35177=DIRECTION('',(0.,1.,0.));
#35178=DIRECTION('',(0.,0.,-1.));
#35179=DIRECTION('',(0.,1.,0.));
#35180=DIRECTION('center_axis',(0.,-1.,0.));
#35181=DIRECTION('ref_axis',(-1.,0.,0.));
#35182=DIRECTION('',(-1.,0.,0.));
#35183=DIRECTION('',(0.,0.,-1.));
#35184=DIRECTION('',(-1.,0.,0.));
#35185=DIRECTION('center_axis',(1.,0.,0.));
#35186=DIRECTION('ref_axis',(0.,-1.,0.));
#35187=DIRECTION('',(0.,-1.,0.));
#35188=DIRECTION('',(0.,-1.,0.));
#35189=DIRECTION('center_axis',(0.,0.,-1.));
#35190=DIRECTION('ref_axis',(-1.,0.,0.));
#35191=DIRECTION('',(0.,0.,-1.));
#35192=DIRECTION('',(0.,0.,-1.));
#35193=DIRECTION('',(0.,0.,-1.));
#35194=DIRECTION('',(0.,0.,-1.));
#35195=DIRECTION('',(0.,0.,-1.));
#35196=DIRECTION('',(0.,0.,-1.));
#35197=DIRECTION('',(0.,0.,-1.));
#35198=DIRECTION('',(0.,0.,-1.));
#35199=DIRECTION('',(0.,0.,-1.));
#35200=DIRECTION('',(0.,0.,-1.));
#35201=DIRECTION('',(0.,0.,-1.));
#35202=DIRECTION('',(0.,0.,-1.));
#35203=DIRECTION('',(0.,0.,-1.));
#35204=DIRECTION('',(0.,0.,-1.));
#35205=DIRECTION('',(0.,0.,-1.));
#35206=DIRECTION('',(0.,0.,-1.));
#35207=DIRECTION('',(0.,0.,-1.));
#35208=DIRECTION('',(0.,0.,-1.));
#35209=DIRECTION('',(0.,0.,-1.));
#35210=DIRECTION('',(0.,0.,-1.));
#35211=DIRECTION('',(0.,0.,-1.));
#35212=DIRECTION('',(0.,0.,-1.));
#35213=DIRECTION('',(0.,0.,-1.));
#35214=DIRECTION('',(0.,0.,-1.));
#35215=DIRECTION('',(0.,0.,-1.));
#35216=DIRECTION('',(0.,0.,-1.));
#35217=DIRECTION('',(0.,0.,-1.));
#35218=DIRECTION('',(0.,0.,-1.));
#35219=DIRECTION('',(0.,0.,-1.));
#35220=DIRECTION('',(0.,0.,-1.));
#35221=DIRECTION('',(0.,0.,-1.));
#35222=DIRECTION('',(0.,0.,-1.));
#35223=DIRECTION('',(0.,0.,-1.));
#35224=DIRECTION('center_axis',(0.,0.,1.));
#35225=DIRECTION('ref_axis',(1.,0.,0.));
#35226=DIRECTION('center_axis',(0.,0.,1.));
#35227=DIRECTION('ref_axis',(1.,0.,0.));
#35228=DIRECTION('center_axis',(0.,0.,1.));
#35229=DIRECTION('ref_axis',(1.,0.,0.));
#35230=DIRECTION('center_axis',(0.,0.,1.));
#35231=DIRECTION('ref_axis',(1.,0.,0.));
#35232=DIRECTION('center_axis',(0.,0.,1.));
#35233=DIRECTION('ref_axis',(1.,0.,0.));
#35234=DIRECTION('center_axis',(0.,0.,1.));
#35235=DIRECTION('ref_axis',(1.,0.,0.));
#35236=DIRECTION('center_axis',(0.,0.,1.));
#35237=DIRECTION('ref_axis',(1.,0.,0.));
#35238=DIRECTION('center_axis',(0.,0.,1.));
#35239=DIRECTION('ref_axis',(1.,0.,0.));
#35240=DIRECTION('center_axis',(0.,0.,1.));
#35241=DIRECTION('ref_axis',(1.,0.,0.));
#35242=DIRECTION('center_axis',(0.,0.,1.));
#35243=DIRECTION('ref_axis',(1.,0.,0.));
#35244=DIRECTION('center_axis',(0.,0.,1.));
#35245=DIRECTION('ref_axis',(1.,0.,0.));
#35246=DIRECTION('center_axis',(0.,0.,-1.));
#35247=DIRECTION('ref_axis',(1.,9.16593808558309E-14,0.));
#35248=DIRECTION('center_axis',(0.,0.,1.));
#35249=DIRECTION('ref_axis',(0.888987483758174,0.457931494572398,0.));
#35250=DIRECTION('center_axis',(0.,0.,-1.));
#35251=DIRECTION('ref_axis',(-1.,0.,0.));
#35252=DIRECTION('center_axis',(0.,0.,-1.));
#35253=DIRECTION('ref_axis',(1.,0.,0.));
#35254=DIRECTION('center_axis',(-1.22464679914735E-16,-1.,0.));
#35255=DIRECTION('ref_axis',(1.,-1.22464679914735E-16,0.));
#35256=DIRECTION('center_axis',(0.,0.,1.));
#35257=DIRECTION('ref_axis',(1.,0.,0.));
#35258=DIRECTION('center_axis',(0.,0.,1.));
#35259=DIRECTION('ref_axis',(1.,0.,0.));
#35260=DIRECTION('',(3.20493781063927E-16,1.,0.));
#35261=DIRECTION('',(0.866025403784439,0.5,0.));
#35262=DIRECTION('',(0.866025403784439,-0.5,0.));
#35263=DIRECTION('',(1.60246890531964E-16,-1.,0.));
#35264=DIRECTION('',(-0.866025403784439,-0.5,0.));
#35265=DIRECTION('',(-0.866025403784439,0.5,0.));
#35266=DIRECTION('center_axis',(0.,0.,1.));
#35267=DIRECTION('ref_axis',(-0.978794305969862,-0.204845567686921,0.));
#35268=DIRECTION('center_axis',(0.,0.,-1.));
#35269=DIRECTION('ref_axis',(1.,0.,0.));
#35270=DIRECTION('',(0.866025403784438,1.06057523872491E-16,0.5));
#35271=DIRECTION('center_axis',(0.,0.,1.));
#35272=DIRECTION('ref_axis',(1.,0.,0.));
#35273=DIRECTION('center_axis',(-0.5,0.866025403784439,0.));
#35274=DIRECTION('ref_axis',(-0.866025403784439,-0.5,0.));
#35275=DIRECTION('',(0.,0.,1.));
#35276=DIRECTION('',(0.,0.,1.));
#35277=DIRECTION('center_axis',(0.5,0.866025403784439,0.));
#35278=DIRECTION('ref_axis',(-0.866025403784439,0.5,0.));
#35279=DIRECTION('',(0.,0.,1.));
#35280=DIRECTION('center_axis',(1.,-3.20493781063927E-16,0.));
#35281=DIRECTION('ref_axis',(3.20493781063927E-16,1.,0.));
#35282=DIRECTION('',(0.,0.,1.));
#35283=DIRECTION('center_axis',(0.5,-0.866025403784439,0.));
#35284=DIRECTION('ref_axis',(0.866025403784439,0.5,0.));
#35285=DIRECTION('',(0.,0.,1.));
#35286=DIRECTION('center_axis',(-0.5,-0.866025403784439,0.));
#35287=DIRECTION('ref_axis',(0.866025403784439,-0.5,0.));
#35288=DIRECTION('',(0.,0.,1.));
#35289=DIRECTION('center_axis',(-1.,-1.60246890531964E-16,0.));
#35290=DIRECTION('ref_axis',(1.60246890531964E-16,-1.,0.));
#35291=DIRECTION('center_axis',(0.,0.,1.));
#35292=DIRECTION('ref_axis',(1.,0.,0.));
#35293=DIRECTION('center_axis',(0.,0.,-1.));
#35294=DIRECTION('ref_axis',(-1.,0.,0.));
#35295=DIRECTION('center_axis',(0.,0.,1.));
#35296=DIRECTION('ref_axis',(1.,0.,0.));
#35297=DIRECTION('center_axis',(0.,0.,1.));
#35298=DIRECTION('ref_axis',(1.,0.,0.));
#35299=DIRECTION('',(0.707106781186548,8.65956056235493E-17,-0.707106781186547));
#66000=CARTESIAN_POINT('',(0.,0.,0.));
#66001=CARTESIAN_POINT('Origin',(0.,0.,-1.425));
#66002=CARTESIAN_POINT('',(-0.791102872936695,2.03416717624305E-5,-2.8446668491763));
#66003=CARTESIAN_POINT('',(-0.791090026729892,1.30542722735929E-5,-2.87313315082371));
#66004=CARTESIAN_POINT('',(-0.7911,-9.68818082805471E-17,-1.425));
#66005=CARTESIAN_POINT('',(0.342081635505615,0.713330693753523,-2.9089));
#66006=CARTESIAN_POINT('Ctrl Pts',(-0.791102872936695,2.03416717624305E-5,
-2.8446668491763));
#66007=CARTESIAN_POINT('Ctrl Pts',(-0.791132933740977,0.0293885304818959,
-2.84584855390734));
#66008=CARTESIAN_POINT('Ctrl Pts',(-0.789528925786739,0.0587534438189118,
-2.84703025863837));
#66009=CARTESIAN_POINT('Ctrl Pts',(-0.786265627890728,0.0879327739588084,
-2.84821196336941));
#66010=CARTESIAN_POINT('Ctrl Pts',(-0.771682871848867,0.218326953851245,
-2.85349266784549));
#66011=CARTESIAN_POINT('Ctrl Pts',(-0.723965033050537,0.345015142138505,
-2.85877337232157));
#66012=CARTESIAN_POINT('Ctrl Pts',(-0.64890100849163,0.452629069386829,
-2.86405407679765));
#66013=CARTESIAN_POINT('Ctrl Pts',(-0.573836983932724,0.560242996635152,
-2.86933478127373));
#66014=CARTESIAN_POINT('Ctrl Pts',(-0.47142677361324,0.648782662844538,
-2.8746154857498));
#66015=CARTESIAN_POINT('Ctrl Pts',(-0.354094167074879,0.707505252038821,
-2.87989619022588));
#66016=CARTESIAN_POINT('Ctrl Pts',(-0.236761560536518,0.766227841233104,
-2.88517689470196));
#66017=CARTESIAN_POINT('Ctrl Pts',(-0.10450655777928,0.795133353412285,
-2.89045759917804));
#66018=CARTESIAN_POINT('Ctrl Pts',(0.0266262731194924,0.790718402262909,
-2.89573830365412));
#66019=CARTESIAN_POINT('Ctrl Pts',(0.135571996118135,0.787050441755417,
-2.90012553576941));
#66020=CARTESIAN_POINT('Ctrl Pts',(0.243743155897518,0.760383503731005,
-2.9045127678847));
#66021=CARTESIAN_POINT('Ctrl Pts',(0.342095308501471,0.713339076749545,
-2.9089));
#66022=CARTESIAN_POINT('',(-0.342067962509755,0.713322310757504,-2.9089));
#66023=CARTESIAN_POINT('Origin',(0.,0.,-2.9089));
#66024=CARTESIAN_POINT('Ctrl Pts',(-0.342067962509754,0.713322310757504,
-2.9089));
#66025=CARTESIAN_POINT('Ctrl Pts',(-0.460406866917162,0.65657384333148,
-2.90361929552392));
#66026=CARTESIAN_POINT('Ctrl Pts',(-0.564293460884465,0.569839529886298,
-2.89833859104784));
#66027=CARTESIAN_POINT('Ctrl Pts',(-0.641163354894195,0.463527805702664,
-2.89305788657176));
#66028=CARTESIAN_POINT('Ctrl Pts',(-0.718033248903927,0.357216081519026,
-2.88777718209569));
#66029=CARTESIAN_POINT('Ctrl Pts',(-0.767886442956084,0.231326946596934,
-2.88249647761961));
#66030=CARTESIAN_POINT('Ctrl Pts',(-0.784669586715434,0.101191204740451,
-2.87721577314353));
#66031=CARTESIAN_POINT('Ctrl Pts',(-0.788994719067196,0.0676543230158658,
-2.87585489903692));
#66032=CARTESIAN_POINT('Ctrl Pts',(-0.791123574843936,0.0338354119852844,
-2.87449402493032));
#66033=CARTESIAN_POINT('Ctrl Pts',(-0.791090026729892,1.30542722735929E-5,
-2.87313315082371));
#66034=CARTESIAN_POINT('Origin',(0.,0.,-1.425));
#66035=CARTESIAN_POINT('',(-0.791132110743512,-1.71897034488278E-5,-2.6446668491763));
#66036=CARTESIAN_POINT('',(-0.791144428618858,-1.44065313715571E-5,-2.6731331508237));
#66037=CARTESIAN_POINT('',(-0.7911,-9.68818082805471E-17,-1.425));
#66038=CARTESIAN_POINT('Ctrl Pts',(-0.791132110743512,-1.71897034488278E-5,
-2.6446668491763));
#66039=CARTESIAN_POINT('Ctrl Pts',(-0.791026015708889,0.111307599100088,
-2.64914676686106));
#66040=CARTESIAN_POINT('Ctrl Pts',(-0.767301189153144,0.222676174543509,
-2.65362668454582));
#66041=CARTESIAN_POINT('Ctrl Pts',(-0.721687452926102,0.324211361281666,
-2.65810660223059));
#66042=CARTESIAN_POINT('Ctrl Pts',(-0.667920246023168,0.443895996763073,
-2.66338730670667));
#66043=CARTESIAN_POINT('Ctrl Pts',(-0.583739442038409,0.549917607154516,
-2.66866801118275));
#66044=CARTESIAN_POINT('Ctrl Pts',(-0.479357396305173,0.629414230058327,
-2.67394871565882));
#66045=CARTESIAN_POINT('Ctrl Pts',(-0.374975350571937,0.708910852962139,
-2.6792294201349));
#66046=CARTESIAN_POINT('Ctrl Pts',(-0.250392063090227,0.761882488378319,
-2.68451012461098));
#66047=CARTESIAN_POINT('Ctrl Pts',(-0.120721297776761,0.781902906330603,
-2.68979082908706));
#66048=CARTESIAN_POINT('Ctrl Pts',(0.00894946753670305,0.801923324282887,
-2.69507153356314));
#66049=CARTESIAN_POINT('Ctrl Pts',(0.143707710681922,0.788992524771275,
-2.70035223803922));
#66050=CARTESIAN_POINT('Ctrl Pts',(0.267205297646592,0.744679202764205,
-2.70563294251529));
#66051=CARTESIAN_POINT('Ctrl Pts',(0.390702884611263,0.700365880757135,
-2.71091364699137));
#66052=CARTESIAN_POINT('Ctrl Pts',(0.502939815395386,0.624670036254607,
-2.71619435146745));
#66053=CARTESIAN_POINT('Ctrl Pts',(0.590300118688603,0.526774673675583,
-2.72147505594353));
#66054=CARTESIAN_POINT('Ctrl Pts',(0.677660421981819,0.428879311096558,
-2.72675576041961));
#66055=CARTESIAN_POINT('Ctrl Pts',(0.740144097784128,0.308784430441036,
-2.73203646489569));
#66056=CARTESIAN_POINT('Ctrl Pts',(0.770170967713734,0.181059290505753,
-2.73731716937176));
#66057=CARTESIAN_POINT('Ctrl Pts',(0.800197837643339,0.0533341505704711,
-2.74259787384784));
#66058=CARTESIAN_POINT('Ctrl Pts',(0.797767901700242,-0.0820212486445725,
-2.74787857832392));
#66059=CARTESIAN_POINT('Ctrl Pts',(0.763175946702779,-0.20858633702776,
-2.7531592828));
#66060=CARTESIAN_POINT('Ctrl Pts',(0.728583991705317,-0.335151425410948,
-2.75843998727608));
#66061=CARTESIAN_POINT('Ctrl Pts',(0.661830017653489,-0.452926202962279,
-2.76372069175216));
#66062=CARTESIAN_POINT('Ctrl Pts',(0.57101225153822,-0.547622862109841,
-2.76900139622824));
#66063=CARTESIAN_POINT('Ctrl Pts',(0.480194485422949,-0.642319521257404,
-2.77428210070431));
#66064=CARTESIAN_POINT('Ctrl Pts',(0.365312927244237,-0.713938062001196,
-2.77956280518039));
#66065=CARTESIAN_POINT('Ctrl Pts',(0.240304381141893,-0.753790143362176,
-2.78484350965647));
#66066=CARTESIAN_POINT('Ctrl Pts',(0.11529583503955,-0.793642224723155,
-2.79012421413255));
#66067=CARTESIAN_POINT('Ctrl Pts',(-0.0198396989864242,-0.801727846701323,
-2.79540491860863));
#66068=CARTESIAN_POINT('Ctrl Pts',(-0.148708318074358,-0.777066048525618,
-2.80068562308471));
#66069=CARTESIAN_POINT('Ctrl Pts',(-0.277576937162291,-0.752404250349915,
-2.80596632756078));
#66070=CARTESIAN_POINT('Ctrl Pts',(-0.400178641312184,-0.69499503202034,
-2.81124703203686));
#66071=CARTESIAN_POINT('Ctrl Pts',(-0.50164005756068,-0.611803078728568,
-2.81652773651294));
#66072=CARTESIAN_POINT('Ctrl Pts',(-0.603101473809176,-0.528611125436796,
-2.82180844098902));
#66073=CARTESIAN_POINT('Ctrl Pts',(-0.683422602156275,-0.419636437182826,
-2.8270891454651));
#66074=CARTESIAN_POINT('Ctrl Pts',(-0.732859329687128,-0.298099007307034,
-2.83236984994118));
#66075=CARTESIAN_POINT('Ctrl Pts',(-0.771233212274681,-0.203758963032545,
-2.83646884968622));
#66076=CARTESIAN_POINT('Ctrl Pts',(-0.790998600502259,-0.101849605433625,
-2.84056784943126));
#66077=CARTESIAN_POINT('Ctrl Pts',(-0.791102872936695,2.03416717624305E-5,
-2.8446668491763));
#66078=CARTESIAN_POINT('Ctrl Pts',(-0.791090026729892,1.30542722735929E-5,
-2.87313315082371));
#66079=CARTESIAN_POINT('Ctrl Pts',(-0.790993395516444,-0.0974080843082692,
-2.86921332045424));
#66080=CARTESIAN_POINT('Ctrl Pts',(-0.772956226440993,-0.194857818535022,
-2.86529349008476));
#66081=CARTESIAN_POINT('Ctrl Pts',(-0.737787983582658,-0.285678789184145,
-2.86137365971529));
#66082=CARTESIAN_POINT('Ctrl Pts',(-0.690410143223988,-0.408030692461386,
-2.85609295523921));
#66083=CARTESIAN_POINT('Ctrl Pts',(-0.611941369040105,-0.518352150224994,
-2.85081225076314));
#66084=CARTESIAN_POINT('Ctrl Pts',(-0.511899355351125,-0.60324695438924,
-2.84553154628706));
#66085=CARTESIAN_POINT('Ctrl Pts',(-0.411857341662145,-0.688141758553486,
-2.84025084181098));
#66086=CARTESIAN_POINT('Ctrl Pts',(-0.290242088468068,-0.74760990911837,
-2.8349701373349));
#66087=CARTESIAN_POINT('Ctrl Pts',(-0.161808168596516,-0.774443449936211,
-2.82968943285882));
#66088=CARTESIAN_POINT('Ctrl Pts',(-0.0333742487249623,-0.801276990754052,
-2.82440872838274));
#66089=CARTESIAN_POINT('Ctrl Pts',(0.101878337824068,-0.795475921824851,
-2.81912802390667));
#66090=CARTESIAN_POINT('Ctrl Pts',(0.227541932230471,-0.757740739969511,
-2.81384731943059));
#66091=CARTESIAN_POINT('Ctrl Pts',(0.353205526636875,-0.720005558114172,
-2.80856661495451));
#66092=CARTESIAN_POINT('Ctrl Pts',(0.469280128900652,-0.650336263332695,
-2.80328591047843));
#66093=CARTESIAN_POINT('Ctrl Pts',(0.561683974793613,-0.557186414195635,
-2.79800520600235));
#66094=CARTESIAN_POINT('Ctrl Pts',(0.654087820686573,-0.464036565058575,
-2.79272450152627));
#66095=CARTESIAN_POINT('Ctrl Pts',(0.722820910208717,-0.347406161565934,
-2.7874437970502));
#66096=CARTESIAN_POINT('Ctrl Pts',(0.759545036365206,-0.221443320796046,
-2.78216309257412));
#66097=CARTESIAN_POINT('Ctrl Pts',(0.796269162521695,-0.0954804800261573,
-2.77688238809804));
#66098=CARTESIAN_POINT('Ctrl Pts',(0.800984325312529,0.0398147980209764,
-2.77160168362196));
#66099=CARTESIAN_POINT('Ctrl Pts',(0.773118447809453,0.168028797714986,
-2.76632097914588));
#66100=CARTESIAN_POINT('Ctrl Pts',(0.745252570306378,0.296242797408994,
-2.7610402746698));
#66101=CARTESIAN_POINT('Ctrl Pts',(0.684805652509392,0.417375518749878,
-2.75575957019373));
#66102=CARTESIAN_POINT('Ctrl Pts',(0.599110814457919,0.516732021631281,
-2.75047886571765));
#66103=CARTESIAN_POINT('Ctrl Pts',(0.513415976406445,0.616088524512684,
-2.74519816124157));
#66104=CARTESIAN_POINT('Ctrl Pts',(0.402473218100484,0.693668808934607,
-2.73991745676549));
#66105=CARTESIAN_POINT('Ctrl Pts',(0.27974149361296,0.740061146397167,-2.73463675228941));
#66106=CARTESIAN_POINT('Ctrl Pts',(0.157009769125436,0.786453483859727,
-2.72935604781333));
#66107=CARTESIAN_POINT('Ctrl Pts',(0.0224890784563497,0.801657874362924,
-2.72407534333726));
#66108=CARTESIAN_POINT('Ctrl Pts',(-0.107501255149887,0.783829861479462,
-2.71879463886118));
#66109=CARTESIAN_POINT('Ctrl Pts',(-0.237491588756123,0.766001848595999,
-2.7135139343851));
#66110=CARTESIAN_POINT('Ctrl Pts',(-0.36295156529951,0.715141432325876,
-2.70823322990902));
#66111=CARTESIAN_POINT('Ctrl Pts',(-0.468661069712101,0.637418691408968,
-2.70295252543294));
#66112=CARTESIAN_POINT('Ctrl Pts',(-0.574370574124692,0.559695950492061,
-2.69767182095686));
#66113=CARTESIAN_POINT('Ctrl Pts',(-0.660329606406489,0.455110884928367,
-2.69239111648079));
#66114=CARTESIAN_POINT('Ctrl Pts',(-0.716110084252664,0.336351198465617,
-2.68711041200471));
#66115=CARTESIAN_POINT('Ctrl Pts',(-0.765324370666461,0.231571292490118,
-2.68245132494437));
#66116=CARTESIAN_POINT('Ctrl Pts',(-0.791046853705215,0.115757478055327,
-2.67779223788404));
#66117=CARTESIAN_POINT('Ctrl Pts',(-0.791144428618858,-1.44065313715571E-5,
-2.6731331508237));
#66118=CARTESIAN_POINT('Origin',(0.,0.,-1.425));
#66119=CARTESIAN_POINT('',(-0.79103374865932,3.27018256038314E-6,-2.4446668491763));
#66120=CARTESIAN_POINT('',(-0.791033002877254,-8.32524903205056E-7,-2.47313315082371));
#66121=CARTESIAN_POINT('',(-0.7911,-9.68818082805471E-17,-1.425));
#66122=CARTESIAN_POINT('Ctrl Pts',(-0.79103374865932,3.27018256038314E-6,
-2.4446668491763));
#66123=CARTESIAN_POINT('Ctrl Pts',(-0.791042731182178,0.0620858397671934,
-2.44716427533871));
#66124=CARTESIAN_POINT('Ctrl Pts',(-0.783823321886597,0.124166354682933,
-2.44966170150112));
#66125=CARTESIAN_POINT('Ctrl Pts',(-0.769352119996688,0.184507728644354,
-2.45215912766353));
#66126=CARTESIAN_POINT('Ctrl Pts',(-0.738753361264814,0.31209707177161,
-2.45743983213961));
#66127=CARTESIAN_POINT('Ctrl Pts',(-0.675732304910451,0.431910827705095,
-2.46272053661569));
#66128=CARTESIAN_POINT('Ctrl Pts',(-0.587934321254863,0.529413846025484,
-2.46800124109177));
#66129=CARTESIAN_POINT('Ctrl Pts',(-0.500136337599273,0.626916864345873,
-2.47328194556784));
#66130=CARTESIAN_POINT('Ctrl Pts',(-0.387561426642458,0.702109145053164,
-2.47856265004392));
#66131=CARTESIAN_POINT('Ctrl Pts',(-0.263866561671389,0.74586877136973,
-2.48384335452));
#66132=CARTESIAN_POINT('Ctrl Pts',(-0.140171696700323,0.789628397686295,
-2.48912405899608));
#66133=CARTESIAN_POINT('Ctrl Pts',(-0.00535687771500397,0.801955369612136,
-2.49440476347216));
#66134=CARTESIAN_POINT('Ctrl Pts',(0.124222897835128,0.781354246245838,
-2.49968546794824));
#66135=CARTESIAN_POINT('Ctrl Pts',(0.253802673385261,0.760753122879539,
-2.50496617242431));
#66136=CARTESIAN_POINT('Ctrl Pts',(0.378147405500207,0.707223904221101,
-2.51024687690039));
#66137=CARTESIAN_POINT('Ctrl Pts',(0.482172270479579,0.627260462689446,
-2.51552758137647));
#66138=CARTESIAN_POINT('Ctrl Pts',(0.586197135458951,0.547297021157791,
-2.52080828585255));
#66139=CARTESIAN_POINT('Ctrl Pts',(0.669902133302747,0.440899356752921,
-2.52608899032863));
#66140=CARTESIAN_POINT('Ctrl Pts',(0.72313263088872,0.320975052951074,-2.53136969480471));
#66141=CARTESIAN_POINT('Ctrl Pts',(0.776363128474693,0.201050749149226,
-2.53665039928079));
#66142=CARTESIAN_POINT('Ctrl Pts',(0.799119125802842,0.0675998059503994,
-2.54193110375686));
#66143=CARTESIAN_POINT('Ctrl Pts',(0.788639989575818,-0.0631882371553828,
-2.54721180823294));
#66144=CARTESIAN_POINT('Ctrl Pts',(0.778160853348794,-0.193976280261165,
-2.55249251270902));
#66145=CARTESIAN_POINT('Ctrl Pts',(0.734446583566596,-0.322101423273906,
-2.5577732171851));
#66146=CARTESIAN_POINT('Ctrl Pts',(0.662800356661787,-0.432020223694912,
-2.56305392166118));
#66147=CARTESIAN_POINT('Ctrl Pts',(0.59115412975698,-0.541939024115916,
-2.56833462613726));
#66148=CARTESIAN_POINT('Ctrl Pts',(0.491575945729561,-0.633651481945187,
-2.57361533061333));
#66149=CARTESIAN_POINT('Ctrl Pts',(0.376146085946411,-0.696031542749064,
-2.57889603508941));
#66150=CARTESIAN_POINT('Ctrl Pts',(0.260716226163259,-0.758411603552943,
-2.58417673956549));
#66151=CARTESIAN_POINT('Ctrl Pts',(0.129434690624375,-0.791459267331427,
-2.58945744404157));
#66152=CARTESIAN_POINT('Ctrl Pts',(-0.00177216186859303,-0.791165372037872,
-2.59473814851765));
#66153=CARTESIAN_POINT('Ctrl Pts',(-0.132979014361561,-0.790871476744317,
-2.60001885299372));
#66154=CARTESIAN_POINT('Ctrl Pts',(-0.264111183808613,-0.757236022378723,
-2.6052995574698));
#66155=CARTESIAN_POINT('Ctrl Pts',(-0.379260431687407,-0.694339478522506,
-2.61058026194588));
#66156=CARTESIAN_POINT('Ctrl Pts',(-0.4944096795662,-0.631442934666289,
-2.61586096642196));
#66157=CARTESIAN_POINT('Ctrl Pts',(-0.593576005876736,-0.53928530131945,
-2.62114167089804));
#66158=CARTESIAN_POINT('Ctrl Pts',(-0.664729093579334,-0.429046639207677,
-2.62642237537412));
#66159=CARTESIAN_POINT('Ctrl Pts',(-0.735882181281933,-0.318807977095903,
-2.6317030798502));
#66160=CARTESIAN_POINT('Ctrl Pts',(-0.779022030376594,-0.190488286219194,
-2.63698378432627));
#66161=CARTESIAN_POINT('Ctrl Pts',(-0.78891515001337,-0.059654610495154,
-2.64226448880235));
#66162=CARTESIAN_POINT('Ctrl Pts',(-0.790415381576396,-0.0398144774497269,
-2.64306527559367));
#66163=CARTESIAN_POINT('Ctrl Pts',(-0.791151075266596,-0.019916533104998,
-2.64386606238498));
#66164=CARTESIAN_POINT('Ctrl Pts',(-0.791132110743512,-1.71897034488278E-5,
-2.6446668491763));
#66165=CARTESIAN_POINT('Ctrl Pts',(-0.791144428618858,-1.44065313715571E-5,
-2.6731331508237));
#66166=CARTESIAN_POINT('Ctrl Pts',(-0.791157447106144,-0.0154607415709918,
-2.67251153340796));
#66167=CARTESIAN_POINT('Ctrl Pts',(-0.790714316293819,-0.0309063302168789,
-2.67188991599221));
#66168=CARTESIAN_POINT('Ctrl Pts',(-0.7898099700181,-0.0463248671453487,
-2.67126829857647));
#66169=CARTESIAN_POINT('Ctrl Pts',(-0.782127454526808,-0.177306938931758,
-2.66598759410039));
#66170=CARTESIAN_POINT('Ctrl Pts',(-0.741160500133669,-0.306336775142769,
-2.66070688962431));
#66171=CARTESIAN_POINT('Ctrl Pts',(-0.671878993445302,-0.417761176977514,
-2.65542618514824));
#66172=CARTESIAN_POINT('Ctrl Pts',(-0.602597486756935,-0.529185578812257,
-2.65014548067216));
#66173=CARTESIAN_POINT('Ctrl Pts',(-0.50500142777334,-0.623004546270734,
-2.64486477619608));
#66174=CARTESIAN_POINT('Ctrl Pts',(-0.390930637547929,-0.687836476651132,
-2.63958407172));
#66175=CARTESIAN_POINT('Ctrl Pts',(-0.276859847322517,-0.752668407031531,
-2.63430336724392));
#66176=CARTESIAN_POINT('Ctrl Pts',(-0.146314325855289,-0.78851330033385,
-2.62902266276784));
#66177=CARTESIAN_POINT('Ctrl Pts',(-0.0151311426031084,-0.791022648891824,
-2.62374195829176));
#66178=CARTESIAN_POINT('Ctrl Pts',(0.116052040649072,-0.793531997449798,
-2.61846125381568));
#66179=CARTESIAN_POINT('Ctrl Pts',(0.247872885686205,-0.762705801263428,
-2.61318054933961));
#66180=CARTESIAN_POINT('Ctrl Pts',(0.364339607554318,-0.702283726586036,
-2.60789984486353));
#66181=CARTESIAN_POINT('Ctrl Pts',(0.48080632942243,-0.641861651908644,
-2.60261914038745));
#66182=CARTESIAN_POINT('Ctrl Pts',(0.581918928121522,-0.551843698740229,
-2.59733843591137));
#66183=CARTESIAN_POINT('Ctrl Pts',(0.655410975513677,-0.443150353199274,
-2.59205773143529));
#66184=CARTESIAN_POINT('Ctrl Pts',(0.72890302290583,-0.334457007658322,
-2.58677702695921));
#66185=CARTESIAN_POINT('Ctrl Pts',(0.774774518991048,-0.207088269744829,
-2.58149632248314));
#66186=CARTESIAN_POINT('Ctrl Pts',(0.787460584406806,-0.0764958191578642,
-2.57621561800706));
#66187=CARTESIAN_POINT('Ctrl Pts',(0.800146649822565,0.0540966314291024,
-2.57093491353098));
#66188=CARTESIAN_POINT('Ctrl Pts',(0.779647284568864,0.187912794689541,
-2.5656542090549));
#66189=CARTESIAN_POINT('Ctrl Pts',(0.728449359675282,0.308718824699482,
-2.56037350457882));
#66190=CARTESIAN_POINT('Ctrl Pts',(0.677251434781699,0.429524854709423,
-2.55509280010275));
#66191=CARTESIAN_POINT('Ctrl Pts',(0.595354950248236,0.537320751468866,
-2.54981209562667));
#66192=CARTESIAN_POINT('Ctrl Pts',(0.492695140236132,0.619029305554604,
-2.54453139115059));
#66193=CARTESIAN_POINT('Ctrl Pts',(0.39003533022403,0.700737859640341,-2.53925068667451));
#66194=CARTESIAN_POINT('Ctrl Pts',(0.266612194733288,0.756359071052374,
-2.53396998219843));
#66195=CARTESIAN_POINT('Ctrl Pts',(0.137398754398226,0.779145278255797,
-2.52868927772235));
#66196=CARTESIAN_POINT('Ctrl Pts',(0.0081853140631645,0.80193148545922,
-2.52340857324627));
#66197=CARTESIAN_POINT('Ctrl Pts',(-0.126818431116216,0.791882688454035,
-2.5181278687702));
#66198=CARTESIAN_POINT('Ctrl Pts',(-0.251234564197799,0.750217952395059,
-2.51284716429412));
#66199=CARTESIAN_POINT('Ctrl Pts',(-0.375650697279383,0.708553216336082,
-2.50756645981804));
#66200=CARTESIAN_POINT('Ctrl Pts',(-0.489479218263168,0.635272541223315,
-2.50228575534196));
#66201=CARTESIAN_POINT('Ctrl Pts',(-0.578911072740594,0.539265938289951,
-2.49700505086588));
#66202=CARTESIAN_POINT('Ctrl Pts',(-0.668342927218019,0.443259335356588,
-2.49172434638981));
#66203=CARTESIAN_POINT('Ctrl Pts',(-0.733378115189086,0.324526804602629,
-2.48644364191373));
#66204=CARTESIAN_POINT('Ctrl Pts',(-0.766126922886764,0.197472328112149,
-2.48116293743765));
#66205=CARTESIAN_POINT('Ctrl Pts',(-0.782726093121508,0.133073071082062,
-2.47848634189967));
#66206=CARTESIAN_POINT('Ctrl Pts',(-0.791030554834729,0.066535819218492,
-2.47580974636169));
#66207=CARTESIAN_POINT('Ctrl Pts',(-0.791033002877254,-8.32524903205056E-7,
-2.47313315082371));
#66208=CARTESIAN_POINT('Origin',(0.,0.,-1.425));
#66209=CARTESIAN_POINT('',(-0.791150917366707,1.23845276237822E-5,-2.2446668491763));
#66210=CARTESIAN_POINT('',(-0.791139629808145,1.56300862382004E-5,-2.27313315082371));
#66211=CARTESIAN_POINT('',(-0.7911,-9.68818082805471E-17,-1.425));
#66212=CARTESIAN_POINT('Ctrl Pts',(-0.791150917366707,1.23845276237822E-5,
-2.2446668491763));
#66213=CARTESIAN_POINT('Ctrl Pts',(-0.791160527113968,0.0128074960584554,
-2.24518178381636));
#66214=CARTESIAN_POINT('Ctrl Pts',(-0.790856504970953,0.0256021508212593,
-2.24569671845641));
#66215=CARTESIAN_POINT('Ctrl Pts',(-0.79023582091272,0.038381425446427,
-2.24621165309647));
#66216=CARTESIAN_POINT('Ctrl Pts',(-0.783870645937939,0.169434121195563,
-2.25149235757255));
#66217=CARTESIAN_POINT('Ctrl Pts',(-0.744203085343301,0.298869333913646,
-2.25677306204863));
#66218=CARTESIAN_POINT('Ctrl Pts',(-0.676045390906717,0.410984690598912,
-2.2620537665247));
#66219=CARTESIAN_POINT('Ctrl Pts',(-0.607887696470134,0.523100047284177,
-2.26733447100078));
#66220=CARTESIAN_POINT('Ctrl Pts',(-0.511239868191607,0.617895547936626,
-2.27261517547686));
#66221=CARTESIAN_POINT('Ctrl Pts',(-0.397826692685,0.683871120212145,-2.27789587995294));
#66222=CARTESIAN_POINT('Ctrl Pts',(-0.284413517178393,0.749846692487665,
-2.28317658442902));
#66223=CARTESIAN_POINT('Ctrl Pts',(-0.154234994443706,0.787002336386255,
-2.2884572889051));
#66224=CARTESIAN_POINT('Ctrl Pts',(-0.0230836717937855,0.790830532142896,
-2.29373799338118));
#66225=CARTESIAN_POINT('Ctrl Pts',(0.108067650856135,0.794658727899538,
-2.29901869785726));
#66226=CARTESIAN_POINT('Ctrl Pts',(0.24019177342129,0.765159475514229,-2.30429940233333));
#66227=CARTESIAN_POINT('Ctrl Pts',(0.357260119044719,0.705911463154589,
-2.30958010680941));
#66228=CARTESIAN_POINT('Ctrl Pts',(0.474328464668147,0.64666345079495,-2.31486081128549));
#66229=CARTESIAN_POINT('Ctrl Pts',(0.57634103334985,0.55766667846098,-2.32014151576157));
#66230=CARTESIAN_POINT('Ctrl Pts',(0.650922217473707,0.449717748451195,
-2.32542222023765));
#66231=CARTESIAN_POINT('Ctrl Pts',(0.725503401597566,0.341768818441408,
-2.33070292471373));
#66232=CARTESIAN_POINT('Ctrl Pts',(0.772653201163578,0.214867730755806,
-2.3359836291898));
#66233=CARTESIAN_POINT('Ctrl Pts',(0.786651660031553,0.0844094321891896,
-2.34126433366588));
#66234=CARTESIAN_POINT('Ctrl Pts',(0.800650118899528,-0.0460488663774256,
-2.34654503814196));
#66235=CARTESIAN_POINT('Ctrl Pts',(0.781497237069466,-0.180064375825055,
-2.35182574261804));
#66236=CARTESIAN_POINT('Ctrl Pts',(0.731516537547499,-0.30137906657135,
-2.35710644709412));
#66237=CARTESIAN_POINT('Ctrl Pts',(0.681535838025532,-0.422693757317647,
-2.3623871515702));
#66238=CARTESIAN_POINT('Ctrl Pts',(0.600727320811662,-0.531307629362611,
-2.36766785604627));
#66239=CARTESIAN_POINT('Ctrl Pts',(0.498894233819384,-0.614044241023943,
-2.37294856052235));
#66240=CARTESIAN_POINT('Ctrl Pts',(0.397061146827107,-0.696780852685274,
-2.37822926499843));
#66241=CARTESIAN_POINT('Ctrl Pts',(0.274203490056424,-0.753640203962973,
-2.38350996947451));
#66242=CARTESIAN_POINT('Ctrl Pts',(0.145225683349696,-0.777724428939013,
-2.38879067395059));
#66243=CARTESIAN_POINT('Ctrl Pts',(0.0162478766429679,-0.801808653915053,
-2.39407137842667));
#66244=CARTESIAN_POINT('Ctrl Pts',(-0.118850079999805,-0.793117752589433,
-2.39935208290275));
#66245=CARTESIAN_POINT('Ctrl Pts',(-0.243678840415138,-0.752706057639257,
-2.40463278737882));
#66246=CARTESIAN_POINT('Ctrl Pts',(-0.36850760083047,-0.712294362689082,
-2.4099134918549));
#66247=CARTESIAN_POINT('Ctrl Pts',(-0.483067165018363,-0.640161874114352,
-2.41519419633098));
#66248=CARTESIAN_POINT('Ctrl Pts',(-0.573459792402489,-0.545059311424541,
-2.42047490080706));
#66249=CARTESIAN_POINT('Ctrl Pts',(-0.663852419786615,-0.449956748734731,
-2.42575560528314));
#66250=CARTESIAN_POINT('Ctrl Pts',(-0.730078110366975,-0.331884111929841,
-2.43103630975922));
#66251=CARTESIAN_POINT('Ctrl Pts',(-0.764102725102462,-0.205165328366884,
-2.43631701423529));
#66252=CARTESIAN_POINT('Ctrl Pts',(-0.782035933210049,-0.138376201305743,
-2.43910029254896));
#66253=CARTESIAN_POINT('Ctrl Pts',(-0.791023738008576,-0.0691851895935175,
-2.44188357086263));
#66254=CARTESIAN_POINT('Ctrl Pts',(-0.79103374865932,3.27018256038314E-6,
-2.4446668491763));
#66255=CARTESIAN_POINT('Ctrl Pts',(-0.791033002877254,-8.32524903205056E-7,
-2.47313315082371));
#66256=CARTESIAN_POINT('Ctrl Pts',(-0.79103538462277,-0.0647355625419663,
-2.47052904188561));
#66257=CARTESIAN_POINT('Ctrl Pts',(-0.783179328184073,-0.129469724503196,
-2.46792493294751));
#66258=CARTESIAN_POINT('Ctrl Pts',(-0.767458105990247,-0.192233810480545,
-2.46532082400941));
#66259=CARTESIAN_POINT('Ctrl Pts',(-0.73557805397176,-0.319509050355758,
-2.46004011953334));
#66260=CARTESIAN_POINT('Ctrl Pts',(-0.671355522510494,-0.438683107879184,
-2.45475941505726));
#66261=CARTESIAN_POINT('Ctrl Pts',(-0.582581638325029,-0.535298437349069,
-2.44947871058118));
#66262=CARTESIAN_POINT('Ctrl Pts',(-0.493807754139564,-0.631913766818955,
-2.4441980061051));
#66263=CARTESIAN_POINT('Ctrl Pts',(-0.380482517229898,-0.705970368235301,
-2.43891730162902));
#66264=CARTESIAN_POINT('Ctrl Pts',(-0.256353926329107,-0.748484099228321,
-2.43363659715294));
#66265=CARTESIAN_POINT('Ctrl Pts',(-0.132225335428317,-0.790997830221342,
-2.42835589267686));
#66266=CARTESIAN_POINT('Ctrl Pts',(0.00270660946359702,-0.801968690791038,
-2.42307518820079));
#66267=CARTESIAN_POINT('Ctrl Pts',(0.132072701821953,-0.780065756058642,
-2.41779448372471));
#66268=CARTESIAN_POINT('Ctrl Pts',(0.261438794180308,-0.758162821326247,
-2.41251377924863));
#66269=CARTESIAN_POINT('Ctrl Pts',(0.385239034005103,-0.703386091291759,
-2.40723307477255));
#66270=CARTESIAN_POINT('Ctrl Pts',(0.488454652426469,-0.622380779639659,
-2.40195237029647));
#66271=CARTESIAN_POINT('Ctrl Pts',(0.591670270847835,-0.541375467987559,
-2.39667166582039));
#66272=CARTESIAN_POINT('Ctrl Pts',(0.674301267865773,-0.434141574717848,
-2.39139096134431));
#66273=CARTESIAN_POINT('Ctrl Pts',(0.726323302271758,-0.313688130025617,
-2.38611025686824));
#66274=CARTESIAN_POINT('Ctrl Pts',(0.778345336677742,-0.193234685333386,
-2.38082955239216));
#66275=CARTESIAN_POINT('Ctrl Pts',(0.799758408471774,-0.0595616892186328,
-2.37554884791608));
#66276=CARTESIAN_POINT('Ctrl Pts',(0.787964800746976,0.0711143805829716,
-2.37026814344));
#66277=CARTESIAN_POINT('Ctrl Pts',(0.776171193022177,0.201790450384576,
-2.36498743896392));
#66278=CARTESIAN_POINT('Ctrl Pts',(0.731170905778547,0.329469593873033,
-2.35970673448784));
#66279=CARTESIAN_POINT('Ctrl Pts',(0.658423128062463,0.438662474773447,
-2.35442603001176));
#66280=CARTESIAN_POINT('Ctrl Pts',(0.585675350346377,0.547855355673862,
-2.34914532553569));
#66281=CARTESIAN_POINT('Ctrl Pts',(0.485180082157836,0.638561973986235,
-2.34386462105961));
#66282=CARTESIAN_POINT('Ctrl Pts',(0.369128860504978,0.699778298237532,
-2.33858391658353));
#66283=CARTESIAN_POINT('Ctrl Pts',(0.253077638852122,0.760994622488829,
-2.33330321210745));
#66284=CARTESIAN_POINT('Ctrl Pts',(0.121470463734948,0.79272065267905,-2.32802250763137));
#66285=CARTESIAN_POINT('Ctrl Pts',(-0.00972680123028606,0.791107560120461,
-2.32274180315529));
#66286=CARTESIAN_POINT('Ctrl Pts',(-0.140924066195523,0.789494467561872,
-2.31746109867922));
#66287=CARTESIAN_POINT('Ctrl Pts',(-0.271711421008817,0.754542252254472,
-2.31218039420314));
#66288=CARTESIAN_POINT('Ctrl Pts',(-0.386222458175134,0.690491126042238,
-2.30689968972706));
#66289=CARTESIAN_POINT('Ctrl Pts',(-0.500733495341449,0.626439999830005,
-2.30161898525098));
#66290=CARTESIAN_POINT('Ctrl Pts',(-0.598968214860784,0.533289962712938,
-2.2963382807749));
#66291=CARTESIAN_POINT('Ctrl Pts',(-0.669009317141909,0.422341468386942,
-2.29105757629882));
#66292=CARTESIAN_POINT('Ctrl Pts',(-0.739050419423034,0.311392974060945,
-2.28577687182274));
#66293=CARTESIAN_POINT('Ctrl Pts',(-0.780897904465948,0.182646022526017,
-2.28049616734667));
#66294=CARTESIAN_POINT('Ctrl Pts',(-0.789475063965926,0.0517194906966256,
-2.27521546287059));
#66295=CARTESIAN_POINT('Ctrl Pts',(-0.79060245916075,0.0345103035689084,
-2.27452135885496));
#66296=CARTESIAN_POINT('Ctrl Pts',(-0.791155046841484,0.0172634600879581,
-2.27382725483933));
#66297=CARTESIAN_POINT('Ctrl Pts',(-0.791139629808145,1.56300862382004E-5,
-2.27313315082371));
#66298=CARTESIAN_POINT('Origin',(0.,0.,-1.425));
#66299=CARTESIAN_POINT('',(-0.791081097997334,-1.97830511448061E-5,-2.0446668491763));
#66300=CARTESIAN_POINT('',(-0.791094572033932,-2.03193093578051E-5,-2.07313315082371));
#66301=CARTESIAN_POINT('',(-0.7911,-9.68818082805471E-17,-1.425));
#66302=CARTESIAN_POINT('Ctrl Pts',(-0.791081097997334,-1.9783051144806E-5,
-2.0446668491763));
#66303=CARTESIAN_POINT('Ctrl Pts',(-0.790990817900606,0.0947535438784193,
-2.04847999677008));
#66304=CARTESIAN_POINT('Ctrl Pts',(-0.773944248118208,0.189558474775009,
-2.05229314436386));
#66305=CARTESIAN_POINT('Ctrl Pts',(-0.740623479673775,0.278249254857598,
-2.05610629195765));
#66306=CARTESIAN_POINT('Ctrl Pts',(-0.69447862775203,0.401074240738709,
-2.06138699643373));
#66307=CARTESIAN_POINT('Ctrl Pts',(-0.617122170298751,0.512173152277855,
-2.0666677009098));
#66308=CARTESIAN_POINT('Ctrl Pts',(-0.51793857019323,0.598068076375167,
-2.07194840538588));
#66309=CARTESIAN_POINT('Ctrl Pts',(-0.41875497008771,0.683963000472479,
-2.07722910986196));
#66310=CARTESIAN_POINT('Ctrl Pts',(-0.297744227329949,0.744653937127956,
-2.08250981433804));
#66311=CARTESIAN_POINT('Ctrl Pts',(-0.169586704242536,0.772778193414549,
-2.08779051881412));
#66312=CARTESIAN_POINT('Ctrl Pts',(-0.0414291811551249,0.800902449701142,
-2.0930712232902));
#66313=CARTESIAN_POINT('Ctrl Pts',(0.0938751222619378,0.796460025618851,
-2.09835192776627));
#66314=CARTESIAN_POINT('Ctrl Pts',(0.219911826981627,0.759989851791787,
-2.10363263224235));
#66315=CARTESIAN_POINT('Ctrl Pts',(0.345948531701318,0.723519677964723,
-2.10891333671843));
#66316=CARTESIAN_POINT('Ctrl Pts',(0.462717637723634,0.655021754392886,
-2.11419404119451));
#66317=CARTESIAN_POINT('Ctrl Pts',(0.556053354925926,0.562805875012443,
-2.11947474567059));
#66318=CARTESIAN_POINT('Ctrl Pts',(0.649389072128219,0.470589995632,-2.12475545014667));
#66319=CARTESIAN_POINT('Ctrl Pts',(0.719291400510487,0.354656160442951,
-2.13003615462275));
#66320=CARTESIAN_POINT('Ctrl Pts',(0.757280171416149,0.229068829072896,
-2.13531685909882));
#66321=CARTESIAN_POINT('Ctrl Pts',(0.79526894232181,0.103481497702842,-2.1405975635749));
#66322=CARTESIAN_POINT('Ctrl Pts',(0.801344155750865,-0.0317593298482181,
-2.14587826805098));
#66323=CARTESIAN_POINT('Ctrl Pts',(0.774768799994326,-0.160246975098601,
-2.15115897252706));
#66324=CARTESIAN_POINT('Ctrl Pts',(0.748193444237787,-0.288734620348983,
-2.15643967700314));
#66325=CARTESIAN_POINT('Ctrl Pts',(0.688967519295655,-0.410469083298688,
-2.16172038147922));
#66326=CARTESIAN_POINT('Ctrl Pts',(0.604275990876151,-0.510682203844568,
-2.1670010859553));
#66327=CARTESIAN_POINT('Ctrl Pts',(0.519584462456648,-0.610895324390448,
-2.17228179043137));
#66328=CARTESIAN_POINT('Ctrl Pts',(0.409427330559771,-0.689587102532504,
-2.17756249490745));
#66329=CARTESIAN_POINT('Ctrl Pts',(0.287168256723413,-0.737211081579309,
-2.18284319938353));
#66330=CARTESIAN_POINT('Ctrl Pts',(0.164909182887057,-0.784835060626115,
-2.18812390385961));
#66331=CARTESIAN_POINT('Ctrl Pts',(0.0305481671112177,-0.801391240577672,
-2.19340460833569));
#66332=CARTESIAN_POINT('Ctrl Pts',(-0.0996148460812547,-0.784871116115957,
-2.19868531281176));
#66333=CARTESIAN_POINT('Ctrl Pts',(-0.229777859273729,-0.768350991654242,
-2.20396601728784));
#66334=CARTESIAN_POINT('Ctrl Pts',(-0.355742869882836,-0.718754562779255,
-2.20924672176392));
#66335=CARTESIAN_POINT('Ctrl Pts',(-0.462228490871624,-0.642098597334895,
-2.21452742624));
#66336=CARTESIAN_POINT('Ctrl Pts',(-0.568714111860411,-0.565442631890537,
-2.21980813071608));
#66337=CARTESIAN_POINT('Ctrl Pts',(-0.65572034322888,-0.461727129876807,
-2.22508883519216));
#66338=CARTESIAN_POINT('Ctrl Pts',(-0.712692064235652,-0.343534289479849,
-2.23036953966824));
#66339=CARTESIAN_POINT('Ctrl Pts',(-0.764108330892919,-0.236866727197373,
-2.23513530950426));
#66340=CARTESIAN_POINT('Ctrl Pts',(-0.791061978227509,-0.118407608688093,
-2.23990107934028));
#66341=CARTESIAN_POINT('Ctrl Pts',(-0.791150917366707,1.23845276237822E-5,
-2.2446668491763));
#66342=CARTESIAN_POINT('Ctrl Pts',(-0.791139629808145,1.56300862382004E-5,
-2.27313315082371));
#66343=CARTESIAN_POINT('Ctrl Pts',(-0.791037754915302,-0.113957064562566,
-2.26854655036325));
#66344=CARTESIAN_POINT('Ctrl Pts',(-0.766133997457558,-0.227972835565614,
-2.2639599499028));
#66345=CARTESIAN_POINT('Ctrl Pts',(-0.718391205861583,-0.331451139208576,
-2.25937334944235));
#66346=CARTESIAN_POINT('Ctrl Pts',(-0.663423354300215,-0.450589125160531,
-2.25409264496627));
#66347=CARTESIAN_POINT('Ctrl Pts',(-0.578180817220436,-0.555758984940586,
-2.2488119404902));
#66348=CARTESIAN_POINT('Ctrl Pts',(-0.473004753606229,-0.634202085622424,
-2.24353123601412));
#66349=CARTESIAN_POINT('Ctrl Pts',(-0.367828689992021,-0.712645186304262,
-2.23825053153804));
#66350=CARTESIAN_POINT('Ctrl Pts',(-0.242719099843387,-0.764361527887883,
-2.23296982706196));
#66351=CARTESIAN_POINT('Ctrl Pts',(-0.112853595259514,-0.783077166299033,
-2.22768912258588));
#66352=CARTESIAN_POINT('Ctrl Pts',(0.0170119093243585,-0.801792804710183,
-2.22240841810981));
#66353=CARTESIAN_POINT('Ctrl Pts',(0.151633328343468,-0.787507739948862,
-2.21712771363373));
#66354=CARTESIAN_POINT('Ctrl Pts',(0.274679126575874,-0.741954958043571,
-2.21184700915765));
#66355=CARTESIAN_POINT('Ctrl Pts',(0.397724924808278,-0.69640217613828,
-2.20656630468157));
#66356=CARTESIAN_POINT('Ctrl Pts',(0.509195102253979,-0.619581677089019,
-2.20128560020549));
#66357=CARTESIAN_POINT('Ctrl Pts',(0.595566705861264,-0.520812904229037,
-2.19600489572941));
#66358=CARTESIAN_POINT('Ctrl Pts',(0.681938309468549,-0.422044131369055,
-2.19072419125333));
#66359=CARTESIAN_POINT('Ctrl Pts',(0.743211339237417,-0.30132708469835,
-2.18544348677726));
#66360=CARTESIAN_POINT('Ctrl Pts',(0.77195248588383,-0.173306496934467,
-2.18016278230118));
#66361=CARTESIAN_POINT('Ctrl Pts',(0.800693632530243,-0.0452859091705829,
-2.1748820778251));
#66362=CARTESIAN_POINT('Ctrl Pts',(0.7969028960542,0.0900382196864831,-2.16960137334902));
#66363=CARTESIAN_POINT('Ctrl Pts',(0.761040147899091,0.216249105495609,
-2.16432066887294));
#66364=CARTESIAN_POINT('Ctrl Pts',(0.725177399743983,0.342459991304734,
-2.15903996439686));
#66365=CARTESIAN_POINT('Ctrl Pts',(0.65724263990981,0.45955763406592,-2.15375925992079));
#66366=CARTESIAN_POINT('Ctrl Pts',(0.565477342384216,0.553336387373906,
-2.14847855544471));
#66367=CARTESIAN_POINT('Ctrl Pts',(0.473712044858623,0.647115140681891,
-2.14319785096863));
#66368=CARTESIAN_POINT('Ctrl Pts',(0.358116209641609,0.717575004536675,
-2.13791714649255));
#66369=CARTESIAN_POINT('Ctrl Pts',(0.232713292050402,0.756168173123536,
-2.13263644201647));
#66370=CARTESIAN_POINT('Ctrl Pts',(0.107310374459195,0.794761341710397,
-2.12735573754039));
#66371=CARTESIAN_POINT('Ctrl Pts',(-0.0278996255061993,0.801487815029334,
-2.12207503306431));
#66372=CARTESIAN_POINT('Ctrl Pts',(-0.156513769198413,0.775531574078856,
-2.11679432858824));
#66373=CARTESIAN_POINT('Ctrl Pts',(-0.285127912890625,0.749575333128377,
-2.11151362411216));
#66374=CARTESIAN_POINT('Ctrl Pts',(-0.407146200309654,0.690936377908482,
-2.10623291963608));
#66375=CARTESIAN_POINT('Ctrl Pts',(-0.507766039318046,0.606728466166857,
-2.10095221516));
#66376=CARTESIAN_POINT('Ctrl Pts',(-0.60838587832644,0.522520554425229,
-2.09567151068392));
#66377=CARTESIAN_POINT('Ctrl Pts',(-0.687607268924199,0.412743686161869,
-2.09039080620784));
#66378=CARTESIAN_POINT('Ctrl Pts',(-0.735819504729637,0.290715391407736,
-2.08511010173177));
#66379=CARTESIAN_POINT('Ctrl Pts',(-0.772268908025816,0.198459588399807,
-2.08111778476241));
#66380=CARTESIAN_POINT('Ctrl Pts',(-0.790994536208493,0.0992012879231028,
-2.07712546779306));
#66381=CARTESIAN_POINT('Ctrl Pts',(-0.791094572033932,-2.03193093578051E-5,
-2.07313315082371));
#66382=CARTESIAN_POINT('Origin',(0.,0.,-1.425));
#66383=CARTESIAN_POINT('',(-0.791057251695019,1.61679271216408E-5,-1.8446668491763));
#66384=CARTESIAN_POINT('',(-0.79104797996428,1.33236467988428E-5,-1.87313315082371));
#66385=CARTESIAN_POINT('',(-0.7911,-9.68818082805471E-17,-1.425));
#66386=CARTESIAN_POINT('Ctrl Pts',(-0.791057251695019,1.61679271216408E-5,
-1.8446668491763));
#66387=CARTESIAN_POINT('Ctrl Pts',(-0.791091088198568,0.0455198809875166,
-1.84649750524773));
#66388=CARTESIAN_POINT('Ctrl Pts',(-0.787229605616998,0.0910179144373288,
-1.84832816131916));
#66389=CARTESIAN_POINT('Ctrl Pts',(-0.779420639490756,0.135828028067558,
-1.85015881739059));
#66390=CARTESIAN_POINT('Ctrl Pts',(-0.756894921514591,0.265087134304733,
-1.85543952186667));
#66391=CARTESIAN_POINT('Ctrl Pts',(-0.701522594957182,0.388622129777778,
-1.86072022634275));
#66392=CARTESIAN_POINT('Ctrl Pts',(-0.620021128019969,0.491446423612732,
-1.86600093081882));
#66393=CARTESIAN_POINT('Ctrl Pts',(-0.538519661082756,0.594270717447687,
-1.8712816352949));
#66394=CARTESIAN_POINT('Ctrl Pts',(-0.430889053765737,0.676384309644556,
-1.87656233977098));
#66395=CARTESIAN_POINT('Ctrl Pts',(-0.310186463445237,0.727825627721529,
-1.88184304424706));
#66396=CARTESIAN_POINT('Ctrl Pts',(-0.18948387312474,0.7792669457985,-1.88712374872314));
#66397=CARTESIAN_POINT('Ctrl Pts',(-0.0557092998007569,0.800035989755576,
-1.89240445319922));
#66398=CARTESIAN_POINT('Ctrl Pts',(0.0749084559988265,0.787613172625225,
-1.8976851576753));
#66399=CARTESIAN_POINT('Ctrl Pts',(0.205526211798415,0.775190355494874,
-1.90296586215137));
#66400=CARTESIAN_POINT('Ctrl Pts',(0.332987150073606,0.729575677277096,
-1.90824656662745));
#66401=CARTESIAN_POINT('Ctrl Pts',(0.44182840601411,0.656302861575303,-1.91352727110353));
#66402=CARTESIAN_POINT('Ctrl Pts',(0.550669661954614,0.58303004587351,-1.91880797557961));
#66403=CARTESIAN_POINT('Ctrl Pts',(0.640891235560426,0.482099092687703,
-1.92408868005569));
#66404=CARTESIAN_POINT('Ctrl Pts',(0.70154793833288,0.365754393950074,-1.92936938453177));
#66405=CARTESIAN_POINT('Ctrl Pts',(0.762204641105332,0.249409695212449,
-1.93465008900784));
#66406=CARTESIAN_POINT('Ctrl Pts',(0.793296473044426,0.117651250923005,
-1.93993079348392));
#66407=CARTESIAN_POINT('Ctrl Pts',(0.791051542930121,-0.01353672415229,
-1.94521149796));
#66408=CARTESIAN_POINT('Ctrl Pts',(0.788806612815815,-0.144724699227588,
-1.95049220243608));
#66409=CARTESIAN_POINT('Ctrl Pts',(0.753224920648107,-0.275342205088737,
-1.95577290691216));
#66410=CARTESIAN_POINT('Ctrl Pts',(0.688623042965317,-0.389543439387815,
-1.96105361138824));
#66411=CARTESIAN_POINT('Ctrl Pts',(0.624021165282528,-0.503744673686888,
-1.96633431586431));
#66412=CARTESIAN_POINT('Ctrl Pts',(0.530399102084659,-0.601529636423893,
-1.97161502034039));
#66413=CARTESIAN_POINT('Ctrl Pts',(0.419114570693421,-0.671035590043754,
-1.97689572481647));
#66414=CARTESIAN_POINT('Ctrl Pts',(0.30783003930218,-0.740541543663617,
-1.98217642929255));
#66415=CARTESIAN_POINT('Ctrl Pts',(0.178883039717568,-0.781768488166335,
-1.98745713376863));
#66416=CARTESIAN_POINT('Ctrl Pts',(0.0479167175907291,-0.789714995835985,
-1.99273783824471));
#66417=CARTESIAN_POINT('Ctrl Pts',(-0.0830496045361099,-0.797661503505635,
-1.99801854272078));
#66418=CARTESIAN_POINT('Ctrl Pts',(-0.216035249205176,-0.772327574342217,
-2.00329924719686));
#66419=CARTESIAN_POINT('Ctrl Pts',(-0.334907124403696,-0.716786582252031,
-2.00857995167294));
#66420=CARTESIAN_POINT('Ctrl Pts',(-0.453778999602217,-0.661245590161845,
-2.01386065614902));
#66421=CARTESIAN_POINT('Ctrl Pts',(-0.558537105330192,-0.575497535144891,
-2.0191413606251));
#66422=CARTESIAN_POINT('Ctrl Pts',(-0.636472760413809,-0.469944902860034,
-2.02442206510118));
#66423=CARTESIAN_POINT('Ctrl Pts',(-0.714408415497425,-0.364392270575176,
-2.02970276957726));
#66424=CARTESIAN_POINT('Ctrl Pts',(-0.765521619936684,-0.239035061022416,
-2.03498347405333));
#66425=CARTESIAN_POINT('Ctrl Pts',(-0.783611598961207,-0.109080926134498,
-2.04026417852941));
#66426=CARTESIAN_POINT('Ctrl Pts',(-0.788638972361532,-0.0729654635288157,
-2.04173173541171));
#66427=CARTESIAN_POINT('Ctrl Pts',(-0.791115843879582,-0.0364949639280258,
-2.043199292294));
#66428=CARTESIAN_POINT('Ctrl Pts',(-0.791081097997334,-1.9783051144806E-5,
-2.0446668491763));
#66429=CARTESIAN_POINT('Ctrl Pts',(-0.791094572033932,-2.03193093578051E-5,
-2.07313315082371));
#66430=CARTESIAN_POINT('Ctrl Pts',(-0.791126855269133,-0.0320407926677618,
-2.07184476331698));
#66431=CARTESIAN_POINT('Ctrl Pts',(-0.789219355838881,-0.0640574445681548,
-2.07055637581026));
#66432=CARTESIAN_POINT('Ctrl Pts',(-0.785341763947706,-0.0958336900125776,
-2.06926798830353));
#66433=CARTESIAN_POINT('Ctrl Pts',(-0.769448706347217,-0.226074755433851,
-2.06398728382745));
#66434=CARTESIAN_POINT('Ctrl Pts',(-0.720459510133122,-0.352277165031491,
-2.05870657935137));
#66435=CARTESIAN_POINT('Ctrl Pts',(-0.644317276999745,-0.459130731819986,
-2.05342587487529));
#66436=CARTESIAN_POINT('Ctrl Pts',(-0.568175043866367,-0.565984298608481,
-2.04814517039922));
#66437=CARTESIAN_POINT('Ctrl Pts',(-0.464879773813709,-0.65348902258783,
-2.04286446592314));
#66438=CARTESIAN_POINT('Ctrl Pts',(-0.346962684781801,-0.711029308615985,
-2.03758376144706));
#66439=CARTESIAN_POINT('Ctrl Pts',(-0.229045595749893,-0.768569594644141,
-2.03230305697098));
#66440=CARTESIAN_POINT('Ctrl Pts',(-0.0965066877387357,-0.796145442721103,
-2.0270223524949));
#66441=CARTESIAN_POINT('Ctrl Pts',(0.0345751428900571,-0.790411501583861,
-2.02174164801882));
#66442=CARTESIAN_POINT('Ctrl Pts',(0.16565697351885,-0.784677560446619,
-2.01646094354275));
#66443=CARTESIAN_POINT('Ctrl Pts',(0.295281726765278,-0.745633830095173,
-2.01118023906667));
#66444=CARTESIAN_POINT('Ctrl Pts',(0.407724035605994,-0.678016882629838,
-2.00589953459059));
#66445=CARTESIAN_POINT('Ctrl Pts',(0.520166344446709,-0.610399935164503,
-2.00061883011451));
#66446=CARTESIAN_POINT('Ctrl Pts',(0.615426208881714,-0.514209770585277,
-1.99533812563843));
#66447=CARTESIAN_POINT('Ctrl Pts',(0.681947222489256,-0.401115654245894,
-1.99005742116235));
#66448=CARTESIAN_POINT('Ctrl Pts',(0.748468236096796,-0.288021537906514,
-1.98477671668627));
#66449=CARTESIAN_POINT('Ctrl Pts',(0.786250398876875,-0.158023469806975,
-1.9794960122102));
#66450=CARTESIAN_POINT('Ctrl Pts',(0.790710185215964,-0.0268921054894726,
-1.97421530773412));
#66451=CARTESIAN_POINT('Ctrl Pts',(0.795169971555054,0.104239258828034,
-1.96893460325804));
#66452=CARTESIAN_POINT('Ctrl Pts',(0.76630738145315,0.236503919363504,-1.96365389878196));
#66453=CARTESIAN_POINT('Ctrl Pts',(0.707623866687246,0.353856249961072,
-1.95837319430588));
#66454=CARTESIAN_POINT('Ctrl Pts',(0.648940351921342,0.471208580558639,
-1.9530924898298));
#66455=CARTESIAN_POINT('Ctrl Pts',(0.560435912491437,0.573648581218303,
-1.94781178535373));
#66456=CARTESIAN_POINT('Ctrl Pts',(0.452847423557364,0.648748790611111,
-1.94253108087765));
#66457=CARTESIAN_POINT('Ctrl Pts',(0.34525893462329,0.723849000003919,-1.93725037640157));
#66458=CARTESIAN_POINT('Ctrl Pts',(0.218586396185047,0.77160941812987,-1.93196967192549));
#66459=CARTESIAN_POINT('Ctrl Pts',(0.0881970286911367,0.78623601194042,
-1.92668896744941));
#66460=CARTESIAN_POINT('Ctrl Pts',(-0.0421923388027758,0.800862605750971,
-1.92140826297333));
#66461=CARTESIAN_POINT('Ctrl Pts',(-0.176298535352356,0.78235537524612,
-1.91612755849726));
#66462=CARTESIAN_POINT('Ctrl Pts',(-0.297852529711402,0.732959516539925,
-1.91084685402118));
#66463=CARTESIAN_POINT('Ctrl Pts',(-0.419406524070446,0.68356365783373,
-1.9055661495451));
#66464=CARTESIAN_POINT('Ctrl Pts',(-0.528408316238956,0.603279170926192,
-1.90028544506902));
#66465=CARTESIAN_POINT('Ctrl Pts',(-0.611634404184154,0.501845731236419,
-1.89500474059294));
#66466=CARTESIAN_POINT('Ctrl Pts',(-0.69486049212935,0.400412291546648,
-1.88972403611686));
#66467=CARTESIAN_POINT('Ctrl Pts',(-0.752310875851237,0.277829899074643,
-1.88444333164079));
#66468=CARTESIAN_POINT('Ctrl Pts',(-0.777015988604014,0.148969580101607,
-1.87916262716471));
#66469=CARTESIAN_POINT('Ctrl Pts',(-0.786418704568611,0.0999256032318913,
-1.87715280171771));
#66470=CARTESIAN_POINT('Ctrl Pts',(-0.791078110168372,0.0499722384426156,
-1.87514297627071));
#66471=CARTESIAN_POINT('Ctrl Pts',(-0.79104797996428,1.33236467988428E-5,
-1.87313315082371));
#66472=CARTESIAN_POINT('Origin',(0.,0.,-1.425));
#66473=CARTESIAN_POINT('',(-0.791165709393907,-3.94338443360231E-6,-1.6446668491763));
#66474=CARTESIAN_POINT('',(-0.791167324336245,7.15608088368358E-7,-1.6731331508237));
#66475=CARTESIAN_POINT('',(-0.7911,-9.68818082805471E-17,-1.425));
#66476=CARTESIAN_POINT('Ctrl Pts',(-0.791165709393907,-3.94338443360232E-6,
-1.6446668491763));
#66477=CARTESIAN_POINT('Ctrl Pts',(-0.791130303728021,0.127431427810519,
-1.64979571820145));
#66478=CARTESIAN_POINT('Ctrl Pts',(-0.759749767008419,0.254883610031654,
-1.65492458722661));
#66479=CARTESIAN_POINT('Ctrl Pts',(-0.700520896362271,0.367717636553784,
-1.66005345625176));
#66480=CARTESIAN_POINT('Ctrl Pts',(-0.639538609468196,0.483892010667631,
-1.66533416072784));
#66481=CARTESIAN_POINT('Ctrl Pts',(-0.549034733691348,0.584569903594896,
-1.67061486520392));
#66482=CARTESIAN_POINT('Ctrl Pts',(-0.439988704887787,0.657537623291678,
-1.67589556968));
#66483=CARTESIAN_POINT('Ctrl Pts',(-0.330942676084231,0.730505342988456,
-1.68117627415608));
#66484=CARTESIAN_POINT('Ctrl Pts',(-0.203354494253961,0.775762889454755,
-1.68645697863216));
#66485=CARTESIAN_POINT('Ctrl Pts',(-0.0727024607003433,0.787819864360512,
-1.69173768310824));
#66486=CARTESIAN_POINT('Ctrl Pts',(0.0579495728532782,0.79987683926627,
-1.69701838758431));
#66487=CARTESIAN_POINT('Ctrl Pts',(0.191665458130249,0.778733242611484,
-1.70229909206039));
#66488=CARTESIAN_POINT('Ctrl Pts',(0.312223514315988,0.726954100051079,
-1.70757979653647));
#66489=CARTESIAN_POINT('Ctrl Pts',(0.432781570501728,0.675174957490674,
-1.71286050101255));
#66490=CARTESIAN_POINT('Ctrl Pts',(0.540181797596237,0.592760269024648,
-1.71814120548863));
#66491=CARTESIAN_POINT('Ctrl Pts',(0.621394986693395,0.48970813448953,-1.72342190996471));
#66492=CARTESIAN_POINT('Ctrl Pts',(0.702608175790553,0.386655999954413,
-1.72870261444078));
#66493=CARTESIAN_POINT('Ctrl Pts',(0.75763432689036,0.262966419350202,-1.73398331891686));
#66494=CARTESIAN_POINT('Ctrl Pts',(0.779797967907005,0.133644736974585,
-1.73926402339294));
#66495=CARTESIAN_POINT('Ctrl Pts',(0.80196160892365,0.00432305459896595,
-1.74454472786902));
#66496=CARTESIAN_POINT('Ctrl Pts',(0.791262739857134,-0.130630729548055,
-1.7498254323451));
#66497=CARTESIAN_POINT('Ctrl Pts',(0.748999289062897,-0.254844759522685,
-1.75510613682118));
#66498=CARTESIAN_POINT('Ctrl Pts',(0.706735838268662,-0.379058789497312,
-1.76038684129725));
#66499=CARTESIAN_POINT('Ctrl Pts',(0.632907805746706,-0.492533065299543,
-1.76566754577333));
#66500=CARTESIAN_POINT('Ctrl Pts',(0.536471605136735,-0.581501507611902,
-1.77094825024941));
#66501=CARTESIAN_POINT('Ctrl Pts',(0.440035404526762,-0.670469949924263,
-1.77622895472549));
#66502=CARTESIAN_POINT('Ctrl Pts',(0.320991035828772,-0.734932558746751,
-1.78150965920157));
#66503=CARTESIAN_POINT('Ctrl Pts',(0.193780311605213,-0.767069082486765,
-1.78679036367765));
#66504=CARTESIAN_POINT('Ctrl Pts',(0.0665695873816547,-0.799205606226778,
-1.79207106815373));
#66505=CARTESIAN_POINT('Ctrl Pts',(-0.0688074923674732,-0.799016044884316,
-1.7973517726298));
#66506=CARTESIAN_POINT('Ctrl Pts',(-0.195927719788058,-0.766523395006019,
-1.80263247710588));
#66507=CARTESIAN_POINT('Ctrl Pts',(-0.32304794720864,-0.734030745127722,
-1.80791318158196));
#66508=CARTESIAN_POINT('Ctrl Pts',(-0.441911322300681,-0.66923500671359,
-1.81319388605804));
#66509=CARTESIAN_POINT('Ctrl Pts',(-0.538097989657374,-0.579996844818653,
-1.81847459053412));
#66510=CARTESIAN_POINT('Ctrl Pts',(-0.63428465701407,-0.490758682923715,
-1.8237552950102));
#66511=CARTESIAN_POINT('Ctrl Pts',(-0.707794616635418,-0.37707809754797,
-1.82903599948627));
#66512=CARTESIAN_POINT('Ctrl Pts',(-0.749710041748631,-0.252746196359444,
-1.83431670396235));
#66513=CARTESIAN_POINT('Ctrl Pts',(-0.777094692072668,-0.171516299991357,
-1.837766752367));
#66514=CARTESIAN_POINT('Ctrl Pts',(-0.790993483531841,-0.0857399798821861,
-1.84121680077165));
#66515=CARTESIAN_POINT('Ctrl Pts',(-0.791057251695019,1.61679271216408E-5,
-1.8446668491763));
#66516=CARTESIAN_POINT('Ctrl Pts',(-0.79104797996428,1.33236467988428E-5,
-1.87313315082371));
#66517=CARTESIAN_POINT('Ctrl Pts',(-0.790998944734453,-0.0812920289971471,
-1.86986227179463));
#66518=CARTESIAN_POINT('Ctrl Pts',(-0.778529321983252,-0.162612081249939,
-1.86659139276555));
#66519=CARTESIAN_POINT('Ctrl Pts',(-0.753870902032603,-0.240050922536179,
-1.86332051373647));
#66520=CARTESIAN_POINT('Ctrl Pts',(-0.714060860924751,-0.365072860726848,
-1.85803980926039));
#66521=CARTESIAN_POINT('Ctrl Pts',(-0.642480936925383,-0.479978491634118,
-1.85275910478431));
#66522=CARTESIAN_POINT('Ctrl Pts',(-0.547814815427932,-0.570828091757565,
-1.84747840030824));
#66523=CARTESIAN_POINT('Ctrl Pts',(-0.45314869393048,-0.661677691881011,
-1.84219769583216));
#66524=CARTESIAN_POINT('Ctrl Pts',(-0.335396374934945,-0.728471261220633,
-1.83691699135608));
#66525=CARTESIAN_POINT('Ctrl Pts',(-0.208842926591348,-0.763105768786138,
-1.83163628688));
#66526=CARTESIAN_POINT('Ctrl Pts',(-0.0822894782477499,-0.797740276351643,
-1.82635558240392));
#66527=CARTESIAN_POINT('Ctrl Pts',(0.0530650994439101,-0.80021572214303,
-1.82107487792784));
#66528=CARTESIAN_POINT('Ctrl Pts',(0.180800328456221,-0.770231798598347,
-1.81579417345177));
#66529=CARTESIAN_POINT('Ctrl Pts',(0.308535557468532,-0.740247875053664,
-1.81051346897569));
#66530=CARTESIAN_POINT('Ctrl Pts',(0.428651437801493,-0.677804582172911,
-1.80523276449961));
#66531=CARTESIAN_POINT('Ctrl Pts',(0.526576166953947,-0.590477199168613,
-1.79995206002353));
#66532=CARTESIAN_POINT('Ctrl Pts',(0.624500896106401,-0.503149816164315,
-1.79467135554745));
#66533=CARTESIAN_POINT('Ctrl Pts',(0.700234474078348,-0.390938343036472,
-1.78939065107137));
#66534=CARTESIAN_POINT('Ctrl Pts',(0.744589316864623,-0.267455662779823,
-1.78410994659529));
#66535=CARTESIAN_POINT('Ctrl Pts',(0.788944159650899,-0.143972982523175,
-1.77882924211922));
#66536=CARTESIAN_POINT('Ctrl Pts',(0.801920267251505,-0.00921909513772246,
-1.77354853764314));
#66537=CARTESIAN_POINT('Ctrl Pts',(0.781943449170847,0.120458393815963,
-1.76826783316706));
#66538=CARTESIAN_POINT('Ctrl Pts',(0.761966631090189,0.250135882769648,
-1.76298712869098));
#66539=CARTESIAN_POINT('Ctrl Pts',(0.709036887328268,0.374736973291566,
-1.7577064242149));
#66540=CARTESIAN_POINT('Ctrl Pts',(0.629575365283726,0.479145741679694,
-1.75242571973882));
#66541=CARTESIAN_POINT('Ctrl Pts',(0.550113843239185,0.583554510067822,
-1.74714501526275));
#66542=CARTESIAN_POINT('Ctrl Pts',(0.444120542912024,0.66777095632216,-1.74186431078667));
#66543=CARTESIAN_POINT('Ctrl Pts',(0.324453992537908,0.721578401192921,
-1.73658360631059));
#66544=CARTESIAN_POINT('Ctrl Pts',(0.204787442163794,0.775385846063682,
-1.73130290183451));
#66545=CARTESIAN_POINT('Ctrl Pts',(0.0714476417427256,0.798784289550868,
-1.72602219735843));
#66546=CARTESIAN_POINT('Ctrl Pts',(-0.059389352471172,0.788935160298346,
-1.72074149288235));
#66547=CARTESIAN_POINT('Ctrl Pts',(-0.19022634668507,0.779086031045823,
-1.71546078840628));
#66548=CARTESIAN_POINT('Ctrl Pts',(-0.318560534691797,0.735989329053593,
-1.7101800839302));
#66549=CARTESIAN_POINT('Ctrl Pts',(-0.428823113793521,0.664873310803156,
-1.70489937945412));
#66550=CARTESIAN_POINT('Ctrl Pts',(-0.539085692895245,0.59375729255272,
-1.69961867497804));
#66551=CARTESIAN_POINT('Ctrl Pts',(-0.631276663091966,0.494621958044076,
-1.69433797050196));
#66552=CARTESIAN_POINT('Ctrl Pts',(-0.694211919447908,0.379493864559592,
-1.68905726602588));
#66553=CARTESIAN_POINT('Ctrl Pts',(-0.757147175803852,0.264365771075104,
-1.68377656154981));
#66554=CARTESIAN_POINT('Ctrl Pts',(-0.790826718319016,0.133244918614775,
-1.67849585707373));
#66555=CARTESIAN_POINT('Ctrl Pts',(-0.791164728860946,0.0020381727865403,
-1.67321515259765));
#66556=CARTESIAN_POINT('Ctrl Pts',(-0.791166478467409,0.00135902186643757,
-1.673187818673));
#66557=CARTESIAN_POINT('Ctrl Pts',(-0.79116733475644,0.000679868644999612,
-1.67316048474835));
#66558=CARTESIAN_POINT('Ctrl Pts',(-0.791167298283308,7.15331164842455E-7,
-1.6731331508237));
#66559=CARTESIAN_POINT('Origin',(0.,0.,-1.425));
#66560=CARTESIAN_POINT('',(-0.791042737690139,-1.10214458017843E-5,-1.4446668491763));
#66561=CARTESIAN_POINT('',(-0.791050601996816,-1.425480118063E-5,-1.4731331508237));
#66562=CARTESIAN_POINT('',(-0.7911,-9.68818082805471E-17,-1.425));
#66563=CARTESIAN_POINT('Ctrl Pts',(-0.791042737690139,-1.10214458017843E-5,
-1.4446668491763));
#66564=CARTESIAN_POINT('Ctrl Pts',(-0.791004053579004,0.0782010396373887,
-1.4478132266791));
#66565=CARTESIAN_POINT('Ctrl Pts',(-0.779479835816688,0.156424253179001,
-1.4509596041819));
#66566=CARTESIAN_POINT('Ctrl Pts',(-0.756635697237545,0.231188685144309,
-1.45410598168471));
#66567=CARTESIAN_POINT('Ctrl Pts',(-0.718295369435313,0.356669136927015,
-1.45938668616078));
#66568=CARTESIAN_POINT('Ctrl Pts',(-0.648068643805594,0.472406756836154,
-1.46466739063686));
#66569=CARTESIAN_POINT('Ctrl Pts',(-0.554475043107099,0.56436088901011,
-1.46994809511294));
#66570=CARTESIAN_POINT('Ctrl Pts',(-0.460881442408603,0.656315021184065,
-1.47522879958902));
#66571=CARTESIAN_POINT('Ctrl Pts',(-0.343920966641331,0.724485665622839,
-1.4805095040651));
#66572=CARTESIAN_POINT('Ctrl Pts',(-0.217782621860084,0.76060273210701,
-1.48579020854118));
#66573=CARTESIAN_POINT('Ctrl Pts',(-0.0916442770788372,0.796719798591182,
-1.49107091301725));
#66574=CARTESIAN_POINT('Ctrl Pts',(0.0436719367163846,0.800783287120751,
-1.49635161749333));
#66575=CARTESIAN_POINT('Ctrl Pts',(0.171750195596534,0.77230023746303,-1.50163232196941));
#66576=CARTESIAN_POINT('Ctrl Pts',(0.299828454476682,0.74381718780531,-1.50691302644549));
#66577=CARTESIAN_POINT('Ctrl Pts',(0.420668758441757,0.682787599960299,
-1.51219373092157));
#66578=CARTESIAN_POINT('Ctrl Pts',(0.519611421872524,0.596615250167572,
-1.51747443539765));
#66579=CARTESIAN_POINT('Ctrl Pts',(0.618554085303293,0.510442900374843,
-1.52275513987373));
#66580=CARTESIAN_POINT('Ctrl Pts',(0.69559910819975,0.399127788634402,-1.5280358443498));
#66581=CARTESIAN_POINT('Ctrl Pts',(0.741399809221914,0.276174056273594,
-1.53331654882588));
#66582=CARTESIAN_POINT('Ctrl Pts',(0.787200510244078,0.153220323912786,
-1.53859725330196));
#66583=CARTESIAN_POINT('Ctrl Pts',(0.801756889391944,0.0186279709316112,
-1.54387795777804));
#66584=CARTESIAN_POINT('Ctrl Pts',(0.783303046257617,-0.111274993580937,
-1.54915866225412));
#66585=CARTESIAN_POINT('Ctrl Pts',(0.764849203123291,-0.241177958093484,
-1.5544393667302));
#66586=CARTESIAN_POINT('Ctrl Pts',(0.713385137706772,-0.36639153413741,
-1.55972007120627));
#66587=CARTESIAN_POINT('Ctrl Pts',(0.635154189315716,-0.4717254946127,-1.56500077568235));
#66588=CARTESIAN_POINT('Ctrl Pts',(0.556923240924658,-0.577059455087992,
-1.57028148015843));
#66589=CARTESIAN_POINT('Ctrl Pts',(0.451925409559061,-0.662513799994649,
-1.57556218463451));
#66590=CARTESIAN_POINT('Ctrl Pts',(0.332898458597657,-0.717721674980074,
-1.58084288911059));
#66591=CARTESIAN_POINT('Ctrl Pts',(0.213871507636254,-0.7729295499655,-1.58612359358667));
#66592=CARTESIAN_POINT('Ctrl Pts',(0.0808154370790435,-0.797890955029695,
-1.59140429806274));
#66593=CARTESIAN_POINT('Ctrl Pts',(-0.0501281173771344,-0.789577708855262,
-1.59668500253882));
#66594=CARTESIAN_POINT('Ctrl Pts',(-0.181071671833312,-0.781264462680829,
-1.6019657070149));
#66595=CARTESIAN_POINT('Ctrl Pts',(-0.309902710188458,-0.739676565267769,
-1.60724641149098));
#66596=CARTESIAN_POINT('Ctrl Pts',(-0.420992154574379,-0.669859233167479,
-1.61252711596706));
#66597=CARTESIAN_POINT('Ctrl Pts',(-0.532081598960299,-0.600041901067189,
-1.61780782044314));
#66598=CARTESIAN_POINT('Ctrl Pts',(-0.625429449376996,-0.501995134279669,
-1.62308852491922));
#66599=CARTESIAN_POINT('Ctrl Pts',(-0.689711254499554,-0.387613430997369,
-1.62836922939529));
#66600=CARTESIAN_POINT('Ctrl Pts',(-0.753993059622111,-0.273231727715071,
-1.63364993387137));
#66601=CARTESIAN_POINT('Ctrl Pts',(-0.789208819450532,-0.142515087937991,
-1.63893063834745));
#66602=CARTESIAN_POINT('Ctrl Pts',(-0.79108635035909,-0.0113213403992397,
-1.64421134282353));
#66603=CARTESIAN_POINT('Ctrl Pts',(-0.791140334776021,-0.00754914259760037,
-1.64436317827445));
#66604=CARTESIAN_POINT('Ctrl Pts',(-0.791166757546086,-0.00377655035762189,
-1.64451501372537));
#66605=CARTESIAN_POINT('Ctrl Pts',(-0.791165709393907,-3.94338443360232E-6,
-1.6446668491763));
#66606=CARTESIAN_POINT('Ctrl Pts',(-0.791167298283308,7.15331164842455E-7,
-1.6731331508237));
#66607=CARTESIAN_POINT('Ctrl Pts',(-0.791160288427158,-0.130527339633897,
-1.66787978027227));
#66608=CARTESIAN_POINT('Ctrl Pts',(-0.75817652789474,-0.261058807542124,
-1.66262640972084));
#66609=CARTESIAN_POINT('Ctrl Pts',(-0.696157971514176,-0.375912038965486,
-1.65737303916941));
#66610=CARTESIAN_POINT('Ctrl Pts',(-0.633816725056783,-0.491362865693143,
-1.65209233469333));
#66611=CARTESIAN_POINT('Ctrl Pts',(-0.542137753573301,-0.590971879952318,
-1.64681163021726));
#66612=CARTESIAN_POINT('Ctrl Pts',(-0.432243049112271,-0.662655060220662,
-1.64153092574118));
#66613=CARTESIAN_POINT('Ctrl Pts',(-0.322348344651241,-0.734338240489005,
-1.6362502212651));
#66614=CARTESIAN_POINT('Ctrl Pts',(-0.194237907212663,-0.778095586766515,
-1.63096951678902));
#66615=CARTESIAN_POINT('Ctrl Pts',(-0.063453395297621,-0.788618696815594,
-1.62568881231294));
#66616=CARTESIAN_POINT('Ctrl Pts',(0.0673311166174213,-0.799141806864672,
-1.62040810783686));
#66617=CARTESIAN_POINT('Ctrl Pts',(0.200789703008928,-0.776430680685319,
-1.61512740336078));
#66618=CARTESIAN_POINT('Ctrl Pts',(0.320731897157678,-0.723240508052168,
-1.60984669888471));
#66619=CARTESIAN_POINT('Ctrl Pts',(0.440674091306426,-0.670050335419017,
-1.60456599440863));
#66620=CARTESIAN_POINT('Ctrl Pts',(0.547099893212418,-0.586381116332069,
-1.59928528993255));
#66621=CARTESIAN_POINT('Ctrl Pts',(0.627098305910867,-0.482383143430243,
-1.59400458545647));
#66622=CARTESIAN_POINT('Ctrl Pts',(0.707096718609317,-0.378385170528417,
-1.58872388098039));
#66623=CARTESIAN_POINT('Ctrl Pts',(0.760667742100224,-0.254058443811713,
-1.58344317650431));
#66624=CARTESIAN_POINT('Ctrl Pts',(0.781312432431045,-0.124485602663945,
-1.57816247202824));
#66625=CARTESIAN_POINT('Ctrl Pts',(0.801957122761867,0.0050872384838257,
-1.57288176755216));
#66626=CARTESIAN_POINT('Ctrl Pts',(0.789675479932601,0.139906194062661,
-1.56760106307608));
#66627=CARTESIAN_POINT('Ctrl Pts',(0.745957445766109,0.263615764794187,
-1.5623203586));
#66628=CARTESIAN_POINT('Ctrl Pts',(0.702239411599617,0.387325335525712,
-1.55703965412392));
#66629=CARTESIAN_POINT('Ctrl Pts',(0.627084986095899,0.499925521409928,
-1.55175894964784));
#66630=CARTESIAN_POINT('Ctrl Pts',(0.529611493646138,0.587756282943728,
-1.54647824517177));
#66631=CARTESIAN_POINT('Ctrl Pts',(0.432138001196376,0.67558704447753,-1.54119754069569));
#66632=CARTESIAN_POINT('Ctrl Pts',(0.312345441800571,0.738648381660915,
-1.53591683621961));
#66633=CARTESIAN_POINT('Ctrl Pts',(0.184766394429838,0.769290037522467,
-1.53063613174353));
#66634=CARTESIAN_POINT('Ctrl Pts',(0.057187347059108,0.799931693384018,
-1.52535542726745));
#66635=CARTESIAN_POINT('Ctrl Pts',(-0.078178188286549,0.798153667923737,
-1.52007472279137));
#66636=CARTESIAN_POINT('Ctrl Pts',(-0.204908404256992,0.764171661478476,
-1.51479401831529));
#66637=CARTESIAN_POINT('Ctrl Pts',(-0.331638620227433,0.730189655033216,
-1.50951331383922));
#66638=CARTESIAN_POINT('Ctrl Pts',(-0.449733516822661,0.664003667602976,
-1.50423260936314));
#66639=CARTESIAN_POINT('Ctrl Pts',(-0.544866466249495,0.573643021659559,
-1.49895190488706));
#66640=CARTESIAN_POINT('Ctrl Pts',(-0.639999415676332,0.48328237571614,
-1.49367120041098));
#66641=CARTESIAN_POINT('Ctrl Pts',(-0.712170417934775,0.368747071259543,
-1.4883904959349));
#66642=CARTESIAN_POINT('Ctrl Pts',(-0.752624081245608,0.243931905808006,
-1.48310979145882));
#66643=CARTESIAN_POINT('Ctrl Pts',(-0.77809995370761,0.165329006190866,
-1.47978424458045));
#66644=CARTESIAN_POINT('Ctrl Pts',(-0.790997027553039,0.0826492102907407,
-1.47645869770208));
#66645=CARTESIAN_POINT('Ctrl Pts',(-0.791050601996816,-1.425480118063E-5,
-1.4731331508237));
#66646=CARTESIAN_POINT('Origin',(0.,0.,-1.425));
#66647=CARTESIAN_POINT('',(-0.791104263028763,2.01628765369166E-5,-1.2446668491763));
#66648=CARTESIAN_POINT('',(-0.791090383657342,2.02495652405869E-5,-1.2731331508237));
#66649=CARTESIAN_POINT('',(-0.7911,-9.68818082805471E-17,-1.425));
#66650=CARTESIAN_POINT('Ctrl Pts',(-0.791104263028763,2.01628765369166E-5,
-1.2446668491763));
#66651=CARTESIAN_POINT('Ctrl Pts',(-0.791133904479299,0.0289453631637145,
-1.24583073515675));
#66652=CARTESIAN_POINT('Ctrl Pts',(-0.789578009246314,0.0578673918392402,
-1.2469946211372));
#66653=CARTESIAN_POINT('Ctrl Pts',(-0.786412187639368,0.0866121100375816,
-1.24815850711765));
#66654=CARTESIAN_POINT('Ctrl Pts',(-0.77204843671267,0.217030694506554,
-1.25343921159373));
#66655=CARTESIAN_POINT('Ctrl Pts',(-0.724543437014594,0.343799242098573,
-1.2587199160698));
#66656=CARTESIAN_POINT('Ctrl Pts',(-0.649660235625171,0.451538885059025,
-1.26400062054588));
#66657=CARTESIAN_POINT('Ctrl Pts',(-0.574777034235747,0.559278528019478,
-1.26928132502196));
#66658=CARTESIAN_POINT('Ctrl Pts',(-0.472515631154975,0.647989266348364,
-1.27456202949804));
#66659=CARTESIAN_POINT('Ctrl Pts',(-0.355281821229079,0.706909197830279,
-1.27984273397412));
#66660=CARTESIAN_POINT('Ctrl Pts',(-0.238048011303183,0.765829129312195,
-1.2851234384502));
#66661=CARTESIAN_POINT('Ctrl Pts',(-0.105841794532163,0.794958253947141,
-1.29040414292628));
#66662=CARTESIAN_POINT('Ctrl Pts',(0.0252982930063838,0.790762785444449,
-1.29568484740235));
#66663=CARTESIAN_POINT('Ctrl Pts',(0.15643838054493,0.786567316941757,-1.30096555187843));
#66664=CARTESIAN_POINT('Ctrl Pts',(0.286512338850998,0.74904725530143,-1.30624625635451));
#66665=CARTESIAN_POINT('Ctrl Pts',(0.399740305797077,0.682754329458378,
-1.31152696083059));
#66666=CARTESIAN_POINT('Ctrl Pts',(0.512968272743153,0.616461403615328,
-1.31680766530667));
#66667=CARTESIAN_POINT('Ctrl Pts',(0.609350248329239,0.521395613569551,
-1.32208836978275));
#66668=CARTESIAN_POINT('Ctrl Pts',(0.677193697737961,0.409089821697983,
-1.32736907425882));
#66669=CARTESIAN_POINT('Ctrl Pts',(0.745037147146684,0.296784029826413,
-1.3326497787349));
#66670=CARTESIAN_POINT('Ctrl Pts',(0.784342070378046,0.167238236129048,
-1.33793048321098));
#66671=CARTESIAN_POINT('Ctrl Pts',(0.790340208838238,0.0361682286880373,
-1.34321118768706));
#66672=CARTESIAN_POINT('Ctrl Pts',(0.796338347298431,-0.0949017787529772,
-1.34849189216314));
#66673=CARTESIAN_POINT('Ctrl Pts',(0.769029700987452,-0.227495999937637,
-1.35377259663922));
#66674=CARTESIAN_POINT('Ctrl Pts',(0.711727205709581,-0.345528828212252,
-1.35905330111529));
#66675=CARTESIAN_POINT('Ctrl Pts',(0.65442471043171,-0.463561656486866,
-1.36433400559137));
#66676=CARTESIAN_POINT('Ctrl Pts',(0.567128366186948,-0.567033091851435,
-1.36961471006745));
#66677=CARTESIAN_POINT('Ctrl Pts',(0.460428488626161,-0.643390544952542,
-1.37489541454353));
#66678=CARTESIAN_POINT('Ctrl Pts',(0.353728611065377,-0.719747998053647,
-1.38017611901961));
#66679=CARTESIAN_POINT('Ctrl Pts',(0.227625200188569,-0.768991468891293,
-1.38545682349569));
#66680=CARTESIAN_POINT('Ctrl Pts',(0.0974164329971917,-0.785147008562731,
-1.39073752797176));
#66681=CARTESIAN_POINT('Ctrl Pts',(-0.0327923341941915,-0.801302548234169,
-1.39601823244784));
#66682=CARTESIAN_POINT('Ctrl Pts',(-0.167106457700145,-0.784370156739396,
-1.40129893692392));
#66683=CARTESIAN_POINT('Ctrl Pts',(-0.289231681711864,-0.736403979325904,
-1.4065796414));
#66684=CARTESIAN_POINT('Ctrl Pts',(-0.411356905723584,-0.688437801912412,
-1.41186034587608));
#66685=CARTESIAN_POINT('Ctrl Pts',(-0.52129323024107,-0.609437838580201,
-1.41714105035216));
#66686=CARTESIAN_POINT('Ctrl Pts',(-0.605703780871598,-0.508987933364585,
-1.42242175482824));
#66687=CARTESIAN_POINT('Ctrl Pts',(-0.690114331502122,-0.408538028148975,
-1.42770245930431));
#66688=CARTESIAN_POINT('Ctrl Pts',(-0.748999108245692,-0.286638181049963,
-1.43298316378039));
#66689=CARTESIAN_POINT('Ctrl Pts',(-0.775214531630106,-0.158076615672323,
-1.43826386825647));
#66690=CARTESIAN_POINT('Ctrl Pts',(-0.785810141647417,-0.106115287793623,
-1.44039819522975));
#66691=CARTESIAN_POINT('Ctrl Pts',(-0.791068978833091,-0.0530657205264479,
-1.44253252220302));
#66692=CARTESIAN_POINT('Ctrl Pts',(-0.791042737690139,-1.10214458017843E-5,
-1.4446668491763));
#66693=CARTESIAN_POINT('Ctrl Pts',(-0.791050601996816,-1.425480118063E-5,
-1.4731331508237));
#66694=CARTESIAN_POINT('Ctrl Pts',(-0.791082099517261,-0.0486138108255385,
-1.471177993226));
#66695=CARTESIAN_POINT('Ctrl Pts',(-0.786674232982901,-0.0972077220952497,
-1.46922283562829));
#66696=CARTESIAN_POINT('Ctrl Pts',(-0.777773211183365,-0.144964182843345,
-1.46726767803059));
#66697=CARTESIAN_POINT('Ctrl Pts',(-0.753732353447066,-0.273950079596685,
-1.46198697355451));
#66698=CARTESIAN_POINT('Ctrl Pts',(-0.696914313611244,-0.396826846656892,
-1.45670626907843));
#66699=CARTESIAN_POINT('Ctrl Pts',(-0.61421194591545,-0.498687745825661,
-1.45142556460235));
#66700=CARTESIAN_POINT('Ctrl Pts',(-0.531509578219655,-0.600548644994431,
-1.44614486012628));
#66701=CARTESIAN_POINT('Ctrl Pts',(-0.422922882663888,-0.681393676271764,
-1.4408641556502));
#66702=CARTESIAN_POINT('Ctrl Pts',(-0.301625004027223,-0.731415162057432,
-1.43558345117412));
#66703=CARTESIAN_POINT('Ctrl Pts',(-0.180327125390558,-0.7814366478431,
-1.43030274669804));
#66704=CARTESIAN_POINT('Ctrl Pts',(-0.046318063672995,-0.800634588137102,
-1.42502204222196));
#66705=CARTESIAN_POINT('Ctrl Pts',(0.0841449337465121,-0.786679993686579,
-1.41974133774588));
#66706=CARTESIAN_POINT('Ctrl Pts',(0.214607931166019,-0.772725399236057,
-1.4144606332698));
#66707=CARTESIAN_POINT('Ctrl Pts',(0.34152486428747,-0.72561827004101,-1.40917992879373));
#66708=CARTESIAN_POINT('Ctrl Pts',(0.449498864034337,-0.6510733857053,-1.40389922431765));
#66709=CARTESIAN_POINT('Ctrl Pts',(0.557472863781204,-0.57652850136959,
-1.39861851984157));
#66710=CARTESIAN_POINT('Ctrl Pts',(0.646503930153488,-0.474545861893217,
-1.39333781536549));
#66711=CARTESIAN_POINT('Ctrl Pts',(0.705791300487265,-0.357497444044592,
-1.38805711088941));
#66712=CARTESIAN_POINT('Ctrl Pts',(0.765078670821043,-0.240449026195966,
-1.38277640641333));
#66713=CARTESIAN_POINT('Ctrl Pts',(0.794622345116314,-0.108334829975088,
-1.37749570193726));
#66714=CARTESIAN_POINT('Ctrl Pts',(0.790838246181988,0.0228177719709503,
-1.37221499746118));
#66715=CARTESIAN_POINT('Ctrl Pts',(0.787054147247662,0.153970373916989,
-1.3669342929851));
#66716=CARTESIAN_POINT('Ctrl Pts',(0.749942275083739,0.284161381588188,
-1.36165358850902));
#66717=CARTESIAN_POINT('Ctrl Pts',(0.684004839307479,0.397596733067401,
-1.35637288403294));
#66718=CARTESIAN_POINT('Ctrl Pts',(0.618067403531222,0.511032084546611,
-1.35109217955686));
#66719=CARTESIAN_POINT('Ctrl Pts',(0.523304404142631,0.607711779833835,
-1.34581147508079));
#66720=CARTESIAN_POINT('Ctrl Pts',(0.411211970610016,0.675907166383779,
-1.34053077060471));
#66721=CARTESIAN_POINT('Ctrl Pts',(0.299119537077399,0.744102552933724,
-1.33525006612863));
#66722=CARTESIAN_POINT('Ctrl Pts',(0.169697669400756,0.783813630746388,
-1.32996936165255));
#66723=CARTESIAN_POINT('Ctrl Pts',(0.0386471216343184,0.790222868772667,
-1.32468865717647));
#66724=CARTESIAN_POINT('Ctrl Pts',(-0.0924034261321194,0.796632106798947,
-1.31940795270039));
#66725=CARTESIAN_POINT('Ctrl Pts',(-0.225082653988353,0.769739505038843,
-1.31412724822431));
#66726=CARTESIAN_POINT('Ctrl Pts',(-0.343294642735622,0.712807527044253,
-1.30884654374824));
#66727=CARTESIAN_POINT('Ctrl Pts',(-0.461506631482891,0.655875549049664,
-1.30356583927216));
#66728=CARTESIAN_POINT('Ctrl Pts',(-0.565251381121196,0.56890419482059,
-1.29828513479608));
#66729=CARTESIAN_POINT('Ctrl Pts',(-0.641943145302336,0.462444353994365,
-1.29300443032));
#66730=CARTESIAN_POINT('Ctrl Pts',(-0.718634909483477,0.35598451316814,
-1.28772372584392));
#66731=CARTESIAN_POINT('Ctrl Pts',(-0.768273688207453,0.230036185744764,
-1.28244302136784));
#66732=CARTESIAN_POINT('Ctrl Pts',(-0.784837575978011,0.0998787348482238,
-1.27716231689177));
#66733=CARTESIAN_POINT('Ctrl Pts',(-0.789050312798929,0.0667754505526489,
-1.27581926153574));
#66734=CARTESIAN_POINT('Ctrl Pts',(-0.791123597755304,0.0333998987815609,
-1.27447620617972));
#66735=CARTESIAN_POINT('Ctrl Pts',(-0.791090383657342,2.02495652405869E-5,
-1.2731331508237));
#66736=CARTESIAN_POINT('Origin',(0.,0.,-1.425));
#66737=CARTESIAN_POINT('',(-0.791130810276663,-1.74211169955418E-5,-1.0446668491763));
#66738=CARTESIAN_POINT('',(-0.791143275750807,-1.47194715005396E-5,-1.0731331508237));
#66739=CARTESIAN_POINT('',(-0.7911,-9.68818082805471E-17,-1.425));
#66740=CARTESIAN_POINT('Ctrl Pts',(-0.791130810276663,-1.74211169955418E-5,
-1.0446668491763));
#66741=CARTESIAN_POINT('Ctrl Pts',(-0.791024239474405,0.110865102978929,
-1.04912894811047));
#66742=CARTESIAN_POINT('Ctrl Pts',(-0.767493315443536,0.22179143015014,
-1.05359104704465));
#66743=CARTESIAN_POINT('Ctrl Pts',(-0.722230908301505,0.322998918832374,
-1.05805314597882));
#66744=CARTESIAN_POINT('Ctrl Pts',(-0.668664772830517,0.442773680974816,
-1.0633338504549));
#66745=CARTESIAN_POINT('Ctrl Pts',(-0.584662137800377,0.54893651327924,
-1.06861455493098));
#66746=CARTESIAN_POINT('Ctrl Pts',(-0.480413744051037,0.62860832081652,
-1.07389525940706));
#66747=CARTESIAN_POINT('Ctrl Pts',(-0.376165350301698,0.708280128353801,
-1.07917596388314));
#66748=CARTESIAN_POINT('Ctrl Pts',(-0.25167119783316,0.761460911123938,
-1.08445666835922));
#66749=CARTESIAN_POINT('Ctrl Pts',(-0.12203423720693,0.781699067047047,
-1.08973737283529));
#66750=CARTESIAN_POINT('Ctrl Pts',(0.00760272341930042,0.801937222970155,
-1.09501807731137));
#66751=CARTESIAN_POINT('Ctrl Pts',(0.142382492203222,0.789232752046236,
-1.10029878178745));
#66752=CARTESIAN_POINT('Ctrl Pts',(0.265954323794372,0.745126891293006,
-1.10557948626353));
#66753=CARTESIAN_POINT('Ctrl Pts',(0.389526155385522,0.701021030539776,
-1.11086019073961));
#66754=CARTESIAN_POINT('Ctrl Pts',(0.5018900497839,0.625513779957236,-1.11614089521569));
#66755=CARTESIAN_POINT('Ctrl Pts',(0.589414633078783,0.527765266747921,
-1.12142159969176));
#66756=CARTESIAN_POINT('Ctrl Pts',(0.676939216373666,0.430016753538605,
-1.12670230416784));
#66757=CARTESIAN_POINT('Ctrl Pts',(0.739624488565055,0.310026977702514,
-1.13198300864392));
#66758=CARTESIAN_POINT('Ctrl Pts',(0.769865814832208,0.182352443432055,
-1.13726371312));
#66759=CARTESIAN_POINT('Ctrl Pts',(0.80010714109936,0.0546779091615972,
-1.14254441759608));
#66760=CARTESIAN_POINT('Ctrl Pts',(0.797904521442275,-0.0806813835432276,
-1.14782512207216));
#66761=CARTESIAN_POINT('Ctrl Pts',(0.76352516564653,-0.207304384655365,
-1.15310582654824));
#66762=CARTESIAN_POINT('Ctrl Pts',(0.729145809850785,-0.333927385767502,
-1.15838653102431));
#66763=CARTESIAN_POINT('Ctrl Pts',(0.66258971791638,-0.451814095286952,
-1.16366723550039));
#66764=CARTESIAN_POINT('Ctrl Pts',(0.571931111371964,-0.546663141539403,
-1.16894793997647));
#66765=CARTESIAN_POINT('Ctrl Pts',(0.481272504827549,-0.641512187791854,
-1.17422864445255));
#66766=CARTESIAN_POINT('Ctrl Pts',(0.366511383673123,-0.713323570777307,
-1.17950934892863));
#66767=CARTESIAN_POINT('Ctrl Pts',(0.241569940275243,-0.753385525762419,
-1.18479005340471));
#66768=CARTESIAN_POINT('Ctrl Pts',(0.116628496877367,-0.793447480747529,
-1.19007075788078));
#66769=CARTESIAN_POINT('Ctrl Pts',(-0.0184932687639632,-0.8017600077323,
-1.19535146235686));
#66770=CARTESIAN_POINT('Ctrl Pts',(-0.147403122107609,-0.777314676347893,
-1.20063216683294));
#66771=CARTESIAN_POINT('Ctrl Pts',(-0.276312975451259,-0.752869344963485,
-1.20591287130902));
#66772=CARTESIAN_POINT('Ctrl Pts',(-0.399010916497224,-0.695666155209897,
-1.2111935757851));
#66773=CARTESIAN_POINT('Ctrl Pts',(-0.50061190124246,-0.612644685610925,
-1.21647428026118));
#66774=CARTESIAN_POINT('Ctrl Pts',(-0.602212885987697,-0.529623216011954,
-1.22175498473726));
#66775=CARTESIAN_POINT('Ctrl Pts',(-0.682716914432204,-0.420783466567598,
-1.22703568921333));
#66776=CARTESIAN_POINT('Ctrl Pts',(-0.732357677576797,-0.299329281172457,
-1.23231639368941));
#66777=CARTESIAN_POINT('Ctrl Pts',(-0.771057440605863,-0.204644028651473,
-1.23643321218504));
#66778=CARTESIAN_POINT('Ctrl Pts',(-0.790999417301728,-0.102292092389177,
-1.24055003068067));
#66779=CARTESIAN_POINT('Ctrl Pts',(-0.791104263028763,2.01628765369166E-5,
-1.2446668491763));
#66780=CARTESIAN_POINT('Ctrl Pts',(-0.791090383657342,2.02495652405869E-5,
-1.2731331508237));
#66781=CARTESIAN_POINT('Ctrl Pts',(-0.790993004600682,-0.0978441800543782,
-1.26919550170365));
#66782=CARTESIAN_POINT('Ctrl Pts',(-0.772788585159708,-0.195743830485581,
-1.26525785258359));
#66783=CARTESIAN_POINT('Ctrl Pts',(-0.737307591148638,-0.286920369399794,
-1.26132020346353));
#66784=CARTESIAN_POINT('Ctrl Pts',(-0.689724721731569,-0.409195448381568,
-1.25603949898745));
#66785=CARTESIAN_POINT('Ctrl Pts',(-0.611069986080291,-0.519379031975411,
-1.25075879451137));
#66786=CARTESIAN_POINT('Ctrl Pts',(-0.510885347093584,-0.604104249668043,
-1.24547809003529));
#66787=CARTESIAN_POINT('Ctrl Pts',(-0.410700708106876,-0.688829467360676,
-1.24019738555922));
#66788=CARTESIAN_POINT('Ctrl Pts',(-0.288986165784739,-0.748096319152098,
-1.23491668108314));
#66789=CARTESIAN_POINT('Ctrl Pts',(-0.160507463568594,-0.774714874312284,
-1.22963597660706));
#66790=CARTESIAN_POINT('Ctrl Pts',(-0.0320287613524518,-0.801333429472469,
-1.22435527213098));
#66791=CARTESIAN_POINT('Ctrl Pts',(0.103214100757698,-0.79530368800142,
-1.2190745676549));
#66792=CARTESIAN_POINT('Ctrl Pts',(0.228814197458578,-0.757357145198557,
-1.21379386317882));
#66793=CARTESIAN_POINT('Ctrl Pts',(0.354414294159461,-0.719410602395693,
-1.20851315870275));
#66794=CARTESIAN_POINT('Ctrl Pts',(0.470371625451073,-0.649547258261012,
-1.20323245422667));
#66795=CARTESIAN_POINT('Ctrl Pts',(0.562618881286993,-0.556242552095121,
-1.19795174975059));
#66796=CARTESIAN_POINT('Ctrl Pts',(0.654866137122914,-0.462937845929231,
-1.19267104527451));
#66797=CARTESIAN_POINT('Ctrl Pts',(0.723403317503141,-0.34619177773213,
-1.18739034079843));
#66798=CARTESIAN_POINT('Ctrl Pts',(0.759915866069944,-0.220167342803353,
-1.18210963632235));
#66799=CARTESIAN_POINT('Ctrl Pts',(0.796428414636747,-0.0941429078745748,
-1.17682893184628));
#66800=CARTESIAN_POINT('Ctrl Pts',(0.800916331390125,0.0411598937858802,
-1.1715482273702));
#66801=CARTESIAN_POINT('Ctrl Pts',(0.772835166783604,0.169326865335895,
-1.16626752289412));
#66802=CARTESIAN_POINT('Ctrl Pts',(0.744754002177082,0.29749383688591,-1.16098681841804));
#66803=CARTESIAN_POINT('Ctrl Pts',(0.684103756210661,0.418524978325484,
-1.15570611394196));
#66804=CARTESIAN_POINT('Ctrl Pts',(0.598242185439255,0.517737452675375,
-1.15042540946588));
#66805=CARTESIAN_POINT('Ctrl Pts',(0.512380614667846,0.616949927025268,
-1.1451447049898));
#66806=CARTESIAN_POINT('Ctrl Pts',(0.401307719091452,0.694343734285476,
-1.13986400051373));
#66807=CARTESIAN_POINT('Ctrl Pts',(0.278498255695447,0.740529880502141,
-1.13458329603765));
#66808=CARTESIAN_POINT('Ctrl Pts',(0.155688792299449,0.786716026718803,
-1.12930259156157));
#66809=CARTESIAN_POINT('Ctrl Pts',(0.0211427610838415,0.801694511891926,
-1.12402188708549));
#66810=CARTESIAN_POINT('Ctrl Pts',(-0.108817448365971,0.783648228016271,
-1.11874118260941));
#66811=CARTESIAN_POINT('Ctrl Pts',(-0.238777657815787,0.765601944140615,
-1.11346047813333));
#66812=CARTESIAN_POINT('Ctrl Pts',(-0.364152045499809,0.714530891216179,
-1.10817977365726));
#66813=CARTESIAN_POINT('Ctrl Pts',(-0.469730875528235,0.636630730421804,
-1.10289906918118));
#66814=CARTESIAN_POINT('Ctrl Pts',(-0.575309705556658,0.55873056962743,
-1.0976183647051));
#66815=CARTESIAN_POINT('Ctrl Pts',(-0.661092977929487,0.454001300963119,
-1.09233766022902));
#66816=CARTESIAN_POINT('Ctrl Pts',(-0.716673934610609,0.335148107247632,
-1.08705695575294));
#66817=CARTESIAN_POINT('Ctrl Pts',(-0.765524638913044,0.230686749108265,
-1.0824156874432));
#66818=CARTESIAN_POINT('Ctrl Pts',(-0.791044530563423,0.115314881568087,
-1.07777441913345));
#66819=CARTESIAN_POINT('Ctrl Pts',(-0.791143275750807,-1.47194715005396E-5,
-1.0731331508237));
#66820=CARTESIAN_POINT('Origin',(0.,0.,-1.425));
#66821=CARTESIAN_POINT('',(-0.791033958661136,3.6737787218466E-6,-0.844666849176296));
#66822=CARTESIAN_POINT('',(-0.791032964947078,-4.2330507261862E-7,-0.873133150823704));
#66823=CARTESIAN_POINT('',(-0.7911,-9.68818082805471E-17,-1.425));
#66824=CARTESIAN_POINT('Ctrl Pts',(-0.791033958661136,3.6737787218466E-6,
-0.844666849176296));
#66825=CARTESIAN_POINT('Ctrl Pts',(-0.791043981016399,0.0616432469844158,
-0.847146456588119));
#66826=CARTESIAN_POINT('Ctrl Pts',(-0.783928212048688,0.123280544004755,
-0.849626063999942));
#66827=CARTESIAN_POINT('Ctrl Pts',(-0.769660893106755,0.183215436290213,
-0.852105671411765));
#66828=CARTESIAN_POINT('Ctrl Pts',(-0.739276448117974,0.310855986345038,
-0.857386375887843));
#66829=CARTESIAN_POINT('Ctrl Pts',(-0.676456693085718,0.430775409428172,
-0.862667080363922));
#66830=CARTESIAN_POINT('Ctrl Pts',(-0.588822577554407,0.528425736158908,
-0.867947784840001));
#66831=CARTESIAN_POINT('Ctrl Pts',(-0.501188462023096,0.626076062889645,
-0.873228489316079));
#66832=CARTESIAN_POINT('Ctrl Pts',(-0.38873998599273,0.701457293267984,
-0.878509193792157));
#66833=CARTESIAN_POINT('Ctrl Pts',(-0.265118784355619,0.745424588174215,
-0.883789898268235));
#66834=CARTESIAN_POINT('Ctrl Pts',(-0.141497582718508,0.789391883080447,
-0.889070602744314));
#66835=CARTESIAN_POINT('Ctrl Pts',(-0.00670365547465232,0.80194524251457,
-0.894351307220393));
#66836=CARTESIAN_POINT('Ctrl Pts',(0.122910534398462,0.781561761479401,
-0.899632011696472));
#66837=CARTESIAN_POINT('Ctrl Pts',(0.252524724271576,0.761178280444233,
-0.90491271617255));
#66838=CARTESIAN_POINT('Ctrl Pts',(0.376959176773948,0.707857958939773,
-0.910193420648627));
#66839=CARTESIAN_POINT('Ctrl Pts',(0.481118183817872,0.628069327122963,
-0.915474125124706));
#66840=CARTESIAN_POINT('Ctrl Pts',(0.585277190861797,0.548280695306153,
-0.920754829600784));
#66841=CARTESIAN_POINT('Ctrl Pts',(0.669160752447273,0.442023753176993,
-0.926035534076864));
#66842=CARTESIAN_POINT('Ctrl Pts',(0.722592573074247,0.322189012554494,
-0.931316238552942));
#66843=CARTESIAN_POINT('Ctrl Pts',(0.776024393701218,0.202354271932001,
-0.936596943029021));
#66844=CARTESIAN_POINT('Ctrl Pts',(0.79900447336969,0.0689417328161721,
-0.941877647505098));
#66845=CARTESIAN_POINT('Ctrl Pts',(0.788744994336818,-0.0618637242777383,
-0.947158351981176));
#66846=CARTESIAN_POINT('Ctrl Pts',(0.778485515303946,-0.19266918137166,
-0.952439056457254));
#66847=CARTESIAN_POINT('Ctrl Pts',(0.734986477569723,-0.320867556443662,
-0.957719760933334));
#66848=CARTESIAN_POINT('Ctrl Pts',(0.663524946790219,-0.430906522879311,
-0.963000465409413));
#66849=CARTESIAN_POINT('Ctrl Pts',(0.592063416010716,-0.540945489314955,
-0.968281169885491));
#66850=CARTESIAN_POINT('Ctrl Pts',(0.492639392185934,-0.632825047114247,
-0.973561874361569));
#66851=CARTESIAN_POINT('Ctrl Pts',(0.377314454809184,-0.695398870192459,
-0.978842578837647));
#66852=CARTESIAN_POINT('Ctrl Pts',(0.261989517432433,-0.757972693270672,
-0.984123283313726));
#66853=CARTESIAN_POINT('Ctrl Pts',(0.130763666503716,-0.791240781627805,
-0.989403987789805));
#66854=CARTESIAN_POINT('Ctrl Pts',(-0.000443494528374638,-0.791167232502398,
-0.994684692265883));
#66855=CARTESIAN_POINT('Ctrl Pts',(-0.131650655560465,-0.791093683376991,
-0.999965396741962));
#66856=CARTESIAN_POINT('Ctrl Pts',(-0.262839126695928,-0.757678496769043,
-1.00524610121804));
#66857=CARTESIAN_POINT('Ctrl Pts',(-0.378093839198509,-0.694975420596321,
-1.01052680569412));
#66858=CARTESIAN_POINT('Ctrl Pts',(-0.493348551701089,-0.632272344423598,
-1.0158075101702));
#66859=CARTESIAN_POINT('Ctrl Pts',(-0.592669505570787,-0.540281378686101,
-1.02108821464627));
#66860=CARTESIAN_POINT('Ctrl Pts',(-0.66400762519825,-0.430162364871081,
-1.02636891912235));
#66861=CARTESIAN_POINT('Ctrl Pts',(-0.735345744825713,-0.320043351056061,
-1.03164962359843));
#66862=CARTESIAN_POINT('Ctrl Pts',(-0.778701030210941,-0.191796289163518,
-1.03693032807451));
#66863=CARTESIAN_POINT('Ctrl Pts',(-0.788813854947635,-0.0609794122270167,
-1.04221103255059));
#66864=CARTESIAN_POINT('Ctrl Pts',(-0.790381527293484,-0.0407004095068838,
-1.04302963809249));
#66865=CARTESIAN_POINT('Ctrl Pts',(-0.791150361490256,-0.020359652444469,
-1.04384824363439));
#66866=CARTESIAN_POINT('Ctrl Pts',(-0.791130810276663,-1.74211169955418E-5,
-1.0446668491763));
#66867=CARTESIAN_POINT('Ctrl Pts',(-0.791143275750807,-1.47194715005396E-5,
-1.0731331508237));
#66868=CARTESIAN_POINT('Ctrl Pts',(-0.791156880058908,-0.0159038930835007,
-1.07249371465737));
#66869=CARTESIAN_POINT('Ctrl Pts',(-0.790687963417032,-0.031792264431447,
-1.07185427849104));
#66870=CARTESIAN_POINT('Ctrl Pts',(-0.78973105947805,-0.0476511913555044,
-1.07121484232471));
#66871=CARTESIAN_POINT('Ctrl Pts',(-0.781828586674952,-0.178620177476483,
-1.06593413784863));
#66872=CARTESIAN_POINT('Ctrl Pts',(-0.74064500007934,-0.307581030951775,
-1.06065343337255));
#66873=CARTESIAN_POINT('Ctrl Pts',(-0.67117646746268,-0.41888892545189,
-1.05537272889647));
#66874=CARTESIAN_POINT('Ctrl Pts',(-0.60170793484602,-0.530196819952006,
-1.05009202442039));
#66875=CARTESIAN_POINT('Ctrl Pts',(-0.503954456208311,-0.623851755476946,
-1.04481131994431));
#66876=CARTESIAN_POINT('Ctrl Pts',(-0.389774949625676,-0.688492026813836,
-1.03953061546824));
#66877=CARTESIAN_POINT('Ctrl Pts',(-0.27559544304304,-0.753132298150725,
-1.03424991099216));
#66878=CARTESIAN_POINT('Ctrl Pts',(-0.144989908515477,-0.788757905299564,
-1.02896920651608));
#66879=CARTESIAN_POINT('Ctrl Pts',(-0.0138026960941072,-0.791046944196395,
-1.02368850204));
#66880=CARTESIAN_POINT('Ctrl Pts',(0.117384516327263,-0.793335983093227,
-1.01840779756392));
#66881=CARTESIAN_POINT('Ctrl Pts',(0.24915340664244,-0.762288453738051,
-1.01312709308784));
#66882=CARTESIAN_POINT('Ctrl Pts',(0.365518492830672,-0.701670872803422,
-1.00784638861177));
#66883=CARTESIAN_POINT('Ctrl Pts',(0.481883579018903,-0.641053291868793,
-1.00256568413569));
#66884=CARTESIAN_POINT('Ctrl Pts',(0.582844861080188,-0.550865659354709,
-0.997284979659609));
#66885=CARTESIAN_POINT('Ctrl Pts',(0.656154267748824,-0.442049046211985,
-0.99200427518353));
#66886=CARTESIAN_POINT('Ctrl Pts',(0.729463674417461,-0.33323243306926,
-0.986723570707451));
#66887=CARTESIAN_POINT('Ctrl Pts',(0.775121205693448,-0.205786839297894,
-0.981442866231373));
#66888=CARTESIAN_POINT('Ctrl Pts',(0.787587939274424,-0.0751732681967957,
-0.976162161755294));
#66889=CARTESIAN_POINT('Ctrl Pts',(0.8000546728554,0.0554403029043047,-0.970881457279216));
#66890=CARTESIAN_POINT('Ctrl Pts',(0.779330608741366,0.189221851335134,
-0.965600752803138));
#66891=CARTESIAN_POINT('Ctrl Pts',(0.727929877190982,0.309941730385962,
-0.960320048327059));
#66892=CARTESIAN_POINT('Ctrl Pts',(0.6765291456406,0.430661609436785,-0.955039343850981));
#66893=CARTESIAN_POINT('Ctrl Pts',(0.594451746653871,0.538319819107605,
-0.949758639374903));
#66894=CARTESIAN_POINT('Ctrl Pts',(0.491654861950048,0.619855853455302,
-0.944477934898824));
#66895=CARTESIAN_POINT('Ctrl Pts',(0.388857977246223,0.701391887803002,
-0.939197230422746));
#66896=CARTESIAN_POINT('Ctrl Pts',(0.265341606825302,0.756805746827579,
-0.933916525946668));
#66897=CARTESIAN_POINT('Ctrl Pts',(0.136090082071649,0.77937492383554,-0.928635821470589));
#66898=CARTESIAN_POINT('Ctrl Pts',(0.00683855731799995,0.8019441008435,
-0.923355116994511));
#66899=CARTESIAN_POINT('Ctrl Pts',(-0.128148121768382,0.791668595834846,
-0.918074412518432));
#66900=CARTESIAN_POINT('Ctrl Pts',(-0.25249410860933,0.749794976950034,
-0.912793708042354));
#66901=CARTESIAN_POINT('Ctrl Pts',(-0.376840095450286,0.707921358065218,
-0.907513003566275));
#66902=CARTESIAN_POINT('Ctrl Pts',(-0.490545390045807,0.63444962530424,
-0.902232299090197));
#66903=CARTESIAN_POINT('Ctrl Pts',(-0.579815887140293,0.538292967965992,
-0.896951594614119));
#66904=CARTESIAN_POINT('Ctrl Pts',(-0.669086384234776,0.442136310627747,
-0.89167089013804));
#66905=CARTESIAN_POINT('Ctrl Pts',(-0.733922083828226,0.323294728712234,
-0.886390185661961));
#66906=CARTESIAN_POINT('Ctrl Pts',(-0.766457472993615,0.196185433797119,
-0.881109481185883));
#66907=CARTESIAN_POINT('Ctrl Pts',(-0.78283868460536,0.132187297883035,
-0.87845070439849));
#66908=CARTESIAN_POINT('Ctrl Pts',(-0.791031728575481,0.0660932867542428,
-0.875791927611097));
#66909=CARTESIAN_POINT('Ctrl Pts',(-0.791032964947078,-4.2330507261862E-7,
-0.873133150823704));
#66910=CARTESIAN_POINT('Origin',(0.,0.,-1.425));
#66911=CARTESIAN_POINT('',(-0.791151924025282,1.20225912425137E-5,-0.644666849176296));
#66912=CARTESIAN_POINT('',(-0.791140835429741,1.53413302099771E-5,-0.673133150823704));
#66913=CARTESIAN_POINT('',(-0.7911,-9.68818082805471E-17,-1.425));
#66914=CARTESIAN_POINT('Ctrl Pts',(-0.791151924025282,1.20225912425137E-5,
-0.644666849176296));
#66915=CARTESIAN_POINT('Ctrl Pts',(-0.791160987250509,0.0123643276965679,
-0.645163965065766));
#66916=CARTESIAN_POINT('Ctrl Pts',(-0.790877649980244,0.0247162168630147,
-0.645661080955236));
#66917=CARTESIAN_POINT('Ctrl Pts',(-0.790299163437089,0.0370542675482504,
-0.646158196844706));
#66918=CARTESIAN_POINT('Ctrl Pts',(-0.784154084306661,0.168117468020605,
-0.651438901320784));
#66919=CARTESIAN_POINT('Ctrl Pts',(-0.744703950154256,0.297619114999562,
-0.656719605796863));
#66920=CARTESIAN_POINT('Ctrl Pts',(-0.676734635769451,0.409848776041709,
-0.662000310272941));
#66921=CARTESIAN_POINT('Ctrl Pts',(-0.608765321384648,0.522078437083854,
-0.66728101474902));
#66922=CARTESIAN_POINT('Ctrl Pts',(-0.512276826767448,0.617036112189189,
-0.672561719225099));
#66923=CARTESIAN_POINT('Ctrl Pts',(-0.398974609042237,0.683202054894812,
-0.677842423701178));
#66924=CARTESIAN_POINT('Ctrl Pts',(-0.28567239131703,0.749367997600434,
-0.683123128177256));
#66925=CARTESIAN_POINT('Ctrl Pts',(-0.155556450483816,0.786742207906344,
-0.688403832653334));
#66926=CARTESIAN_POINT('Ctrl Pts',(-0.0244117417609882,0.79079065076485,
-0.693684537129412));
#66927=CARTESIAN_POINT('Ctrl Pts',(0.106732966961839,0.794839093623355,
-0.69896524160549));
#66928=CARTESIAN_POINT('Ctrl Pts',(0.238906443574278,0.765561769034455,
-0.704245946081569));
#66929=CARTESIAN_POINT('Ctrl Pts',(0.356074123855939,0.706510442097727,
-0.709526650557647));
#66930=CARTESIAN_POINT('Ctrl Pts',(0.473241804137603,0.647459115160997,
-0.714807355033725));
#66931=CARTESIAN_POINT('Ctrl Pts',(0.575403688088487,0.558633785876438,
-0.720088059509804));
#66932=CARTESIAN_POINT('Ctrl Pts',(0.650166053979608,0.450810258008273,
-0.725368763985882));
#66933=CARTESIAN_POINT('Ctrl Pts',(0.724928419870729,0.342986730140108,
-0.730649468461961));
#66934=CARTESIAN_POINT('Ctrl Pts',(0.772291267702086,0.216165003688338,
-0.735930172938039));
#66935=CARTESIAN_POINT('Ctrl Pts',(0.786508795481657,0.0857303977763639,
-0.741210877414117));
#66936=CARTESIAN_POINT('Ctrl Pts',(0.800726323261227,-0.0447042081356141,
-0.746491581890196));
#66937=CARTESIAN_POINT('Ctrl Pts',(0.781798530989006,-0.178751693507805,
-0.751772286366276));
#66938=CARTESIAN_POINT('Ctrl Pts',(0.732021635035464,-0.300150149613334,
-0.757052990842354));
#66939=CARTESIAN_POINT('Ctrl Pts',(0.682244739081924,-0.421548605718856,
-0.762333695318433));
#66940=CARTESIAN_POINT('Ctrl Pts',(0.601618739447067,-0.530298032557726,
-0.76761439979451));
#66941=CARTESIAN_POINT('Ctrl Pts',(0.499924742008656,-0.613205543680484,
-0.772895104270588));
#66942=CARTESIAN_POINT('Ctrl Pts',(0.398230744570239,-0.696113054803247,
-0.778175808746667));
#66943=CARTESIAN_POINT('Ctrl Pts',(0.275468749328266,-0.753178650209894,
-0.783456513222746));
#66944=CARTESIAN_POINT('Ctrl Pts',(0.146531570990962,-0.777479443571225,
-0.788737217698825));
#66945=CARTESIAN_POINT('Ctrl Pts',(0.0175943926536692,-0.801780236932554,
-0.794017922174903));
#66946=CARTESIAN_POINT('Ctrl Pts',(-0.117517968778952,-0.793316228248573,
-0.799298626650981));
#66947=CARTESIAN_POINT('Ctrl Pts',(-0.242414419632999,-0.753114224820442,
-0.804579331127059));
#66948=CARTESIAN_POINT('Ctrl Pts',(-0.367310870487054,-0.712912221392309,
-0.809860035603137));
#66949=CARTESIAN_POINT('Ctrl Pts',(-0.481991410762531,-0.640972223220024,
-0.815140740079216));
#66950=CARTESIAN_POINT('Ctrl Pts',(-0.57254362372496,-0.546021597928866,
-0.820421444555294));
#66951=CARTESIAN_POINT('Ctrl Pts',(-0.663095836687388,-0.451070972637709,
-0.825702149031373));
#66952=CARTESIAN_POINT('Ctrl Pts',(-0.729519722336766,-0.33310972022768,
-0.830982853507451));
#66953=CARTESIAN_POINT('Ctrl Pts',(-0.763757097688803,-0.206448255509406,
-0.83626355798353));
#66954=CARTESIAN_POINT('Ctrl Pts',(-0.781917972250301,-0.139261943799696,
-0.839064655047785));
#66955=CARTESIAN_POINT('Ctrl Pts',(-0.791022636872949,-0.0696276826711715,
-0.841865752112041));
#66956=CARTESIAN_POINT('Ctrl Pts',(-0.791033958661136,3.6737787218466E-6,
-0.844666849176296));
#66957=CARTESIAN_POINT('Ctrl Pts',(-0.791032964947078,-4.2330507261862E-7,
-0.873133150823704));
#66958=CARTESIAN_POINT('Ctrl Pts',(-0.791034184183284,-0.0651781130134306,
-0.870511223135018));
#66959=CARTESIAN_POINT('Ctrl Pts',(-0.783069089680566,-0.130355509939776,
-0.867889295446333));
#66960=CARTESIAN_POINT('Ctrl Pts',(-0.76713419073724,-0.193522390807475,
-0.865267367757648));
#66961=CARTESIAN_POINT('Ctrl Pts',(-0.735040440578149,-0.320743912582239,
-0.859986663281569));
#66962=CARTESIAN_POINT('Ctrl Pts',(-0.670617861522639,-0.43980994821705,
-0.854705958805491));
#66963=CARTESIAN_POINT('Ctrl Pts',(-0.581681848970635,-0.536276056635037,
-0.849425254329413));
#66964=CARTESIAN_POINT('Ctrl Pts',(-0.492745836418631,-0.632742165053023,
-0.844144549853334));
#66965=CARTESIAN_POINT('Ctrl Pts',(-0.379296390370133,-0.706608346254182,
-0.838863845377255));
#66966=CARTESIAN_POINT('Ctrl Pts',(-0.255096577932519,-0.74891355860943,
-0.833583140901176));
#66967=CARTESIAN_POINT('Ctrl Pts',(-0.130896765494906,-0.791218770964677,
-0.828302436425098));
#66968=CARTESIAN_POINT('Ctrl Pts',(0.00405341333182155,-0.801963014474012,
-0.82302173194902));
#66969=CARTESIAN_POINT('Ctrl Pts',(0.133382539981627,-0.779842856202435,
-0.817741027472942));
#66970=CARTESIAN_POINT('Ctrl Pts',(0.262711666631428,-0.757722697930859,
-0.812460322996864));
#66971=CARTESIAN_POINT('Ctrl Pts',(0.386419741104306,-0.702738137878373,
-0.807179618520785));
#66972=CARTESIAN_POINT('Ctrl Pts',(0.489499175527448,-0.621559602532107,
-0.801898914044706));
#66973=CARTESIAN_POINT('Ctrl Pts',(0.592578609950594,-0.540381067185838,
-0.796618209568628));
#66974=CARTESIAN_POINT('Ctrl Pts',(0.675029404324002,-0.433008556545788,
-0.79133750509255));
#66975=CARTESIAN_POINT('Ctrl Pts',(0.72684907863968,-0.312467917109214,
-0.786056800616472));
#66976=CARTESIAN_POINT('Ctrl Pts',(0.778668752955358,-0.191927277672641,
-0.780776096140393));
#66977=CARTESIAN_POINT('Ctrl Pts',(0.799857307213305,-0.0582185094395453,
-0.775495391664314));
#66978=CARTESIAN_POINT('Ctrl Pts',(0.787844261747754,0.0724375701763816,
-0.770214687188236));
#66979=CARTESIAN_POINT('Ctrl Pts',(0.775831216282202,0.203093649792305,
-0.764933982712157));
#66980=CARTESIAN_POINT('Ctrl Pts',(0.73061657109315,0.330697040791069,-0.759653278236079));
#66981=CARTESIAN_POINT('Ctrl Pts',(0.657685519962043,0.439767596776046,
-0.754372573760001));
#66982=CARTESIAN_POINT('Ctrl Pts',(0.584754468830932,0.548838152761029,
-0.749091869283922));
#66983=CARTESIAN_POINT('Ctrl Pts',(0.484107011757771,0.639375873732224,
-0.743811164807844));
#66984=CARTESIAN_POINT('Ctrl Pts',(0.367953148474873,0.700397217919481,
-0.738530460331766));
#66985=CARTESIAN_POINT('Ctrl Pts',(0.251799285191982,0.761418562106735,
-0.733249755855687));
#66986=CARTESIAN_POINT('Ctrl Pts',(0.120139015699353,0.792923529510048,
-0.727969051379608));
#66987=CARTESIAN_POINT('Ctrl Pts',(-0.0110553552671211,0.791090109571494,
-0.722688346903529));
#66988=CARTESIAN_POINT('Ctrl Pts',(-0.142249726233599,0.789256689632941,
-0.717407642427451));
#66989=CARTESIAN_POINT('Ctrl Pts',(-0.272978198673932,0.754084882352523,
-0.712126937951373));
#66990=CARTESIAN_POINT('Ctrl Pts',(-0.387381508380938,0.689841539272919,
-0.706846233475295));
#66991=CARTESIAN_POINT('Ctrl Pts',(-0.501784818087942,0.625598196193318,
-0.701565528999217));
#66992=CARTESIAN_POINT('Ctrl Pts',(-0.599862965061619,0.532283317314533,
-0.696284824523138));
#66993=CARTESIAN_POINT('Ctrl Pts',(-0.669717644236744,0.421217354034596,
-0.69100412004706));
#66994=CARTESIAN_POINT('Ctrl Pts',(-0.739572323411872,0.310151390754656,
-0.685723415570981));
#66995=CARTESIAN_POINT('Ctrl Pts',(-0.781203534788445,0.181334343073565,
-0.680442711094903));
#66996=CARTESIAN_POINT('Ctrl Pts',(-0.789560807201604,0.0503935915873558,
-0.675162006618824));
#66997=CARTESIAN_POINT('Ctrl Pts',(-0.790631100041234,0.0336243705062366,
-0.674485721353784));
#66998=CARTESIAN_POINT('Ctrl Pts',(-0.791155659727199,0.0168203180943188,
-0.673809436088744));
#66999=CARTESIAN_POINT('Ctrl Pts',(-0.791140835429741,1.53413302099771E-5,
-0.673133150823704));
#67000=CARTESIAN_POINT('Origin',(0.,0.,-1.425));
#67001=CARTESIAN_POINT('',(-0.791079804116067,-1.96820758422422E-5,-0.444666849176296));
#67002=CARTESIAN_POINT('',(-0.791093201014614,-2.03057722054419E-5,-0.473133150823703));
#67003=CARTESIAN_POINT('',(-0.7911,-9.68818082805471E-17,-1.425));
#67004=CARTESIAN_POINT('Ctrl Pts',(-0.791079804116067,-1.96820758422422E-5,
-0.444666849176296));
#67005=CARTESIAN_POINT('Ctrl Pts',(-0.790990645563059,0.0943112144519883,
-0.448462178019491));
#67006=CARTESIAN_POINT('Ctrl Pts',(-0.774106485915666,0.188673174257029,
-0.452257506862687));
#67007=CARTESIAN_POINT('Ctrl Pts',(-0.7410897206494,0.277005076527925,-0.456052835705883));
#67008=CARTESIAN_POINT('Ctrl Pts',(-0.695151203242722,0.399907383804603,
-0.461333540181961));
#67009=CARTESIAN_POINT('Ctrl Pts',(-0.617981431816262,0.511136049324216,
-0.46661424465804));
#67010=CARTESIAN_POINT('Ctrl Pts',(-0.518942221524803,0.597197418942259,
-0.471894949134119));
#67011=CARTESIAN_POINT('Ctrl Pts',(-0.41990301123335,0.683258788560297,
-0.477175653610197));
#67012=CARTESIAN_POINT('Ctrl Pts',(-0.298994362076898,0.744152862276769,
-0.482456358086275));
#67013=CARTESIAN_POINT('Ctrl Pts',(-0.170884250937674,0.772492303686205,
-0.487737062562353));
#67014=CARTESIAN_POINT('Ctrl Pts',(-0.0427741397984416,0.800831745095644,
-0.493017767038432));
#67015=CARTESIAN_POINT('Ctrl Pts',(0.0925374333235549,0.796616554198045,
-0.49829847151451));
#67016=CARTESIAN_POINT('Ctrl Pts',(0.218635207479237,0.760358094928631,
-0.503579175990589));
#67017=CARTESIAN_POINT('Ctrl Pts',(0.344732981634912,0.724099635659218,
-0.508859880466667));
#67018=CARTESIAN_POINT('Ctrl Pts',(0.461616956824271,0.655797908017987,
-0.514140584942746));
#67019=CARTESIAN_POINT('Ctrl Pts',(0.555107407625345,0.563738904522544,
-0.519421289418824));
#67020=CARTESIAN_POINT('Ctrl Pts',(0.648597858426425,0.471679901027096,
-0.524701993894903));
#67021=CARTESIAN_POINT('Ctrl Pts',(0.718694784839222,0.355863621677439,
-0.529982698370981));
#67022=CARTESIAN_POINT('Ctrl Pts',(0.756894410636733,0.230340264868805,
-0.53526340284706));
#67023=CARTESIAN_POINT('Ctrl Pts',(0.795094036434242,0.104816908060178,
-0.540544107323138));
#67024=CARTESIAN_POINT('Ctrl Pts',(0.801396361616462,-0.0304135262074155,
-0.545824811799215));
#67025=CARTESIAN_POINT('Ctrl Pts',(0.775036822517206,-0.158945620308655,
-0.551105516275294));
#67026=CARTESIAN_POINT('Ctrl Pts',(0.74867728341795,-0.287477714409898,
-0.556386220751372));
#67027=CARTESIAN_POINT('Ctrl Pts',(0.689655880037216,-0.40931146834479,
-0.561666925227452));
#67028=CARTESIAN_POINT('Ctrl Pts',(0.605132766644463,-0.509666676570216,
-0.56694762970353));
#67029=CARTESIAN_POINT('Ctrl Pts',(0.520609653251709,-0.610021884795641,
-0.572228334179609));
#67030=CARTESIAN_POINT('Ctrl Pts',(0.410584829846934,-0.688898547311603,
-0.577509038655687));
#67031=CARTESIAN_POINT('Ctrl Pts',(0.288405907024508,-0.736727778264311,
-0.582789743131765));
#67032=CARTESIAN_POINT('Ctrl Pts',(0.166226984202082,-0.784557009217019,
-0.588070447607843));
#67033=CARTESIAN_POINT('Ctrl Pts',(0.0318939619620019,-0.801338808606473,
-0.593351152083922));
#67034=CARTESIAN_POINT('Ctrl Pts',(-0.0982966111957519,-0.785037300196832,
-0.59863185656));
#67035=CARTESIAN_POINT('Ctrl Pts',(-0.228487184353502,-0.768735791787191,
-0.603912561036079));
#67036=CARTESIAN_POINT('Ctrl Pts',(-0.354535308428928,-0.719350975578457,
-0.609193265512157));
#67037=CARTESIAN_POINT('Ctrl Pts',(-0.461149513513319,-0.642873947721737,
-0.614473969988235));
#67038=CARTESIAN_POINT('Ctrl Pts',(-0.567763718597715,-0.566396919865013,
-0.619754674464314));
#67039=CARTESIAN_POINT('Ctrl Pts',(-0.654944004691074,-0.462827680360298,
-0.625035378940393));
#67040=CARTESIAN_POINT('Ctrl Pts',(-0.712114135683525,-0.344730683625065,
-0.630316083416471));
#67041=CARTESIAN_POINT('Ctrl Pts',(-0.76390237479996,-0.237751122800469,
-0.635099672003079));
#67042=CARTESIAN_POINT('Ctrl Pts',(-0.791064711482551,-0.118850292960821,
-0.639883260589688));
#67043=CARTESIAN_POINT('Ctrl Pts',(-0.791151924025282,1.20225912425137E-5,
-0.644666849176296));
#67044=CARTESIAN_POINT('Ctrl Pts',(-0.791140835429741,1.53413302099771E-5,
-0.673133150823704));
#67045=CARTESIAN_POINT('Ctrl Pts',(-0.791039905713343,-0.11439962799359,
-0.668528731612665));
#67046=CARTESIAN_POINT('Ctrl Pts',(-0.765936218386557,-0.228857445000086,
-0.663924312401627));
#67047=CARTESIAN_POINT('Ctrl Pts',(-0.717833561436095,-0.332657121399638,
-0.659319893190589));
#67048=CARTESIAN_POINT('Ctrl Pts',(-0.662665709807682,-0.451702627609097,
-0.654039188714511));
#67049=CARTESIAN_POINT('Ctrl Pts',(-0.577246673101113,-0.556729184736689,
-0.648758484238432));
#67050=CARTESIAN_POINT('Ctrl Pts',(-0.47193902227101,-0.634995544551145,
-0.643477779762354));
#67051=CARTESIAN_POINT('Ctrl Pts',(-0.366631371440906,-0.7132619043656,
-0.638197075286275));
#67052=CARTESIAN_POINT('Ctrl Pts',(-0.241435106487268,-0.764768066866919,
-0.632916370810197));
#67053=CARTESIAN_POINT('Ctrl Pts',(-0.111538354423194,-0.783265585759063,
-0.627635666334118));
#67054=CARTESIAN_POINT('Ctrl Pts',(0.0183583976408846,-0.801763104651207,
-0.62235496185804));
#67055=CARTESIAN_POINT('Ctrl Pts',(0.1529556368154,-0.787251979934175,-0.617074257381961));
#67056=CARTESIAN_POINT('Ctrl Pts',(0.275924761245081,-0.741492621995504,
-0.611793552905882));
#67057=CARTESIAN_POINT('Ctrl Pts',(0.398893885674758,-0.695733264056833,
-0.606512848429804));
#67058=CARTESIAN_POINT('Ctrl Pts',(0.510234895359602,-0.618725672896525,
-0.601232143953725));
#67059=CARTESIAN_POINT('Ctrl Pts',(0.596440507175103,-0.519811988840799,
-0.595951439477647));
#67060=CARTESIAN_POINT('Ctrl Pts',(0.682646118990602,-0.420898304785076,
-0.590670735001569));
#67061=CARTESIAN_POINT('Ctrl Pts',(0.743716332936759,-0.300078527833936,
-0.585390030525491));
#67062=CARTESIAN_POINT('Ctrl Pts',(0.772242444237319,-0.172009853381406,
-0.580109326049412));
#67063=CARTESIAN_POINT('Ctrl Pts',(0.80076855553788,-0.0439411789288734,
-0.574828621573334));
#67064=CARTESIAN_POINT('Ctrl Pts',(0.796750564192842,0.0913763930250492,
-0.569547917097255));
#67065=CARTESIAN_POINT('Ctrl Pts',(0.760675910964986,0.217526873786918,
-0.564267212621177));
#67066=CARTESIAN_POINT('Ctrl Pts',(0.72460125773713,0.343677354548784,-0.558986508145099));
#67067=CARTESIAN_POINT('Ctrl Pts',(0.656469942626458,0.460660744118596,
-0.55370580366902));
#67068=CARTESIAN_POINT('Ctrl Pts',(0.564547284633123,0.554285256664192,
-0.548425099192942));
#67069=CARTESIAN_POINT('Ctrl Pts',(0.472624626639786,0.647909769209791,
-0.543144394716863));
#67070=CARTESIAN_POINT('Ctrl Pts',(0.356910625763784,0.718175404731173,
-0.537863690240785));
#67071=CARTESIAN_POINT('Ctrl Pts',(0.231443072534656,0.756557920134102,
-0.532582985764707));
#67072=CARTESIAN_POINT('Ctrl Pts',(0.105975519305528,0.794940435537032,
-0.527302281288628));
#67073=CARTESIAN_POINT('Ctrl Pts',(-0.0292455862767264,0.80143983082151,
-0.52202157681255));
#67074=CARTESIAN_POINT('Ctrl Pts',(-0.157815958291974,0.775267634852832,
-0.516740872336471));
#67075=CARTESIAN_POINT('Ctrl Pts',(-0.286386330307222,0.749095438884155,
-0.511460167860393));
#67076=CARTESIAN_POINT('Ctrl Pts',(-0.408305968755463,0.690251651662321,
-0.506179463384315));
#67077=CARTESIAN_POINT('Ctrl Pts',(-0.508784249053499,0.605874880034648,
-0.500898758908236));
#67078=CARTESIAN_POINT('Ctrl Pts',(-0.609262529351534,0.521498108406975,
-0.495618054432158));
#67079=CARTESIAN_POINT('Ctrl Pts',(-0.688299451499364,0.411588352373463,
-0.490337349956079));
#67080=CARTESIAN_POINT('Ctrl Pts',(-0.736306687820121,0.289479263183488,
-0.48505664548));
#67081=CARTESIAN_POINT('Ctrl Pts',(-0.772439116004476,0.197574412291118,
-0.481082147261235));
#67082=CARTESIAN_POINT('Ctrl Pts',(-0.790993997334175,0.0987589419568265,
-0.477107649042469));
#67083=CARTESIAN_POINT('Ctrl Pts',(-0.791093201014614,-2.03057722054419E-5,
-0.473133150823703));
#67084=CARTESIAN_POINT('Origin',(0.,0.,-1.425));
#67085=CARTESIAN_POINT('',(-0.791058280240756,1.64158700123596E-5,-0.244666849176296));
#67086=CARTESIAN_POINT('',(-0.791048813772023,1.36328575649638E-5,-0.273133150823704));
#67087=CARTESIAN_POINT('',(-0.7911,-9.68818082805471E-17,-1.425));
#67088=CARTESIAN_POINT('Ctrl Pts',(-0.791058280240756,1.64158700123596E-5,
-0.244666849176296));
#67089=CARTESIAN_POINT('Ctrl Pts',(-0.791092359377555,0.0450770503401576,
-0.246479686497138));
#67090=CARTESIAN_POINT('Ctrl Pts',(-0.787306067959793,0.0901320191018208,
-0.248292523817981));
#67091=CARTESIAN_POINT('Ctrl Pts',(-0.779647639886365,0.134518896239813,
-0.250105361138824));
#67092=CARTESIAN_POINT('Ctrl Pts',(-0.757339021820034,0.26381565005596,
-0.255386065614902));
#67093=CARTESIAN_POINT('Ctrl Pts',(-0.702174248899364,0.387443460909541,
-0.260666770090981));
#67094=CARTESIAN_POINT('Ctrl Pts',(-0.620845581003012,0.490404481077766,
-0.265947474567059));
#67095=CARTESIAN_POINT('Ctrl Pts',(-0.539516913106655,0.593365501245996,
-0.271228179043138));
#67096=CARTESIAN_POINT('Ctrl Pts',(-0.432024350234614,0.675659730728867,
-0.276508883519216));
#67097=CARTESIAN_POINT('Ctrl Pts',(-0.311408317767632,0.727303681583887,
-0.281789587995295));
#67098=CARTESIAN_POINT('Ctrl Pts',(-0.190792285300657,0.778947632438904,
-0.287070292471373));
#67099=CARTESIAN_POINT('Ctrl Pts',(-0.0570527832387434,0.799941304666074,
-0.292350996947451));
#67100=CARTESIAN_POINT('Ctrl Pts',(0.0735856500869722,0.787737861403673,
-0.29763170142353));
#67101=CARTESIAN_POINT('Ctrl Pts',(0.204224083412692,0.775534418141272,
-0.302912405899608));
#67102=CARTESIAN_POINT('Ctrl Pts',(0.331761448002213,0.730133859389297,
-0.308193110375687));
#67103=CARTESIAN_POINT('Ctrl Pts',(0.440725603578711,0.657043932549396,
-0.313473814851765));
#67104=CARTESIAN_POINT('Ctrl Pts',(0.549689759155209,0.583954005709496,
-0.318754519327844));
#67105=CARTESIAN_POINT('Ctrl Pts',(0.640080705718686,0.483174710781668,
-0.324035223803922));
#67106=CARTESIAN_POINT('Ctrl Pts',(0.700932709326926,0.366932041549318,
-0.32931592828));
#67107=CARTESIAN_POINT('Ctrl Pts',(0.761784712935166,0.250689372316969,
-0.334596632756079));
#67108=CARTESIAN_POINT('Ctrl Pts',(0.793097773588171,0.118983328780098,
-0.339877337232157));
#67109=CARTESIAN_POINT('Ctrl Pts',(0.791073160808736,-0.0122082313716788,
-0.345158041708236));
#67110=CARTESIAN_POINT('Ctrl Pts',(0.789048548029301,-0.143399791523455,
-0.350438746184314));
#67111=CARTESIAN_POINT('Ctrl Pts',(0.753686261817425,-0.274076868290138,
-0.355719450660393));
#67112=CARTESIAN_POINT('Ctrl Pts',(0.689276262087855,-0.38838643245431,
-0.361000155136471));
#67113=CARTESIAN_POINT('Ctrl Pts',(0.624866262358284,-0.502695996618483,
-0.36628085961255));
#67114=CARTESIAN_POINT('Ctrl Pts',(0.531408549111018,-0.600638048180145,
-0.371561564088628));
#67115=CARTESIAN_POINT('Ctrl Pts',(0.420240901370344,-0.670330792452888,
-0.376842268564706));
#67116=CARTESIAN_POINT('Ctrl Pts',(0.309073253629671,-0.74002353672563,
-0.382122973040785));
#67117=CARTESIAN_POINT('Ctrl Pts',(0.180195671395589,-0.781466973709453,
-0.387403677516863));
#67118=CARTESIAN_POINT('Ctrl Pts',(0.049242879117497,-0.789633411989491,
-0.392684381992942));
#67119=CARTESIAN_POINT('Ctrl Pts',(-0.0817099131605952,-0.79779985026953,
-0.39796508646902));
#67120=CARTESIAN_POINT('Ctrl Pts',(-0.214737915482698,-0.772689289845784,
-0.403245790945098));
#67121=CARTESIAN_POINT('Ctrl Pts',(-0.333702897304227,-0.717348006756114,
-0.408526495421177));
#67122=CARTESIAN_POINT('Ctrl Pts',(-0.452667879125756,-0.662006723666444,
-0.413807199897256));
#67123=CARTESIAN_POINT('Ctrl Pts',(-0.557569840446711,-0.576434717910848,
-0.419087904373334));
#67124=CARTESIAN_POINT('Ctrl Pts',(-0.635682648284223,-0.471013117809877,
-0.424368608849413));
#67125=CARTESIAN_POINT('Ctrl Pts',(-0.713795456121733,-0.365591517708909,
-0.429649313325491));
#67126=CARTESIAN_POINT('Ctrl Pts',(-0.765119110475802,-0.240320323262568,
-0.434930017801569));
#67127=CARTESIAN_POINT('Ctrl Pts',(-0.783427305959389,-0.110396751522529,
-0.440210722277647));
#67128=CARTESIAN_POINT('Ctrl Pts',(-0.788577101327898,-0.0738513798824403,
-0.44169609791053));
#67129=CARTESIAN_POINT('Ctrl Pts',(-0.791114698046889,-0.0369379099605336,
-0.443181473543413));
#67130=CARTESIAN_POINT('Ctrl Pts',(-0.791079804116067,-1.96820758422422E-5,
-0.444666849176296));
#67131=CARTESIAN_POINT('Ctrl Pts',(-0.791093201014614,-2.03057722054419E-5,
-0.473133150823703));
#67132=CARTESIAN_POINT('Ctrl Pts',(-0.791125803990136,-0.0324837928275328,
-0.471826944566391));
#67133=CARTESIAN_POINT('Ctrl Pts',(-0.789165032446283,-0.0649433675248466,
-0.470520738309078));
#67134=CARTESIAN_POINT('Ctrl Pts',(-0.785179715610441,-0.0971524396805776,
-0.469214532051765));
#67135=CARTESIAN_POINT('Ctrl Pts',(-0.76906795658632,-0.227366631008214,
-0.463933827575687));
#67136=CARTESIAN_POINT('Ctrl Pts',(-0.719866888044401,-0.353486591317053,
-0.458653123099608));
#67137=CARTESIAN_POINT('Ctrl Pts',(-0.643545314872834,-0.460212135918921,
-0.45337241862353));
#67138=CARTESIAN_POINT('Ctrl Pts',(-0.567223741701267,-0.566937680520788,
-0.448091714147451));
#67139=CARTESIAN_POINT('Ctrl Pts',(-0.463781663900054,-0.654268809415684,
-0.442811009671373));
#67140=CARTESIAN_POINT('Ctrl Pts',(-0.345768109322771,-0.711610987069034,
-0.437530305195295));
#67141=CARTESIAN_POINT('Ctrl Pts',(-0.227754554745487,-0.768953164722383,
-0.432249600719217));
#67142=CARTESIAN_POINT('Ctrl Pts',(-0.0951695233921332,-0.796306391134186,
-0.426968896243139));
#67143=CARTESIAN_POINT('Ctrl Pts',(0.0359024929425398,-0.790352322285754,
-0.42168819176706));
#67144=CARTESIAN_POINT('Ctrl Pts',(0.16697450927722,-0.784398253437322,
-0.416407487290981));
#67145=CARTESIAN_POINT('Ctrl Pts',(0.29653351059322,-0.74513688932865,-0.411126782814903));
#67146=CARTESIAN_POINT('Ctrl Pts',(0.408862106534589,-0.67733120419888,
-0.405846078338824));
#67147=CARTESIAN_POINT('Ctrl Pts',(0.521190702475954,-0.609525519069113,
-0.400565373862746));
#67148=CARTESIAN_POINT('Ctrl Pts',(0.616288893042691,-0.513175512918248,
-0.395284669386668));
#67149=CARTESIAN_POINT('Ctrl Pts',(0.682619885199034,-0.399969842206072,
-0.390003964910589));
#67150=CARTESIAN_POINT('Ctrl Pts',(0.748950877355374,-0.286764171493899,
-0.384723260434511));
#67151=CARTESIAN_POINT('Ctrl Pts',(0.786514671101322,-0.156702836220414,
-0.379442555958432));
#67152=CARTESIAN_POINT('Ctrl Pts',(0.790754232170835,-0.025564167156415,
-0.374161851482354));
#67153=CARTESIAN_POINT('Ctrl Pts',(0.794993793240347,0.105574501907587,
-0.368881147006275));
#67154=CARTESIAN_POINT('Ctrl Pts',(0.765909121633421,0.237790504762104,
-0.363600442530197));
#67155=CARTESIAN_POINT('Ctrl Pts',(0.707028610824429,0.355044118136598,
-0.358319738054119));
#67156=CARTESIAN_POINT('Ctrl Pts',(0.648148100015436,0.472297731511095,
-0.35303903357804));
#67157=CARTESIAN_POINT('Ctrl Pts',(0.559471750004376,0.57458895540557,-0.347758329101962));
#67158=CARTESIAN_POINT('Ctrl Pts',(0.451757291238583,0.6495083772731,-0.342477624625883));
#67159=CARTESIAN_POINT('Ctrl Pts',(0.34404283247279,0.72442779914063,-0.337196920149804));
#67160=CARTESIAN_POINT('Ctrl Pts',(0.217290264952266,0.771975418981217,
-0.331916215673726));
#67161=CARTESIAN_POINT('Ctrl Pts',(0.086876517748351,0.786383019276778,
-0.326635511197647));
#67162=CARTESIAN_POINT('Ctrl Pts',(-0.0435372294555523,0.800790619572338,
-0.321354806721569));
#67163=CARTESIAN_POINT('Ctrl Pts',(-0.177612156342845,0.782058200322878,
-0.316074102245491));
#67164=CARTESIAN_POINT('Ctrl Pts',(-0.299083024998013,0.732458276301435,
-0.310793397769413));
#67165=CARTESIAN_POINT('Ctrl Pts',(-0.420553893653188,0.682858352279989,
-0.305512693293334));
#67166=CARTESIAN_POINT('Ctrl Pts',(-0.529420704076237,0.602390923486555,
-0.300231988817256));
#67167=CARTESIAN_POINT('Ctrl Pts',(-0.612476329745163,0.500817858869168,
-0.294951284341177));
#67168=CARTESIAN_POINT('Ctrl Pts',(-0.69553195541409,0.399244794251781,
-0.289670579865099));
#67169=CARTESIAN_POINT('Ctrl Pts',(-0.752776396328893,0.276566093810441,
-0.284389875389021));
#67170=CARTESIAN_POINT('Ctrl Pts',(-0.777265069084892,0.147664467346652,
-0.279109170912942));
#67171=CARTESIAN_POINT('Ctrl Pts',(-0.786502775973659,0.0990397233835045,
-0.277117164216529));
#67172=CARTESIAN_POINT('Ctrl Pts',(-0.791079412605933,0.049529471400793,
-0.275125157520117));
#67173=CARTESIAN_POINT('Ctrl Pts',(-0.791048813772023,1.36328575649638E-5,
-0.273133150823704));
#67174=CARTESIAN_POINT('Origin',(0.,0.,-1.425));
#67175=CARTESIAN_POINT('',(-0.7911,-9.68818082805471E-17,-0.0600000000000001));
#67176=CARTESIAN_POINT('',(-0.79116656670867,1.93884184799344E-7,-0.0731331508237035));
#67177=CARTESIAN_POINT('',(-0.7911,-9.68818082805471E-17,-1.425));
#67178=CARTESIAN_POINT('',(-0.701077753000064,0.366509473613413,-0.0600000000000001));
#67179=CARTESIAN_POINT('Origin',(0.,0.,-0.0600000000000001));
#67180=CARTESIAN_POINT('Ctrl Pts',(-0.701077753000059,0.366509473613423,
-0.0600000000000005));
#67181=CARTESIAN_POINT('Ctrl Pts',(-0.640274482293033,0.4828170276367,-0.0652807044760789));
#67182=CARTESIAN_POINT('Ctrl Pts',(-0.550002542754869,0.58364484092056,
-0.0705614089521573));
#67183=CARTESIAN_POINT('Ctrl Pts',(-0.441098388580055,0.656795701812313,
-0.0758421134282357));
#67184=CARTESIAN_POINT('Ctrl Pts',(-0.332194234405237,0.729946562704068,
-0.0811228179043143));
#67185=CARTESIAN_POINT('Ctrl Pts',(-0.204657865593779,0.775420471203709,
-0.0864035223803925));
#67186=CARTESIAN_POINT('Ctrl Pts',(-0.0740199674866195,0.787697328927234,
-0.0916842268564711));
#67187=CARTESIAN_POINT('Ctrl Pts',(0.0566179306205331,0.799974186650757,
-0.0969649313325495));
#67188=CARTESIAN_POINT('Ctrl Pts',(0.190357358023387,0.77905399359816,-0.102245635808628));
#67189=CARTESIAN_POINT('Ctrl Pts',(0.310999283790884,0.727477099691021,
-0.107526340284706));
#67190=CARTESIAN_POINT('Ctrl Pts',(0.431641209558384,0.67590020578388,-0.112807044760785));
#67191=CARTESIAN_POINT('Ctrl Pts',(0.539185633690539,0.593666611022195,
-0.118087749236863));
#67192=CARTESIAN_POINT('Ctrl Pts',(0.620573231636201,0.490751159083177,
-0.123368453712942));
#67193=CARTESIAN_POINT('Ctrl Pts',(0.701960829581863,0.387835707144159,
-0.12864915818902));
#67194=CARTESIAN_POINT('Ctrl Pts',(0.757191601341032,0.264238398027809,
-0.133929862665099));
#67195=CARTESIAN_POINT('Ctrl Pts',(0.779571649374987,0.134954042504121,
-0.139210567141177));
#67196=CARTESIAN_POINT('Ctrl Pts',(0.801951697408941,0.0056696869804328,
-0.144491271617255));
#67197=CARTESIAN_POINT('Ctrl Pts',(0.791481021717682,-0.129301714950592,
-0.149771976093334));
#67198=CARTESIAN_POINT('Ctrl Pts',(0.749426610355531,-0.253586506955687,
-0.155052680569412));
#67199=CARTESIAN_POINT('Ctrl Pts',(0.70737219899338,-0.377871298960781,
-0.160333385045491));
#67200=CARTESIAN_POINT('Ctrl Pts',(0.633734051960338,-0.491469481039944,
-0.165614089521569));
#67201=CARTESIAN_POINT('Ctrl Pts',(0.537447206462403,-0.580599770531476,
-0.170894793997648));
#67202=CARTESIAN_POINT('Ctrl Pts',(0.441160360964469,-0.669730060023005,
-0.176175498473726));
#67203=CARTESIAN_POINT('Ctrl Pts',(0.322224817001643,-0.734392456926904,
-0.181456202949804));
#67204=CARTESIAN_POINT('Ctrl Pts',(0.195068339550481,-0.766742559953149,
-0.186736907425883));
#67205=CARTESIAN_POINT('Ctrl Pts',(0.0679118620993177,-0.799092662979395,
-0.192017611901961));
#67206=CARTESIAN_POINT('Ctrl Pts',(-0.0674655488401824,-0.799130472127987,
-0.197298316378039));
#67207=CARTESIAN_POINT('Ctrl Pts',(-0.194640214369627,-0.766851356011745,
-0.202579020854118));
#67208=CARTESIAN_POINT('Ctrl Pts',(-0.321814879899078,-0.734572239895501,
-0.207859725330196));
#67209=CARTESIAN_POINT('Ctrl Pts',(-0.440786800018474,-0.669976198514418,
-0.213140429806275));
#67210=CARTESIAN_POINT('Ctrl Pts',(-0.537123170784641,-0.580899693490615,
-0.218421134282353));
#67211=CARTESIAN_POINT('Ctrl Pts',(-0.633459541550805,-0.491823188466814,
-0.223701838758432));
#67212=CARTESIAN_POINT('Ctrl Pts',(-0.707160362963742,-0.378266219800294,
-0.22898254323451));
#67213=CARTESIAN_POINT('Ctrl Pts',(-0.749284542064215,-0.254004887077675,
-0.234263247710589));
#67214=CARTESIAN_POINT('Ctrl Pts',(-0.776947718029759,-0.172401798632439,
-0.237731114865824));
#67215=CARTESIAN_POINT('Ctrl Pts',(-0.790993088555972,-0.0861823248975552,
-0.24119898202106));
#67216=CARTESIAN_POINT('Ctrl Pts',(-0.791058280240756,1.64158700123596E-5,
-0.244666849176296));
#67217=CARTESIAN_POINT('Ctrl Pts',(-0.791048813772023,1.36328575649638E-5,
-0.273133150823704));
#67218=CARTESIAN_POINT('Ctrl Pts',(-0.790998296714364,-0.0817343997010853,
-0.269844453044038));
#67219=CARTESIAN_POINT('Ctrl Pts',(-0.778390176603752,-0.163497659137093,
-0.266555755264372));
#67220=CARTESIAN_POINT('Ctrl Pts',(-0.753466702744765,-0.24131661741456,
-0.263267057484707));
#67221=CARTESIAN_POINT('Ctrl Pts',(-0.713446759051444,-0.366271523225744,
-0.257986353008628));
#67222=CARTESIAN_POINT('Ctrl Pts',(-0.641673967067604,-0.481056782361877,
-0.25270564853255));
#67223=CARTESIAN_POINT('Ctrl Pts',(-0.546855407894365,-0.571747274308673,
-0.247424944056471));
#67224=CARTESIAN_POINT('Ctrl Pts',(-0.452036848721127,-0.662437766255469,
-0.242144239580393));
#67225=CARTESIAN_POINT('Ctrl Pts',(-0.334172522358488,-0.72903349101293,
-0.236863535104314));
#67226=CARTESIAN_POINT('Ctrl Pts',(-0.20756108896749,-0.763455418739467,
-0.231582830628236));
#67227=CARTESIAN_POINT('Ctrl Pts',(-0.0809496555764887,-0.797877346466006,
-0.226302126152158));
#67228=CARTESIAN_POINT('Ctrl Pts',(0.0544088848428741,-0.800125477161621,
-0.221021421676079));
#67229=CARTESIAN_POINT('Ctrl Pts',(0.18209358115504,-0.769927080430184,
-0.2157407172));
#67230=CARTESIAN_POINT('Ctrl Pts',(0.309778277467199,-0.739728683698749,
-0.210460012723922));
#67231=CARTESIAN_POINT('Ctrl Pts',(0.429789129672164,-0.677083759540267,
-0.205179308247844));
#67232=CARTESIAN_POINT('Ctrl Pts',(0.52756706174467,-0.589592046913208,
-0.199898603771765));
#67233=CARTESIAN_POINT('Ctrl Pts',(0.625344993817177,-0.50210033428615,
-0.194617899295687));
#67234=CARTESIAN_POINT('Ctrl Pts',(0.700890005757226,-0.389761833190513,
-0.189337194819609));
#67235=CARTESIAN_POINT('Ctrl Pts',(0.745037418710249,-0.266204839038066,
-0.18405649034353));
#67236=CARTESIAN_POINT('Ctrl Pts',(0.789184831663272,-0.142647844885616,
-0.178775785867452));
#67237=CARTESIAN_POINT('Ctrl Pts',(0.801934645629268,-0.00787235767636212,
-0.173495081391374));
#67238=CARTESIAN_POINT('Ctrl Pts',(0.781740065251379,0.121771400732141,
-0.168214376915295));
#67239=CARTESIAN_POINT('Ctrl Pts',(0.76154548487349,0.251415159140645,-0.162933672439217));
#67240=CARTESIAN_POINT('Ctrl Pts',(0.708406510151714,0.37592718874839,-0.157652967963138));
#67241=CARTESIAN_POINT('Ctrl Pts',(0.628769784162815,0.480202362242657,
-0.15237226348706));
#67242=CARTESIAN_POINT('Ctrl Pts',(0.549133058173913,0.584477535736926,
-0.147091559010981));
#67243=CARTESIAN_POINT('Ctrl Pts',(0.442998580917885,0.668515853117719,
-0.141810854534903));
#67244=CARTESIAN_POINT('Ctrl Pts',(0.323241785950906,0.722122260438018,
-0.136530150058825));
#67245=CARTESIAN_POINT('Ctrl Pts',(0.203484990983934,0.775728667758313,
-0.131249445582746));
#67246=CARTESIAN_POINT('Ctrl Pts',(0.0701058783059993,0.79890316501812,
-0.125968741106667));
#67247=CARTESIAN_POINT('Ctrl Pts',(-0.0607142922230027,0.788834318036469,
-0.120688036630589));
#67248=CARTESIAN_POINT('Ctrl Pts',(-0.191534462752012,0.778765471054817,
-0.11540733215451));
#67249=CARTESIAN_POINT('Ctrl Pts',(-0.319795691132091,0.735453279831711,
-0.110126627678432));
#67250=CARTESIAN_POINT('Ctrl Pts',(-0.429938877917322,0.664152203157782,
-0.104845923202354));
#67251=CARTESIAN_POINT('Ctrl Pts',(-0.54008206470255,0.592851126483854,
-0.0995652187262753));
#67252=CARTESIAN_POINT('Ctrl Pts',(-0.632107209892923,0.493561164359106,
-0.0942845142501968));
#67253=CARTESIAN_POINT('Ctrl Pts',(-0.694848653928772,0.378327514286356,
-0.0890038097741183));
#67254=CARTESIAN_POINT('Ctrl Pts',(-0.757703150259721,0.262886227478213,
-0.0837135901239801));
#67255=CARTESIAN_POINT('Ctrl Pts',(-0.791168292937371,0.13144374384189,
-0.0784233704738418));
#67256=CARTESIAN_POINT('Ctrl Pts',(-0.79116656670867,1.93884184799344E-7,
-0.0731331508237035));
#67257=CARTESIAN_POINT('Origin',(0.,0.,-3.278617978381));
#67258=CARTESIAN_POINT('',(-0.676664313283933,1.40419911898121E-5,-0.178617978381002));
#67259=CARTESIAN_POINT('',(-0.676756940578634,1.65846773781623E-7,-0.139182021618995));
#67260=CARTESIAN_POINT('',(-0.6767,-6.21087748740391E-14,-3.278617978381));
#67261=CARTESIAN_POINT('',(0.564220937616133,0.373642629516334,-0.06));
#67262=CARTESIAN_POINT('Ctrl Pts',(-0.676664313283933,1.40419911898067E-5,
-0.178617978381002));
#67263=CARTESIAN_POINT('Ctrl Pts',(-0.676608548888669,-0.0737196046747348,
-0.175150111225766));
#67264=CARTESIAN_POINT('Ctrl Pts',(-0.646299473199053,-0.259776109946148,
-0.166401539594452));
#67265=CARTESIAN_POINT('Ctrl Pts',(-0.478812698669308,-0.517836875656849,
-0.15237226348706));
#67266=CARTESIAN_POINT('Ctrl Pts',(-0.173510088336382,-0.683601537024222,
-0.136530150058825));
#67267=CARTESIAN_POINT('Ctrl Pts',(0.173891860782926,-0.683504512182157,
-0.120688036630589));
#67268=CARTESIAN_POINT('Ctrl Pts',(0.479101123580215,-0.517569571018445,
-0.104845923202354));
#67269=CARTESIAN_POINT('Ctrl Pts',(0.668069398503454,-0.226056905819471,
-0.0890038097741189));
#67270=CARTESIAN_POINT('Ctrl Pts',(0.693423565747112,0.100768945594041,
-0.0740551687066675));
#67271=CARTESIAN_POINT('Ctrl Pts',(0.615633638736097,0.295835894939612,
-0.0643872321152945));
#67272=CARTESIAN_POINT('Ctrl Pts',(0.564220937616133,0.373642629516334,
-0.06));
#67273=CARTESIAN_POINT('',(0.5370608629359,-0.411689834101531,-0.0600000000000001));
#67274=CARTESIAN_POINT('Origin',(0.,0.,-0.0600000000000001));
#67275=CARTESIAN_POINT('Ctrl Pts',(-0.676756940578634,1.65846773778668E-7,
-0.139182021618995));
#67276=CARTESIAN_POINT('Ctrl Pts',(-0.67675546928947,-0.112031032267847,
-0.133910832316977));
#67277=CARTESIAN_POINT('Ctrl Pts',(-0.619882615330693,-0.336297451995222,
-0.123358938538881));
#67278=CARTESIAN_POINT('Ctrl Pts',(-0.384315741505486,-0.591363827723695,
-0.107526340284706));
#67279=CARTESIAN_POINT('Ctrl Pts',(-0.055404374357266,-0.703098282770509,
-0.091684226856471));
#67280=CARTESIAN_POINT('Ctrl Pts',(0.287037892597339,-0.644247893625522,
-0.0758421134282355));
#67281=CARTESIAN_POINT('Ctrl Pts',(0.468762250669717,-0.500787277377127,
-0.0652807044760785));
#67282=CARTESIAN_POINT('Ctrl Pts',(0.5370608629359,-0.411689834101531,-0.0600000000000001));
#67283=CARTESIAN_POINT('Origin',(0.,0.,-3.278617978381));
#67284=CARTESIAN_POINT('',(-0.676682724618054,-1.68358750310745E-5,-0.378617978381002));
#67285=CARTESIAN_POINT('',(-0.676656215749625,1.16614266989223E-5,-0.339182021618995));
#67286=CARTESIAN_POINT('',(-0.6767,-6.21087748740391E-14,-3.278617978381));
#67287=CARTESIAN_POINT('Ctrl Pts',(-0.676682724618054,-1.68358750310751E-5,
-0.378617978381002));
#67288=CARTESIAN_POINT('Ctrl Pts',(-0.676712572580368,-0.031596364138927,
-0.377132602748119));
#67289=CARTESIAN_POINT('Ctrl Pts',(-0.666825032969671,-0.175426703014129,
-0.370366522639158));
#67290=CARTESIAN_POINT('Ctrl Pts',(-0.566672567635157,-0.419879657837779,
-0.358319738054119));
#67291=CARTESIAN_POINT('Ctrl Pts',(-0.297475915280626,-0.639472286942102,
-0.342477624625884));
#67292=CARTESIAN_POINT('Ctrl Pts',(0.043897043275945,-0.703910346247173,
-0.326635511197648));
#67293=CARTESIAN_POINT('Ctrl Pts',(0.374619303032495,-0.597559288958764,
-0.310793397769413));
#67294=CARTESIAN_POINT('Ctrl Pts',(0.614448027167589,-0.346222973859112,
-0.294951284341178));
#67295=CARTESIAN_POINT('Ctrl Pts',(0.70519379538744,-0.0108828985917093,
-0.279109170912942));
#67296=CARTESIAN_POINT('Ctrl Pts',(0.624839043230104,0.327097684121224,
-0.263267057484707));
#67297=CARTESIAN_POINT('Ctrl Pts',(0.392880175048439,0.585714858477159,
-0.247424944056472));
#67298=CARTESIAN_POINT('Ctrl Pts',(0.0655971465397984,0.70222057750431,
-0.231582830628236));
#67299=CARTESIAN_POINT('Ctrl Pts',(-0.277601643923981,0.6483471683419,-0.215740717200002));
#67300=CARTESIAN_POINT('Ctrl Pts',(-0.553446229800004,0.437165882444832,
-0.199898603771766));
#67301=CARTESIAN_POINT('Ctrl Pts',(-0.664020356520139,0.189362139227846,
-0.187524357498766));
#67302=CARTESIAN_POINT('Ctrl Pts',(-0.676693464278589,0.0385585134182499,
-0.180430815701845));
#67303=CARTESIAN_POINT('Ctrl Pts',(-0.676664313283933,1.40419911898067E-5,
-0.178617978381002));
#67304=CARTESIAN_POINT('Ctrl Pts',(-0.676656215749625,1.16614266988981E-5,
-0.339182021618994));
#67305=CARTESIAN_POINT('Ctrl Pts',(-0.676613003901662,-0.0699148884815599,
-0.33589332383933));
#67306=CARTESIAN_POINT('Ctrl Pts',(-0.648510715023198,-0.25215734145285,
-0.327323921583586));
#67307=CARTESIAN_POINT('Ctrl Pts',(-0.487488465654378,-0.509678055216417,
-0.313473814851765));
#67308=CARTESIAN_POINT('Ctrl Pts',(-0.185028133270616,-0.680574251437019,
-0.297631701423529));
#67309=CARTESIAN_POINT('Ctrl Pts',(0.162325390816526,-0.68634334526228,
-0.281789587995294));
#67310=CARTESIAN_POINT('Ctrl Pts',(0.470294081325063,-0.525585589562447,
-0.265947474567059));
#67311=CARTESIAN_POINT('Ctrl Pts',(0.664155702788206,-0.237305484551378,
-0.250105361138824));
#67312=CARTESIAN_POINT('Ctrl Pts',(0.696873939840873,0.108551823732687,
-0.234263247710588));
#67313=CARTESIAN_POINT('Ctrl Pts',(0.560510101409974,0.428071317231208,
-0.218421134282353));
#67314=CARTESIAN_POINT('Ctrl Pts',(0.288150599099951,0.643728235591383,
-0.202579020854118));
#67315=CARTESIAN_POINT('Ctrl Pts',(-0.0541233696112858,0.703198020558049,
-0.186736907425882));
#67316=CARTESIAN_POINT('Ctrl Pts',(-0.383263958328779,0.592051415322255,
-0.170894793997647));
#67317=CARTESIAN_POINT('Ctrl Pts',(-0.61941646401829,0.337256127609639,
-0.155052680569412));
#67318=CARTESIAN_POINT('Ctrl Pts',(-0.676706952231611,0.112638054466167,
-0.144481756443194));
#67319=CARTESIAN_POINT('Ctrl Pts',(-0.6767569432345,0.000202396555859588,
-0.139191536793055));
#67320=CARTESIAN_POINT('Ctrl Pts',(-0.676756940578634,1.65846773778668E-7,
-0.139182021618995));
#67321=CARTESIAN_POINT('Origin',(0.,0.,-3.278617978381));
#67322=CARTESIAN_POINT('',(-0.676744415355718,1.02840190608962E-5,-0.578617978381002));
#67323=CARTESIAN_POINT('',(-0.676694184207546,-1.73693794768559E-5,-0.539182021618994));
#67324=CARTESIAN_POINT('',(-0.6767,-6.21087748740391E-14,-3.278617978381));
#67325=CARTESIAN_POINT('Ctrl Pts',(-0.676744415355718,1.02840190609223E-5,
-0.578617978381002));
#67326=CARTESIAN_POINT('Ctrl Pts',(-0.676669814511743,-0.101663497973202,
-0.573834389794394));
#67327=CARTESIAN_POINT('Ctrl Pts',(-0.62778641803666,-0.315646428609378,
-0.563770096731707));
#67328=CARTESIAN_POINT('Ctrl Pts',(-0.411086852200351,-0.573083175383003,
-0.548425099192943));
#67329=CARTESIAN_POINT('Ctrl Pts',(-0.0876254735054571,-0.699813191038862,
-0.532582985764706));
#67330=CARTESIAN_POINT('Ctrl Pts',(0.257096392819387,-0.656748179105437,
-0.516740872336472));
#67331=CARTESIAN_POINT('Ctrl Pts',(0.539439199031029,-0.454336963616046,
-0.500898758908236));
#67332=CARTESIAN_POINT('Ctrl Pts',(0.690898371074035,-0.141690390662916,
-0.485056645480001));
#67333=CARTESIAN_POINT('Ctrl Pts',(0.67472551005466,0.205334390789043,-0.469214532051766));
#67334=CARTESIAN_POINT('Ctrl Pts',(0.494844622289992,0.502539078828164,
-0.45337241862353));
#67335=CARTESIAN_POINT('Ctrl Pts',(0.194900041286442,0.67781317475087,-0.437530305195295));
#67336=CARTESIAN_POINT('Ctrl Pts',(-0.152332956558304,0.688630086697795,
-0.42168819176706));
#67337=CARTESIAN_POINT('Ctrl Pts',(-0.462605549975718,0.532365317323737,
-0.405846078338825));
#67338=CARTESIAN_POINT('Ctrl Pts',(-0.642068958012134,0.273695698164427,
-0.391489340543472));
#67339=CARTESIAN_POINT('Ctrl Pts',(-0.676606459173965,0.080672985488116,
-0.382413307224198));
#67340=CARTESIAN_POINT('Ctrl Pts',(-0.676682724618054,-1.68358750310751E-5,
-0.378617978381002));
#67341=CARTESIAN_POINT('Ctrl Pts',(-0.676694184207546,-1.73693794768663E-5,
-0.539182021618994));
#67342=CARTESIAN_POINT('Ctrl Pts',(-0.676722072506792,-0.0277863514175533,
-0.537875815361682));
#67343=CARTESIAN_POINT('Ctrl Pts',(-0.668264186930468,-0.167802341299913,
-0.531288904628292));
#67344=CARTESIAN_POINT('Ctrl Pts',(-0.573681658522724,-0.410251236866699,
-0.519421289418823));
#67345=CARTESIAN_POINT('Ctrl Pts',(-0.308231320835643,-0.634358081474877,
-0.503579175990589));
#67346=CARTESIAN_POINT('Ctrl Pts',(0.032004897278945,-0.704551211216498,
-0.487737062562353));
#67347=CARTESIAN_POINT('Ctrl Pts',(0.364475796750062,-0.603799731912975,
-0.471894949134118));
#67348=CARTESIAN_POINT('Ctrl Pts',(0.60851427060865,-0.356548881847406,
-0.456052835705882));
#67349=CARTESIAN_POINT('Ctrl Pts',(0.704909489523639,-0.0227889061948828,
-0.440210722277648));
#67350=CARTESIAN_POINT('Ctrl Pts',(0.630273170690079,0.316500320697992,
-0.424368608849411));
#67351=CARTESIAN_POINT('Ctrl Pts',(0.402714255056845,0.578997367377502,
-0.408526495421177));
#67352=CARTESIAN_POINT('Ctrl Pts',(0.0774451521325488,0.701012818064358,
-0.39268438199294));
#67353=CARTESIAN_POINT('Ctrl Pts',(-0.26661439669049,0.652942176782176,
-0.376842268564707));
#67354=CARTESIAN_POINT('Ctrl Pts',(-0.545985540464761,0.446448778736983,
-0.36100015513647));
#67355=CARTESIAN_POINT('Ctrl Pts',(-0.662389607688161,0.196987006295065,
-0.348446739487901));
#67356=CARTESIAN_POINT('Ctrl Pts',(-0.676682389723724,0.0423670753341918,
-0.341174028315408));
#67357=CARTESIAN_POINT('Ctrl Pts',(-0.676656215749625,1.16614266988981E-5,
-0.339182021618994));
#67358=CARTESIAN_POINT('Origin',(0.,0.,-3.278617978381));
#67359=CARTESIAN_POINT('',(-0.67664350881809,3.14251806171502E-6,-0.778617978381002));
#67360=CARTESIAN_POINT('',(-0.676734930268368,1.31228392115518E-5,-0.739182021618995));
#67361=CARTESIAN_POINT('',(-0.6767,-6.21087748740391E-14,-3.278617978381));
#67362=CARTESIAN_POINT('Ctrl Pts',(-0.67664350881809,3.14251806169882E-6,
-0.778617978381002));
#67363=CARTESIAN_POINT('Ctrl Pts',(-0.676633824259794,-0.0595589089414728,
-0.775816881316747));
#67364=CARTESIAN_POINT('Ctrl Pts',(-0.654163529573119,-0.231416130782925,
-0.767735079776413));
#67365=CARTESIAN_POINT('Ctrl Pts',(-0.510387952556461,-0.48674517341652,
-0.754372573760001));
#67366=CARTESIAN_POINT('Ctrl Pts',(-0.216097768239373,-0.671355703424805,
-0.738530460331765));
#67367=CARTESIAN_POINT('Ctrl Pts',(0.13062401781091,-0.693075819755666,
-0.722688346903532));
#67368=CARTESIAN_POINT('Ctrl Pts',(0.445652619177005,-0.546635590663221,
-0.706846233475294));
#67369=CARTESIAN_POINT('Ctrl Pts',(0.652552937542223,-0.267565673553371,
-0.69100412004706));
#67370=CARTESIAN_POINT('Ctrl Pts',(0.701124939933614,0.0764234555757611,
-0.675162006618824));
#67371=CARTESIAN_POINT('Ctrl Pts',(0.579583646314047,0.401870032329318,
-0.659319893190589));
#67372=CARTESIAN_POINT('Ctrl Pts',(0.317418508393823,0.629811254653404,
-0.643477779762354));
#67373=CARTESIAN_POINT('Ctrl Pts',(-0.0217615887758392,0.704941954499094,
-0.627635666334118));
#67374=CARTESIAN_POINT('Ctrl Pts',(-0.355661691778637,0.609033239618506,
-0.611793552905885));
#67375=CARTESIAN_POINT('Ctrl Pts',(-0.603267927301802,0.365355352838904,
-0.595951439477647));
#67376=CARTESIAN_POINT('Ctrl Pts',(-0.673935245528764,0.133378091047515,
-0.584892914636021));
#67377=CARTESIAN_POINT('Ctrl Pts',(-0.676752167959069,0.0105763374443912,
-0.579115094270472));
#67378=CARTESIAN_POINT('Ctrl Pts',(-0.676744415355718,1.02840190609223E-5,
-0.578617978381002));
#67379=CARTESIAN_POINT('Ctrl Pts',(-0.676734930268368,1.31228392115622E-5,
-0.739182021618995));
#67380=CARTESIAN_POINT('Ctrl Pts',(-0.676648595874367,-0.0978564382041463,
-0.734577602407957));
#67381=CARTESIAN_POINT('Ctrl Pts',(-0.630547679361052,-0.30804907633827,
-0.724692478720841));
#67382=CARTESIAN_POINT('Ctrl Pts',(-0.420705045567162,-0.56606005627552,
-0.709526650557648));
#67383=CARTESIAN_POINT('Ctrl Pts',(-0.0994296853315642,-0.69823381495827,
-0.693684537129411));
#67384=CARTESIAN_POINT('Ctrl Pts',(0.245970207536815,-0.660995748610087,
-0.677842423701176));
#67385=CARTESIAN_POINT('Ctrl Pts',(0.531690576341267,-0.46338089484376,
-0.662000310272941));
#67386=CARTESIAN_POINT('Ctrl Pts',(0.688407352137116,-0.153336362940691,
-0.646158196844705));
#67387=CARTESIAN_POINT('Ctrl Pts',(0.678096488492109,0.193912028948647,
-0.630316083416472));
#67388=CARTESIAN_POINT('Ctrl Pts',(0.503259700720423,0.494111724518966,
-0.614473969988234));
#67389=CARTESIAN_POINT('Ctrl Pts',(0.206317477008665,0.674425549158015,
-0.598631856560001));
#67390=CARTESIAN_POINT('Ctrl Pts',(-0.140683365416483,0.691104126287348,
-0.582789743131764));
#67391=CARTESIAN_POINT('Ctrl Pts',(-0.453550332947481,0.540100748156837,
-0.56694762970353));
#67392=CARTESIAN_POINT('Ctrl Pts',(-0.639649782541237,0.281308470484841,
-0.552411722532606));
#67393=CARTESIAN_POINT('Ctrl Pts',(-0.67660932624958,0.0844775325776096,
-0.543156519837761));
#67394=CARTESIAN_POINT('Ctrl Pts',(-0.676694184207546,-1.73693794768663E-5,
-0.539182021618994));
#67395=CARTESIAN_POINT('Origin',(0.,0.,-3.278617978381));
#67396=CARTESIAN_POINT('',(-0.676726354840372,-1.49018706585343E-5,-0.978617978381004));
#67397=CARTESIAN_POINT('',(-0.676642658803801,-3.62091512329243E-7,-0.939182021618995));
#67398=CARTESIAN_POINT('',(-0.6767,-6.21087748740391E-14,-3.278617978381));
#67399=CARTESIAN_POINT('Ctrl Pts',(-0.676726354840372,-1.49018706585916E-5,
-0.978617978381004));
#67400=CARTESIAN_POINT('Ctrl Pts',(-0.676743078776964,-0.0174154680940201,
-0.977799372839101));
#67401=CARTESIAN_POINT('Ctrl Pts',(-0.6718429949253,-0.14705514285169,-0.97170006282112));
#67402=CARTESIAN_POINT('Ctrl Pts',(-0.591922568453257,-0.383463686565954,
-0.960320048327059));
#67403=CARTESIAN_POINT('Ctrl Pts',(-0.337047750540382,-0.619528481843024,
-0.944477934898826));
#67404=CARTESIAN_POINT('Ctrl Pts',(-0.000395348502580347,-0.705277654302627,
-0.928635821470588));
#67405=CARTESIAN_POINT('Ctrl Pts',(0.336352976576915,-0.619905961502954,
-0.912793708042355));
#67406=CARTESIAN_POINT('Ctrl Pts',(0.59149228989595,-0.384127058344892,
-0.896951594614118));
#67407=CARTESIAN_POINT('Ctrl Pts',(0.703118375731167,-0.0551477621324492,
-0.881109481185884));
#67408=CARTESIAN_POINT('Ctrl Pts',(0.644147500070733,0.287211984624038,
-0.865267367757648));
#67409=CARTESIAN_POINT('Ctrl Pts',(0.428887711959651,0.559885753068489,
-0.849425254329413));
#67410=CARTESIAN_POINT('Ctrl Pts',(0.109567294787274,0.696714958840452,
-0.833583140901177));
#67411=CARTESIAN_POINT('Ctrl Pts',(-0.236337333828263,0.664500858237221,
-0.817741027472942));
#67412=CARTESIAN_POINT('Ctrl Pts',(-0.524899653622529,0.471059528707363,
-0.801898914044707));
#67413=CARTESIAN_POINT('Ctrl Pts',(-0.657602612550172,0.217736950995035,
-0.788857897680726));
#67414=CARTESIAN_POINT('Ctrl Pts',(-0.676652081852862,0.0527290926991997,
-0.781097585792825));
#67415=CARTESIAN_POINT('Ctrl Pts',(-0.67664350881809,3.14251806169882E-6,
-0.778617978381002));
#67416=CARTESIAN_POINT('Ctrl Pts',(-0.676642658803801,-3.62091512332713E-7,
-0.939182021618995));
#67417=CARTESIAN_POINT('Ctrl Pts',(-0.676643701727751,-0.0557527860905397,
-0.93656009393031));
#67418=CARTESIAN_POINT('Ctrl Pts',(-0.656108130744977,-0.223792859010719,
-0.928657461765547));
#67419=CARTESIAN_POINT('Ctrl Pts',(-0.518534126716599,-0.478057613794162,
-0.915474125124705));
#67420=CARTESIAN_POINT('Ctrl Pts',(-0.22740314400511,-0.66761106399827,
-0.89963201169647));
#67421=CARTESIAN_POINT('Ctrl Pts',(0.118902453310195,-0.695182658927227,
-0.883789898268235));
#67422=CARTESIAN_POINT('Ctrl Pts',(0.436358858299948,-0.55408272799238,
-0.86794778484));
#67423=CARTESIAN_POINT('Ctrl Pts',(0.647941916898673,-0.278546216994571,
-0.852105671411764));
#67424=CARTESIAN_POINT('Ctrl Pts',(0.702315427199591,0.0645737051265365,
-0.836263557983531));
#67425=CARTESIAN_POINT('Ctrl Pts',(0.586286794664772,0.392026168868892,
-0.820421444555292));
#67426=CARTESIAN_POINT('Ctrl Pts',(0.328007939141782,0.624361685672875,
-0.804579331127061));
#67427=CARTESIAN_POINT('Ctrl Pts',(-0.00985517942347469,0.705208903882278,
-0.788737217698822));
#67428=CARTESIAN_POINT('Ctrl Pts',(-0.345327144915973,0.614951937683339,
-0.772895104270589));
#67429=CARTESIAN_POINT('Ctrl Pts',(-0.597012704480207,0.375489751345548,
-0.757052990842353));
#67430=CARTESIAN_POINT('Ctrl Pts',(-0.672795249619501,0.141000208336555,
-0.745815296625156));
#67431=CARTESIAN_POINT('Ctrl Pts',(-0.676747610842367,0.0143879525399922,
-0.739858306884036));
#67432=CARTESIAN_POINT('Ctrl Pts',(-0.676734930268368,1.31228392115622E-5,
-0.739182021618995));
#67433=CARTESIAN_POINT('Origin',(0.,0.,-3.278617978381));
#67434=CARTESIAN_POINT('',(-0.676703646557406,1.72471476807506E-5,-1.178617978381));
#67435=CARTESIAN_POINT('',(-0.676737017697599,-1.25909068602881E-5,-1.139182021619));
#67436=CARTESIAN_POINT('',(-0.6767,-6.21087748740391E-14,-3.278617978381));
#67437=CARTESIAN_POINT('Ctrl Pts',(-0.676703646557406,1.72471476807406E-5,
-1.178617978381));
#67438=CARTESIAN_POINT('Ctrl Pts',(-0.676613962442266,-0.087499758462613,
-1.17450115988537));
#67439=CARTESIAN_POINT('Ctrl Pts',(-0.637674973361225,-0.287353613941579,
-1.16510363691367));
#67440=CARTESIAN_POINT('Ctrl Pts',(-0.446265180001859,-0.546135619674237,
-1.15042540946588));
#67441=CARTESIAN_POINT('Ctrl Pts',(-0.13140095282778,-0.692928939758619,
-1.13458329603765));
#67442=CARTESIAN_POINT('Ctrl Pts',(0.215344966055381,-0.671597551777596,
-1.11874118260941));
#67443=CARTESIAN_POINT('Ctrl Pts',(0.509841934903309,-0.487317070676889,
-1.10289906918118));
#67444=CARTESIAN_POINT('Ctrl Pts',(0.680636426416433,-0.184799299225192,
-1.08705695575294));
#67445=CARTESIAN_POINT('Ctrl Pts',(0.686288731012368,0.162556155357116,
-1.07121484232471));
#67446=CARTESIAN_POINT('Ctrl Pts',(0.52542743525236,0.470470760242527,-1.05537272889647));
#67447=CARTESIAN_POINT('Ctrl Pts',(0.237082166616096,0.664235479503821,
-1.03953061546824));
#67448=CARTESIAN_POINT('Ctrl Pts',(-0.108786128932179,0.696837358435242,
-1.02368850204));
#67449=CARTESIAN_POINT('Ctrl Pts',(-0.428259746586556,0.560366233290937,
-1.00784638861177));
#67450=CARTESIAN_POINT('Ctrl Pts',(-0.632686243670446,0.302011290964289,
-0.992822880725432));
#67451=CARTESIAN_POINT('Ctrl Pts',(-0.676635195111024,0.0948330365135053,
-0.983080077315179));
#67452=CARTESIAN_POINT('Ctrl Pts',(-0.676726354840372,-1.49018706585916E-5,
-0.978617978381004));
#67453=CARTESIAN_POINT('Ctrl Pts',(-0.6767370176976,-1.25909068602707E-5,
-1.139182021619));
#67454=CARTESIAN_POINT('Ctrl Pts',(-0.676748654703403,-0.0136040506252591,
-1.13854258545266));
#67455=CARTESIAN_POINT('Ctrl Pts',(-0.673035053480589,-0.139432545494104,
-1.13262244481025));
#67456=CARTESIAN_POINT('Ctrl Pts',(-0.598313157002194,-0.373414098333714,
-1.12142159969176));
#67457=CARTESIAN_POINT('Ctrl Pts',(-0.347460752777172,-0.613748929087322,
-1.10557948626353));
#67458=CARTESIAN_POINT('Ctrl Pts',(-0.0123042673209635,-0.705170424565585,
-1.08973737283529));
#67459=CARTESIAN_POINT('Ctrl Pts',(0.32583759114047,-0.625497071836542,
-1.07389525940706));
#67460=CARTESIAN_POINT('Ctrl Pts',(0.584921776088787,-0.394059942817653,
-1.05805314597882));
#67461=CARTESIAN_POINT('Ctrl Pts',(0.702086931244113,-0.0670124141673551,
-1.04221103255059));
#67462=CARTESIAN_POINT('Ctrl Pts',(0.648905383326142,0.276294274581765,
-1.02636891912235));
#67463=CARTESIAN_POINT('Ctrl Pts',(0.438280522141762,0.552563938913369,
-1.01052680569412));
#67464=CARTESIAN_POINT('Ctrl Pts',(0.121316063044922,0.694765525572184,
-0.994684692265882));
#67465=CARTESIAN_POINT('Ctrl Pts',(-0.225083200276113,0.668396795047505,
-0.978842578837647));
#67466=CARTESIAN_POINT('Ctrl Pts',(-0.51687073479559,0.479855568049576,
-0.963000465409411));
#67467=CARTESIAN_POINT('Ctrl Pts',(-0.655713957784839,0.225360770249037,
-0.949780279669861));
#67468=CARTESIAN_POINT('Ctrl Pts',(-0.676641601222389,0.0565356176798869,
-0.941840798406389));
#67469=CARTESIAN_POINT('Ctrl Pts',(-0.676642658803801,-3.62091512332713E-7,
-0.939182021618995));
#67470=CARTESIAN_POINT('Origin',(0.,0.,-3.278617978381));
#67471=CARTESIAN_POINT('',(-0.676651018322484,-9.42764808053333E-6,-1.378617978381));
#67472=CARTESIAN_POINT('',(-0.676691774264851,1.73213003940714E-5,-1.339182021619));
#67473=CARTESIAN_POINT('',(-0.6767,-6.21087748740391E-14,-3.278617978381));
#67474=CARTESIAN_POINT('Ctrl Pts',(-0.676651018322484,-9.42764808054344E-6,
-1.378617978381));
#67475=CARTESIAN_POINT('Ctrl Pts',(-0.67667346476596,-0.045391951814263,
-1.37648365140773));
#67476=CARTESIAN_POINT('Ctrl Pts',(-0.661045351089367,-0.203043660447462,
-1.36906861995837));
#67477=CARTESIAN_POINT('Ctrl Pts',(-0.539948223619144,-0.453731905170425,
-1.35637288403294));
#67478=CARTESIAN_POINT('Ctrl Pts',(-0.257832520922968,-0.65645953196946,
-1.34053077060471));
#67479=CARTESIAN_POINT('Ctrl Pts',(0.0868408479677307,-0.699910989400294,
-1.32468865717647));
#67480=CARTESIAN_POINT('Ctrl Pts',(0.4104441021973,-0.57354369051582,-1.30884654374824));
#67481=CARTESIAN_POINT('Ctrl Pts',(0.634461683351754,-0.308018016222288,
-1.29300443032));
#67482=CARTESIAN_POINT('Ctrl Pts',(0.70454041281189,0.0322417845955294,
-1.27716231689176));
#67483=CARTESIAN_POINT('Ctrl Pts',(0.603677153234099,0.364678791023317,
-1.26132020346353));
#67484=CARTESIAN_POINT('Ctrl Pts',(0.356344264045233,0.608634119517723,
-1.2454780900353));
#67485=CARTESIAN_POINT('Ctrl Pts',(0.022551895498706,0.7049171142542,-1.22963597660706));
#67486=CARTESIAN_POINT('Ctrl Pts',(-0.316712218604248,0.630166721230049,
-1.21379386317883));
#67487=CARTESIAN_POINT('Ctrl Pts',(-0.579132739896463,0.402519559200629,
-1.19795174975059));
#67488=CARTESIAN_POINT('Ctrl Pts',(-0.669359637244422,0.16174631842112,
-1.18622645481798));
#67489=CARTESIAN_POINT('Ctrl Pts',(-0.676729001594164,0.024759609724268,
-1.17978186436145));
#67490=CARTESIAN_POINT('Ctrl Pts',(-0.676703646557406,1.72471476807406E-5,
-1.178617978381));
#67491=CARTESIAN_POINT('Ctrl Pts',(-0.676691774264851,1.73213003940645E-5,
-1.339182021619));
#67492=CARTESIAN_POINT('Ctrl Pts',(-0.676608477074042,-0.0836950532711893,
-1.33524437249894));
#67493=CARTESIAN_POINT('Ctrl Pts',(-0.640153403921032,-0.279742992602309,
-1.3260260189028));
#67494=CARTESIAN_POINT('Ctrl Pts',(-0.455423334553543,-0.538522338460017,
-1.31152696083059));
#67495=CARTESIAN_POINT('Ctrl Pts',(-0.143082679303674,-0.690611373754874,
-1.29568484740235));
#67496=CARTESIAN_POINT('Ctrl Pts',(0.203973994150782,-0.675138009881304,
-1.27984273397412));
#67497=CARTESIAN_POINT('Ctrl Pts',(0.501540645971156,-0.495856534811379,
-1.26400062054588));
#67498=CARTESIAN_POINT('Ctrl Pts',(0.677418954516088,-0.196265847101944,
-1.24815850711765));
#67499=CARTESIAN_POINT('Ctrl Pts',(0.688935728376574,0.150944641649023,
-1.23231639368941));
#67500=CARTESIAN_POINT('Ctrl Pts',(0.533296663357694,0.461531571539655,
-1.21647428026118));
#67501=CARTESIAN_POINT('Ctrl Pts',(0.248264321922183,0.660137522897185,
-1.20063216683294));
#67502=CARTESIAN_POINT('Ctrl Pts',(-0.0970041624297474,0.698574917347893,
-1.1847900534047));
#67503=CARTESIAN_POINT('Ctrl Pts',(-0.418736616528254,0.567517725410213,
-1.16894793997647));
#67504=CARTESIAN_POINT('Ctrl Pts',(-0.629986079414507,0.30961194562541,
-1.15374526271457));
#67505=CARTESIAN_POINT('Ctrl Pts',(-0.676652551930573,0.0986393380825266,
-1.14382328992874));
#67506=CARTESIAN_POINT('Ctrl Pts',(-0.6767370176976,-1.25909068602707E-5,
-1.139182021619));
#67507=CARTESIAN_POINT('Origin',(0.,0.,-3.278617978381));
#67508=CARTESIAN_POINT('',(-0.676756207239106,-3.37313647904859E-6,-1.578617978381));
#67509=CARTESIAN_POINT('',(-0.676657745381425,-1.21934319496919E-5,-1.539182021619));
#67510=CARTESIAN_POINT('',(-0.6767,-6.21087748740391E-14,-3.278617978381));
#67511=CARTESIAN_POINT('Ctrl Pts',(-0.676756207239105,-3.37313647901958E-6,
-1.578617978381));
#67512=CARTESIAN_POINT('Ctrl Pts',(-0.676757103819284,-0.00323042804578434,
-1.57846614293008));
#67513=CARTESIAN_POINT('Ctrl Pts',(-0.675948430935335,-0.118691185533526,
-1.57303360300308));
#67514=CARTESIAN_POINT('Ctrl Pts',(-0.614835796701285,-0.345533889877317,
-1.5623203586));
#67515=CARTESIAN_POINT('Ctrl Pts',(-0.375288999670649,-0.597138922433682,
-1.54647824517177));
#67516=CARTESIAN_POINT('Ctrl Pts',(-0.0446861795912879,-0.703860690273713,
-1.53063613174353));
#67517=CARTESIAN_POINT('Ctrl Pts',(0.296758806931518,-0.639805389526875,
-1.5147940183153));
#67518=CARTESIAN_POINT('Ctrl Pts',(0.566201478471519,-0.420514698596517,
-1.49895190488706));
#67519=CARTESIAN_POINT('Ctrl Pts',(0.698267208723158,-0.0991949150966095,
-1.48310979145883));
#67520=CARTESIAN_POINT('Ctrl Pts',(0.660913011645563,0.246192438951009,
-1.46726767803059));
#67521=CARTESIAN_POINT('Ctrl Pts',(0.46320210154304,0.53184634913212,-1.45142556460235));
#67522=CARTESIAN_POINT('Ctrl Pts',(0.153104893757042,0.688458871296389,
-1.43558345117412));
#67523=CARTESIAN_POINT('Ctrl Pts',(-0.194140012861185,0.678031253973823,
-1.41974133774588));
#67524=CARTESIAN_POINT('Ctrl Pts',(-0.494280907634458,0.503093540315427,
-1.40389922431765));
#67525=CARTESIAN_POINT('Ctrl Pts',(-0.650215574940587,0.246104379942304,
-1.39019143786269));
#67526=CARTESIAN_POINT('Ctrl Pts',(-0.676617928273182,0.0668924832797416,
-1.38176435588381));
#67527=CARTESIAN_POINT('Ctrl Pts',(-0.676651018322484,-9.42764808054344E-6,
-1.378617978381));
#67528=CARTESIAN_POINT('Ctrl Pts',(-0.676657745381425,-1.21934319497544E-5,
-1.539182021619));
#67529=CARTESIAN_POINT('Ctrl Pts',(-0.676684688084094,-0.0415838273109365,
-1.53722686402129));
#67530=CARTESIAN_POINT('Ctrl Pts',(-0.662730591069265,-0.195418828189768,
-1.52999100194751));
#67531=CARTESIAN_POINT('Ctrl Pts',(-0.54753273728204,-0.444549912024228,
-1.51747443539765));
#67532=CARTESIAN_POINT('Ctrl Pts',(-0.268880416908177,-0.652012303625934,
-1.50163232196941));
#67533=CARTESIAN_POINT('Ctrl Pts',(0.0750101104497115,-0.701277552761128,
-1.48579020854118));
#67534=CARTESIAN_POINT('Ctrl Pts',(0.400701004053372,-0.580392477576107,
-1.46994809511294));
#67535=CARTESIAN_POINT('Ctrl Pts',(0.629170183477428,-0.318687312109054,
-1.45410598168471));
#67536=CARTESIAN_POINT('Ctrl Pts',(0.70498438292987,0.0203406612799057,
-1.43826386825647));
#67537=CARTESIAN_POINT('Ctrl Pts',(0.609748873285091,0.354433398826739,
-1.42242175482824));
#67538=CARTESIAN_POINT('Ctrl Pts',(0.366570558206358,0.602530288477345,
-1.4065796414));
#67539=CARTESIAN_POINT('Ctrl Pts',(0.034451567471494,0.704435811252572,
-1.39073752797176));
#67540=CARTESIAN_POINT('Ctrl Pts',(-0.306026375229727,0.63542472436951,
-1.37489541454353));
#67541=CARTESIAN_POINT('Ctrl Pts',(-0.57225342141949,0.412241124040289,
-1.35905330111529));
#67542=CARTESIAN_POINT('Ctrl Pts',(-0.667973682251133,0.169370387447164,
-1.34714883680712));
#67543=CARTESIAN_POINT('Ctrl Pts',(-0.676720185312876,0.0285699804139074,
-1.34052507697502));
#67544=CARTESIAN_POINT('Ctrl Pts',(-0.676691774264851,1.73213003940645E-5,
-1.339182021619));
#67545=CARTESIAN_POINT('Origin',(0.,0.,-3.278617978381));
#67546=CARTESIAN_POINT('',(-0.676663433474933,1.38299030018566E-5,-1.778617978381));
#67547=CARTESIAN_POINT('',(-0.676757588646615,6.12124814511891E-7,-1.739182021619));
#67548=CARTESIAN_POINT('',(-0.6767,-6.21087748740391E-14,-3.278617978381));
#67549=CARTESIAN_POINT('Ctrl Pts',(-0.676663433474933,1.38299030018468E-5,
-1.778617978381));
#67550=CARTESIAN_POINT('Ctrl Pts',(-0.67660888674756,-0.0733412266291114,
-1.77516792997636));
#67551=CARTESIAN_POINT('Ctrl Pts',(-0.646522617464707,-0.259018482991803,
-1.76643717709563));
#67552=CARTESIAN_POINT('Ctrl Pts',(-0.479681756700353,-0.517032047602386,
-1.75242571973882));
#67553=CARTESIAN_POINT('Ctrl Pts',(-0.174657691759948,-0.683309166240393,
-1.73658360631059));
#67554=CARTESIAN_POINT('Ctrl Pts',(0.172743407467333,-0.683795613568578,
-1.72074149288235));
#67555=CARTESIAN_POINT('Ctrl Pts',(0.478231933435968,-0.518373363321409,
-1.70489937945412));
#67556=CARTESIAN_POINT('Ctrl Pts',(0.667687487503493,-0.227178663149353,
-1.68905726602588));
#67557=CARTESIAN_POINT('Ctrl Pts',(0.695142643731443,0.119136186044015,
-1.67321515259765));
#67558=CARTESIAN_POINT('Ctrl Pts',(0.553935982945549,0.436545132554703,
-1.65737303916941));
#67559=CARTESIAN_POINT('Ctrl Pts',(0.278328346711741,0.648035537124133,
-1.64153092574118));
#67560=CARTESIAN_POINT('Ctrl Pts',(-0.0648098389800511,0.702293678406998,
-1.62568881231294));
#67561=CARTESIAN_POINT('Ctrl Pts',(-0.392223273354511,0.58615495374357,
-1.60984669888471));
#67562=CARTESIAN_POINT('Ctrl Pts',(-0.622245998352018,0.330274163232033,
-1.59415642090739));
#67563=CARTESIAN_POINT('Ctrl Pts',(-0.676725921543111,0.109003725444774,
-1.58374684740616));
#67564=CARTESIAN_POINT('Ctrl Pts',(-0.676756207239105,-3.37313647901958E-6,
-1.578617978381));
#67565=CARTESIAN_POINT('Ctrl Pts',(-0.676757566361161,6.11887936561055E-7,
-1.739182021619));
#67566=CARTESIAN_POINT('Ctrl Pts',(-0.676751570191694,-0.11165194125938,
-1.73392865106757));
#67567=CARTESIAN_POINT('Ctrl Pts',(-0.620176730411514,-0.335543843334032,
-1.72339457604006));
#67568=CARTESIAN_POINT('Ctrl Pts',(-0.385318490507109,-0.590716838721934,
-1.70757979653647));
#67569=CARTESIAN_POINT('Ctrl Pts',(-0.0565648575352245,-0.70300578914283,
-1.69173768310824));
#67570=CARTESIAN_POINT('Ctrl Pts',(0.285913054528226,-0.644725094847914,
-1.67589556968));
#67571=CARTESIAN_POINT('Ctrl Pts',(0.559020146487969,-0.430015346815531,
-1.66005345625177));
#67572=CARTESIAN_POINT('Ctrl Pts',(0.696492697099633,-0.110971372719233,
-1.64421134282353));
#67573=CARTESIAN_POINT('Ctrl Pts',(0.664975868496808,0.234997482950838,
-1.6283692293953));
#67574=CARTESIAN_POINT('Ctrl Pts',(0.472116559667202,0.523949116579385,
-1.61252711596706));
#67575=CARTESIAN_POINT('Ctrl Pts',(0.164708046420555,0.685775460424648,
-1.59668500253882));
#67576=CARTESIAN_POINT('Ctrl Pts',(-0.182663427862365,0.681212738282163,
-1.58084288911059));
#67577=CARTESIAN_POINT('Ctrl Pts',(-0.4857154435089,0.51136799920729,-1.56500077568235));
#67578=CARTESIAN_POINT('Ctrl Pts',(-0.648061864522484,0.253724400305278,
-1.55111381985182));
#67579=CARTESIAN_POINT('Ctrl Pts',(-0.676611918272213,0.07069740943459,
-1.54250756849737));
#67580=CARTESIAN_POINT('Ctrl Pts',(-0.676657745381425,-1.21934319497544E-5,
-1.539182021619));
#67581=CARTESIAN_POINT('Origin',(0.,0.,-3.278617978381));
#67582=CARTESIAN_POINT('',(-0.67668383139274,-1.69222484240121E-5,-1.978617978381));
#67583=CARTESIAN_POINT('',(-0.676655502517796,1.13969305124695E-5,-1.939182021619));
#67584=CARTESIAN_POINT('',(-0.6767,-6.21087748740391E-14,-3.278617978381));
#67585=CARTESIAN_POINT('Ctrl Pts',(-0.67668383139274,-1.69222484240131E-5,
-1.978617978381));
#67586=CARTESIAN_POINT('Ctrl Pts',(-0.676713552715602,-0.0312174719885095,
-1.97715042149871));
#67587=CARTESIAN_POINT('Ctrl Pts',(-0.66697116919625,-0.174668430854932,
-1.97040216014034));
#67588=CARTESIAN_POINT('Ctrl Pts',(-0.567376904718818,-0.418927408927545,
-1.95837319430588));
#67589=CARTESIAN_POINT('Ctrl Pts',(-0.298549410801028,-0.638971811013141,
-1.94253108087765));
#67590=CARTESIAN_POINT('Ctrl Pts',(0.0427148506610781,-0.703983073299391,
-1.92668896744941));
#67591=CARTESIAN_POINT('Ctrl Pts',(0.373615247395648,-0.598187573318388,
-1.91084685402117));
#67592=CARTESIAN_POINT('Ctrl Pts',(0.613865722048657,-0.347254375426338,
-1.89500474059294));
#67593=CARTESIAN_POINT('Ctrl Pts',(0.705174524058082,-0.0120671694489478,
-1.87916262716471));
#67594=CARTESIAN_POINT('Ctrl Pts',(0.625387483204131,0.326047882696172,
-1.86332051373647));
#67595=CARTESIAN_POINT('Ctrl Pts',(0.393863255448903,0.585054238482422,
-1.84747840030823));
#67596=CARTESIAN_POINT('Ctrl Pts',(0.0667763501367175,0.702109425247569,
-1.83163628688));
#67597=CARTESIAN_POINT('Ctrl Pts',(-0.276512439276773,0.648812451240159,
-1.81579417345177));
#67598=CARTESIAN_POINT('Ctrl Pts',(-0.552711271174482,0.438094711992443,
-1.79995206002353));
#67599=CARTESIAN_POINT('Ctrl Pts',(-0.663861249737369,0.190120444840065,
-1.78755999499994));
#67600=CARTESIAN_POINT('Ctrl Pts',(-0.676692376923236,0.0389373068692174,
-1.78044863445243));
#67601=CARTESIAN_POINT('Ctrl Pts',(-0.676663433474933,1.38299030018468E-5,
-1.778617978381));
#67602=CARTESIAN_POINT('Ctrl Pts',(-0.676655502517796,1.13969305124799E-5,
-1.939182021619));
#67603=CARTESIAN_POINT('Ctrl Pts',(-0.67661355821236,-0.0695364884621566,
-1.93591114258992));
#67604=CARTESIAN_POINT('Ctrl Pts',(-0.648726662967375,-0.251399550700432,
-1.92735955908476));
#67605=CARTESIAN_POINT('Ctrl Pts',(-0.488343718173467,-0.50885865974436,
-1.91352727110353));
#67606=CARTESIAN_POINT('Ctrl Pts',(-0.186170816147377,-0.680262559524874,
-1.8976851576753));
#67607=CARTESIAN_POINT('Ctrl Pts',(0.161172538892235,-0.686614983366474,
-1.88184304424706));
#67608=CARTESIAN_POINT('Ctrl Pts',(0.469410749818722,-0.526374648545063,
-1.86600093081882));
#67609=CARTESIAN_POINT('Ctrl Pts',(0.663756264470278,-0.238420519361853,
-1.85015881739059));
#67610=CARTESIAN_POINT('Ctrl Pts',(0.697055210292531,0.107381360022812,
-1.83431670396235));
#67611=CARTESIAN_POINT('Ctrl Pts',(0.561228294844321,0.427129399295399,
-1.81847459053412));
#67612=CARTESIAN_POINT('Ctrl Pts',(0.289231077053685,0.643243427282921,
-1.80263247710588));
#67613=CARTESIAN_POINT('Ctrl Pts',(-0.0529420095786137,0.703287897164517,
-1.78679036367765));
#67614=CARTESIAN_POINT('Ctrl Pts',(-0.382269825369864,0.592694274721806,
-1.77094825024941));
#67615=CARTESIAN_POINT('Ctrl Pts',(-0.618847866826519,0.338295788328172,
-1.75510613682118));
#67616=CARTESIAN_POINT('Ctrl Pts',(-0.676615359036302,0.113395975047391,
-1.74451739394437));
#67617=CARTESIAN_POINT('Ctrl Pts',(-0.676757597559959,0.000581553674673004,
-1.73920935554364));
#67618=CARTESIAN_POINT('Ctrl Pts',(-0.676757566361161,6.11887936561055E-7,
-1.739182021619));
#67619=CARTESIAN_POINT('Origin',(0.,0.,-3.278617978381));
#67620=CARTESIAN_POINT('',(-0.676743554268804,1.05936162663817E-5,-2.178617978381));
#67621=CARTESIAN_POINT('',(-0.676695356965443,-1.73809590335028E-5,-2.139182021619));
#67622=CARTESIAN_POINT('',(-0.6767,-6.21087748740391E-14,-3.278617978381));
#67623=CARTESIAN_POINT('Ctrl Pts',(-0.676743554268804,1.05936162663918E-5,
-2.178617978381));
#67624=CARTESIAN_POINT('Ctrl Pts',(-0.676667476509358,-0.1012848297298,
-2.17385220854498));
#67625=CARTESIAN_POINT('Ctrl Pts',(-0.628064490957334,-0.314891053553278,
-2.16380573423288));
#67626=CARTESIAN_POINT('Ctrl Pts',(-0.412048695144598,-0.572391997488336,
-2.14847855544471));
#67627=CARTESIAN_POINT('Ctrl Pts',(-0.0888006000396183,-0.699665047999155,
-2.13263644201647));
#67628=CARTESIAN_POINT('Ctrl Pts',(0.255993102559969,-0.657179014729453,
-2.11679432858824));
#67629=CARTESIAN_POINT('Ctrl Pts',(0.538675435341973,-0.455242244654634,
-2.10095221516));
#67630=CARTESIAN_POINT('Ctrl Pts',(0.690659445233286,-0.142850469614568,
-2.08511010173177));
#67631=CARTESIAN_POINT('Ctrl Pts',(0.675069392417806,0.204200982807891,
-2.06926798830353));
#67632=CARTESIAN_POINT('Ctrl Pts',(0.495687876997698,0.501707339548235,
-2.0534258748753));
#67633=CARTESIAN_POINT('Ctrl Pts',(0.196038070227499,0.67748490830463,-2.03758376144706));
#67634=CARTESIAN_POINT('Ctrl Pts',(-0.151176272291756,0.688884940069836,
-2.02174164801882));
#67635=CARTESIAN_POINT('Ctrl Pts',(-0.461710855621964,0.533141455675591,
-2.00589953459059));
#67636=CARTESIAN_POINT('Ctrl Pts',(-0.641831692782511,0.274452916762815,
-1.99152497804465));
#67637=CARTESIAN_POINT('Ctrl Pts',(-0.676606606589992,0.0810513501991045,
-1.98243112597479));
#67638=CARTESIAN_POINT('Ctrl Pts',(-0.67668383139274,-1.69222484240131E-5,
-1.978617978381));
#67639=CARTESIAN_POINT('Ctrl Pts',(-0.676695356965443,-1.73809590334646E-5,
-2.139182021619));
#67640=CARTESIAN_POINT('Ctrl Pts',(-0.676722971761624,-0.0274074129671462,
-2.13789363411227));
#67641=CARTESIAN_POINT('Ctrl Pts',(-0.668403647596514,-0.167044102559928,
-2.13132454212947));
#67642=CARTESIAN_POINT('Ctrl Pts',(-0.574369815989129,-0.409287230630185,
-2.11947474567059));
#67643=CARTESIAN_POINT('Ctrl Pts',(-0.309296212482741,-0.633839550375444,
-2.10363263224235));
#67644=CARTESIAN_POINT('Ctrl Pts',(0.0308216451249593,-0.704603965975287,
-2.08779051881412));
#67645=CARTESIAN_POINT('Ctrl Pts',(0.363461275469507,-0.60441097269192,
-2.07194840538588));
#67646=CARTESIAN_POINT('Ctrl Pts',(0.607914632553942,-0.357570303860817,
-2.05610629195764));
#67647=CARTESIAN_POINT('Ctrl Pts',(0.704870224337332,-0.0239726827650286,
-2.04026417852942));
#67648=CARTESIAN_POINT('Ctrl Pts',(0.630803805217274,0.315441408188147,
-2.02442206510117));
#67649=CARTESIAN_POINT('Ctrl Pts',(0.403686041993089,0.578320241887024,
-2.00857995167294));
#67650=CARTESIAN_POINT('Ctrl Pts',(0.0786223075935471,0.700881769933403,
-1.9927378382447));
#67651=CARTESIAN_POINT('Ctrl Pts',(-0.265517484613883,0.653389002081171,
-1.97689572481647));
#67652=CARTESIAN_POINT('Ctrl Pts',(-0.545235014990942,0.44736506468894,
-1.96105361138823));
#67653=CARTESIAN_POINT('Ctrl Pts',(-0.662223680273716,0.197745313637455,
-1.94848237698908));
#67654=CARTESIAN_POINT('Ctrl Pts',(-0.676681275630061,0.0427458143775428,
-1.941191847066));
#67655=CARTESIAN_POINT('Ctrl Pts',(-0.676655502517796,1.13969305124799E-5,
-1.939182021619));
#67656=CARTESIAN_POINT('Origin',(0.,0.,-3.278617978381));
#67657=CARTESIAN_POINT('',(-0.676643329184379,2.79728545575858E-6,-2.378617978381));
#67658=CARTESIAN_POINT('',(-0.67673389899023,1.33698385852213E-5,-2.339182021619));
#67659=CARTESIAN_POINT('',(-0.6767,-6.21087748740391E-14,-3.278617978381));
#67660=CARTESIAN_POINT('Ctrl Pts',(-0.676643329184379,2.7972854557759E-6,
-2.378617978381));
#67661=CARTESIAN_POINT('Ctrl Pts',(-0.67663476616155,-0.0591804042446534,
-2.37583470006734));
#67662=CARTESIAN_POINT('Ctrl Pts',(-0.654360090959969,-0.230658017222057,
-2.36777071727759));
#67663=CARTESIAN_POINT('Ctrl Pts',(-0.511204661425697,-0.485887353298784,
-2.35442603001177));
#67664=CARTESIAN_POINT('Ctrl Pts',(-0.217224922760744,-0.6709918471119,
-2.33858391658353));
#67665=CARTESIAN_POINT('Ctrl Pts',(0.129459898096913,-0.693294209368428,
-2.32274180315529));
#67666=CARTESIAN_POINT('Ctrl Pts',(0.4447339835604,-0.54738323853179,-2.30689968972706));
#67667=CARTESIAN_POINT('Ctrl Pts',(0.652102673733417,-0.268661178566577,
-2.29105757629882));
#67668=CARTESIAN_POINT('Ctrl Pts',(0.701252295024287,0.0752458947865185,
-2.27521546287059));
#67669=CARTESIAN_POINT('Ctrl Pts',(0.580257720256285,0.400896126249721,
-2.25937334944235));
#67670=CARTESIAN_POINT('Ctrl Pts',(0.318475751250181,0.629277301215201,
-2.24353123601412));
#67671=CARTESIAN_POINT('Ctrl Pts',(-0.0205776948622204,0.70497750633138,
-2.22768912258588));
#67672=CARTESIAN_POINT('Ctrl Pts',(-0.354638393893549,0.609629670813075,
-2.21184700915765));
#67673=CARTESIAN_POINT('Ctrl Pts',(-0.602653507265104,0.366367951846396,
-2.19600489572941));
#67674=CARTESIAN_POINT('Ctrl Pts',(-0.673824797868241,0.134136097894605,
-2.1849285521372));
#67675=CARTESIAN_POINT('Ctrl Pts',(-0.676751774362309,0.0109554197734116,
-2.17913291302106));
#67676=CARTESIAN_POINT('Ctrl Pts',(-0.676743554268804,1.05936162663918E-5,
-2.178617978381));
#67677=CARTESIAN_POINT('Ctrl Pts',(-0.67673389899023,1.33698385852126E-5,
-2.339182021619));
#67678=CARTESIAN_POINT('Ctrl Pts',(-0.676646756100591,-0.0974778733276775,
-2.33459542115855));
#67679=CARTESIAN_POINT('Ctrl Pts',(-0.630818080222992,-0.307293272594146,
-2.32472811622202));
#67680=CARTESIAN_POINT('Ctrl Pts',(-0.42165508048436,-0.565352735712883,
-2.30958010680941));
#67681=CARTESIAN_POINT('Ctrl Pts',(-0.100602142852268,-0.698065850425191,
-2.29373799338118));
#67682=CARTESIAN_POINT('Ctrl Pts',(0.244859799696957,-0.661407893185951,
-2.27789587995294));
#67683=CARTESIAN_POINT('Ctrl Pts',(0.530911635409909,-0.46427315027114,
-2.26205376652471));
#67684=CARTESIAN_POINT('Ctrl Pts',(0.688148871832329,-0.154492242110101,
-2.24621165309647));
#67685=CARTESIAN_POINT('Ctrl Pts',(0.678421183651292,0.192772975931516,
-2.23036953966824));
#67686=CARTESIAN_POINT('Ctrl Pts',(0.50408879085726,0.493265865034647,-2.21452742624));
#67687=CARTESIAN_POINT('Ctrl Pts',(0.207449800749737,0.674078113311214,
-2.19868531281176));
#67688=CARTESIAN_POINT('Ctrl Pts',(-0.13952254273371,0.691339412116387,
-2.18284319938353));
#67689=CARTESIAN_POINT('Ctrl Pts',(-0.45264266065732,0.540861668478527,
-2.1670010859553));
#67690=CARTESIAN_POINT('Ctrl Pts',(-0.639405118876778,0.282065431530378,
-2.15244736003378));
#67691=CARTESIAN_POINT('Ctrl Pts',(-0.676609787197944,0.0848559114366436,
-2.14317433858835));
#67692=CARTESIAN_POINT('Ctrl Pts',(-0.676695356965443,-1.73809590334646E-5,
-2.139182021619));
#67693=CARTESIAN_POINT('Origin',(0.,0.,-3.278617978381));
#67694=CARTESIAN_POINT('',(-0.676727467248305,-1.47039215481353E-5,-2.57861797838101));
#67695=CARTESIAN_POINT('',(-0.676642691248942,-7.12134560654221E-7,-2.539182021619));
#67696=CARTESIAN_POINT('',(-0.6767,-6.21087748740391E-14,-3.278617978381));
#67697=CARTESIAN_POINT('Ctrl Pts',(-0.676727467248305,-1.47039215481135E-5,
-2.57861797838101));
#67698=CARTESIAN_POINT('Ctrl Pts',(-0.676743689334983,-0.0170364276983481,
-2.57781719158969));
#67699=CARTESIAN_POINT('Ctrl Pts',(-0.671964491487141,-0.14629703446376,
-2.5717357003223));
#67700=CARTESIAN_POINT('Ctrl Pts',(-0.592565713804986,-0.382469084713778,
-2.56037350457882));
#67701=CARTESIAN_POINT('Ctrl Pts',(-0.338087697064974,-0.618961578023624,
-2.54453139115059));
#67702=CARTESIAN_POINT('Ctrl Pts',(-0.00157977493823928,-0.705275995805936,
-2.52868927772235));
#67703=CARTESIAN_POINT('Ctrl Pts',(0.335311446522369,-0.62046995075891,
-2.51284716429412));
#67704=CARTESIAN_POINT('Ctrl Pts',(0.590846361696255,-0.385119855146208,
-2.49700505086588));
#67705=CARTESIAN_POINT('Ctrl Pts',(0.703024770348556,-0.0563284851169273,
-2.48116293743765));
#67706=CARTESIAN_POINT('Ctrl Pts',(0.644628928892509,0.286129813186614,
-2.46532082400941));
#67707=CARTESIAN_POINT('Ctrl Pts',(0.429827366355921,0.559164699431498,
-2.44947871058118));
#67708=CARTESIAN_POINT('Ctrl Pts',(0.110737187280514,0.696529971582292,
-2.43363659715294));
#67709=CARTESIAN_POINT('Ctrl Pts',(-0.235221053172144,0.664896820644794,
-2.41779448372471));
#67710=CARTESIAN_POINT('Ctrl Pts',(-0.524107826947175,0.471940368788045,
-2.40195237029647));
#67711=CARTESIAN_POINT('Ctrl Pts',(-0.657417924147744,0.218495181204277,
-2.3888935351819));
#67712=CARTESIAN_POINT('Ctrl Pts',(-0.676651012755633,0.053107682682907,
-2.38111540454342));
#67713=CARTESIAN_POINT('Ctrl Pts',(-0.676643329184379,2.7972854557759E-6,
-2.378617978381));
#67714=CARTESIAN_POINT('Ctrl Pts',(-0.676642691248942,-7.12134560688915E-7,
-2.539182021619));
#67715=CARTESIAN_POINT('Ctrl Pts',(-0.676644728573157,-0.0553742322995621,
-2.5365779126809));
#67716=CARTESIAN_POINT('Ctrl Pts',(-0.656297668877348,-0.22303466957631,
-2.52869309926673));
#67717=CARTESIAN_POINT('Ctrl Pts',(-0.519336234411588,-0.477186125430353,
-2.51552758137647));
#67718=CARTESIAN_POINT('Ctrl Pts',(-0.228523993923267,-0.667228226979231,
-2.49968546794824));
#67719=CARTESIAN_POINT('Ctrl Pts',(0.117734811948404,-0.69538136064443,
-2.48384335452));
#67720=CARTESIAN_POINT('Ctrl Pts',(0.435427729238652,-0.554814757632145,
-2.46800124109176));
#67721=CARTESIAN_POINT('Ctrl Pts',(0.647473219121237,-0.279633962881997,
-2.45215912766353));
#67722=CARTESIAN_POINT('Ctrl Pts',(0.702422880414448,0.0633941617704607,
-2.43631701423529));
#67723=CARTESIAN_POINT('Ctrl Pts',(0.586944327597745,0.391041019558242,
-2.42047490080706));
#67724=CARTESIAN_POINT('Ctrl Pts',(0.329056015185207,0.623809956274138,
-2.40463278737882));
#67725=CARTESIAN_POINT('Ctrl Pts',(-0.0086708539911011,0.705224459989427,
-2.38879067395059));
#67726=CARTESIAN_POINT('Ctrl Pts',(-0.344293921879448,0.615531004932474,
-2.37294856052235));
#67727=CARTESIAN_POINT('Ctrl Pts',(-0.5963812737897,0.376491831185336,-2.35710644709412));
#67728=CARTESIAN_POINT('Ctrl Pts',(-0.672678295201022,0.141758276520581,
-2.34585093412633));
#67729=CARTESIAN_POINT('Ctrl Pts',(-0.676747086585303,0.0147670123138463,
-2.33987612563463));
#67730=CARTESIAN_POINT('Ctrl Pts',(-0.67673389899023,1.33698385852126E-5,
-2.339182021619));
#67731=CARTESIAN_POINT('Origin',(0.,0.,-3.278617978381));
#67732=CARTESIAN_POINT('',(-0.676702457484846,1.74000875470074E-5,-2.778617978381));
#67733=CARTESIAN_POINT('',(-0.676738003850817,-1.23232206216684E-5,-2.739182021619));
#67734=CARTESIAN_POINT('',(-0.6767,-6.21087748740391E-14,-3.278617978381));
#67735=CARTESIAN_POINT('Ctrl Pts',(-0.676702457484846,1.74000875470086E-5,
-2.778617978381));
#67736=CARTESIAN_POINT('Ctrl Pts',(-0.676613263759165,-0.0871212590025935,
-2.77451897863596));
#67737=CARTESIAN_POINT('Ctrl Pts',(-0.637924808175174,-0.286597009727134,
-2.76513927441484));
#67738=CARTESIAN_POINT('Ctrl Pts',(-0.447181721367947,-0.545385311748889,
-2.75047886571765));
#67739=CARTESIAN_POINT('Ctrl Pts',(-0.132564454783822,-0.692707336942753,
-2.73463675228941));
#67740=CARTESIAN_POINT('Ctrl Pts',(0.214216796165651,-0.67195822661804,
-2.71879463886118));
#67741=CARTESIAN_POINT('Ctrl Pts',(0.509022827335671,-0.488172612202699,
-2.70295252543294));
#67742=CARTESIAN_POINT('Ctrl Pts',(0.680325118730706,-0.185942077621786,
-2.68711041200471));
#67743=CARTESIAN_POINT('Ctrl Pts',(0.686560756397345,0.161403385589515,
-2.67126829857647));
#67744=CARTESIAN_POINT('Ctrl Pts',(0.526216791985425,0.469587707696419,
-2.65542618514823));
#67745=CARTESIAN_POINT('Ctrl Pts',(0.238197334034658,0.663836391711814,
-2.63958407172001));
#67746=CARTESIAN_POINT('Ctrl Pts',(-0.107615722986078,0.697019069108502,
-2.62374195829176));
#67747=CARTESIAN_POINT('Ctrl Pts',(-0.427318076565427,0.561084652399629,
-2.60789984486353));
#67748=CARTESIAN_POINT('Ctrl Pts',(-0.632421136632355,0.302767367517842,
-2.59285851822661));
#67749=CARTESIAN_POINT('Ctrl Pts',(-0.67663671448642,0.0952115438137001,
-2.58309789606577));
#67750=CARTESIAN_POINT('Ctrl Pts',(-0.676727467248305,-1.47039215481135E-5,
-2.57861797838101));
#67751=CARTESIAN_POINT('Ctrl Pts',(-0.676738003850817,-1.23232206217291E-5,
-2.739182021619));
#67752=CARTESIAN_POINT('Ctrl Pts',(-0.676749139750634,-0.0132249827090495,
-2.73856040420325));
#67753=CARTESIAN_POINT('Ctrl Pts',(-0.673150018663119,-0.138674493910342,
-2.73265808231143));
#67754=CARTESIAN_POINT('Ctrl Pts',(-0.598939416511963,-0.372408780057021,
-2.72147505594353));
#67755=CARTESIAN_POINT('Ctrl Pts',(-0.348490978460388,-0.613164545241514,
-2.7056329425153));
#67756=CARTESIAN_POINT('Ctrl Pts',(-0.0134884969402019,-0.705148767075711,
-2.68979082908706));
#67757=CARTESIAN_POINT('Ctrl Pts',(0.324786686361382,-0.626043393699459,
-2.67394871565883));
#67758=CARTESIAN_POINT('Ctrl Pts',(0.584259176083316,-0.395041691351842,
-2.65810660223059));
#67759=CARTESIAN_POINT('Ctrl Pts',(0.701973402101012,-0.068191388181339,
-2.64226448880235));
#67760=CARTESIAN_POINT('Ctrl Pts',(0.649368470484853,0.275204128232534,
-2.62642237537412));
#67761=CARTESIAN_POINT('Ctrl Pts',(0.439207867209178,0.551827121547341,
-2.61058026194588));
#67762=CARTESIAN_POINT('Ctrl Pts',(0.122482665136422,0.69456081044579,-2.59473814851765));
#67763=CARTESIAN_POINT('Ctrl Pts',(-0.223960392743318,0.668773852033162,
-2.57889603508941));
#67764=CARTESIAN_POINT('Ctrl Pts',(-0.516064147577321,0.480722912143853,
-2.56305392166118));
#67765=CARTESIAN_POINT('Ctrl Pts',(-0.65552228228443,0.226118938747654,
-2.54981591717104));
#67766=CARTESIAN_POINT('Ctrl Pts',(-0.676640597214846,0.0569141560676507,
-2.54185861715698));
#67767=CARTESIAN_POINT('Ctrl Pts',(-0.676642691248942,-7.12134560688915E-7,
-2.539182021619));
#67768=CARTESIAN_POINT('Ctrl Pts',(-0.291609820351005,0.201568937301636,
1.));
#67769=CARTESIAN_POINT('Ctrl Pts',(-0.291609820351005,0.201568937301636,
0.96));
#67770=CARTESIAN_POINT('Ctrl Pts',(-0.32673942707479,0.201568937301636,
1.));
#67771=CARTESIAN_POINT('Ctrl Pts',(-0.32673942707479,0.201568937301636,
0.96));
#67772=CARTESIAN_POINT('Ctrl Pts',(-0.349931773170829,0.179058706760406,
1.));
#67773=CARTESIAN_POINT('Ctrl Pts',(-0.349931773170829,0.179058706760406,
0.96));
#67774=CARTESIAN_POINT('',(-0.291609820351005,0.201568937301636,1.));
#67775=CARTESIAN_POINT('',(-0.349931773170829,0.179058706760406,1.));
#67776=CARTESIAN_POINT('Ctrl Pts',(-0.291609820351005,0.201568937301636,
1.));
#67777=CARTESIAN_POINT('Ctrl Pts',(-0.32673942707479,0.201568937301636,
1.));
#67778=CARTESIAN_POINT('Ctrl Pts',(-0.349931773170829,0.179058706760406,
1.));
#67779=CARTESIAN_POINT('',(-0.291609820351005,0.201568937301636,0.96));
#67780=CARTESIAN_POINT('',(-0.291609820351005,0.201568937301636,1.));
#67781=CARTESIAN_POINT('',(-0.349931773170829,0.179058706760406,0.96));
#67782=CARTESIAN_POINT('Ctrl Pts',(-0.291609820351005,0.201568937301636,
0.96));
#67783=CARTESIAN_POINT('Ctrl Pts',(-0.32673942707479,0.201568937301636,
0.96));
#67784=CARTESIAN_POINT('Ctrl Pts',(-0.349931773170829,0.179058706760406,
0.96));
#67785=CARTESIAN_POINT('',(-0.349931773170829,0.179058706760406,1.));
#67786=CARTESIAN_POINT('Ctrl Pts',(-0.23345836661756,0.178547120094299,
1.));
#67787=CARTESIAN_POINT('Ctrl Pts',(-0.23345836661756,0.178547120094299,
0.96));
#67788=CARTESIAN_POINT('Ctrl Pts',(-0.256821271404624,0.201568937301636,
1.));
#67789=CARTESIAN_POINT('Ctrl Pts',(-0.256821271404624,0.201568937301636,
0.96));
#67790=CARTESIAN_POINT('Ctrl Pts',(-0.291609820351005,0.201568937301636,
1.));
#67791=CARTESIAN_POINT('Ctrl Pts',(-0.291609820351005,0.201568937301636,
0.96));
#67792=CARTESIAN_POINT('',(-0.23345836661756,0.178547120094299,1.));
#67793=CARTESIAN_POINT('Ctrl Pts',(-0.23345836661756,0.178547120094299,
1.));
#67794=CARTESIAN_POINT('Ctrl Pts',(-0.256821271404624,0.201568937301636,
1.));
#67795=CARTESIAN_POINT('Ctrl Pts',(-0.291609820351005,0.201568937301636,
1.));
#67796=CARTESIAN_POINT('',(-0.23345836661756,0.178547120094299,0.96));
#67797=CARTESIAN_POINT('',(-0.23345836661756,0.178547120094299,1.));
#67798=CARTESIAN_POINT('Ctrl Pts',(-0.23345836661756,0.178547120094299,
0.96));
#67799=CARTESIAN_POINT('Ctrl Pts',(-0.256821271404624,0.201568937301636,
0.96));
#67800=CARTESIAN_POINT('Ctrl Pts',(-0.291609820351005,0.201568937301636,
0.96));
#67801=CARTESIAN_POINT('Ctrl Pts',(-0.210095491632819,0.121759927272797,
1.));
#67802=CARTESIAN_POINT('Ctrl Pts',(-0.210095491632819,0.121759927272797,
0.96));
#67803=CARTESIAN_POINT('Ctrl Pts',(-0.210095491632819,0.15552527308464,
1.));
#67804=CARTESIAN_POINT('Ctrl Pts',(-0.210095491632819,0.15552527308464,
0.96));
#67805=CARTESIAN_POINT('Ctrl Pts',(-0.23345836661756,0.178547120094299,
1.));
#67806=CARTESIAN_POINT('Ctrl Pts',(-0.23345836661756,0.178547120094299,
0.96));
#67807=CARTESIAN_POINT('',(-0.210095491632819,0.121759927272797,1.));
#67808=CARTESIAN_POINT('Ctrl Pts',(-0.210095491632819,0.121759927272797,
1.));
#67809=CARTESIAN_POINT('Ctrl Pts',(-0.210095491632819,0.15552527308464,
1.));
#67810=CARTESIAN_POINT('Ctrl Pts',(-0.23345836661756,0.178547120094299,
1.));
#67811=CARTESIAN_POINT('',(-0.210095491632819,0.121759927272797,0.96));
#67812=CARTESIAN_POINT('',(-0.210095491632819,0.121759927272797,1.));
#67813=CARTESIAN_POINT('Ctrl Pts',(-0.210095491632819,0.121759927272797,
0.96));
#67814=CARTESIAN_POINT('Ctrl Pts',(-0.210095491632819,0.15552527308464,
0.96));
#67815=CARTESIAN_POINT('Ctrl Pts',(-0.23345836661756,0.178547120094299,
0.96));
#67816=CARTESIAN_POINT('Ctrl Pts',(-0.232776251062751,0.0670191407203674,
1.));
#67817=CARTESIAN_POINT('Ctrl Pts',(-0.232776251062751,0.0670191407203674,
0.96));
#67818=CARTESIAN_POINT('Ctrl Pts',(-0.210095491632819,0.0893588423728943,
1.));
#67819=CARTESIAN_POINT('Ctrl Pts',(-0.210095491632819,0.0893588423728943,
0.96));
#67820=CARTESIAN_POINT('Ctrl Pts',(-0.210095491632819,0.121759927272797,
1.));
#67821=CARTESIAN_POINT('Ctrl Pts',(-0.210095491632819,0.121759927272797,
0.96));
#67822=CARTESIAN_POINT('',(-0.232776251062751,0.0670191407203674,1.));
#67823=CARTESIAN_POINT('Ctrl Pts',(-0.232776251062751,0.0670191407203674,
1.));
#67824=CARTESIAN_POINT('Ctrl Pts',(-0.210095491632819,0.0893588423728943,
1.));
#67825=CARTESIAN_POINT('Ctrl Pts',(-0.210095491632819,0.121759927272797,
1.));
#67826=CARTESIAN_POINT('',(-0.232776251062751,0.0670191407203674,0.96));
#67827=CARTESIAN_POINT('',(-0.232776251062751,0.0670191407203674,1.));
#67828=CARTESIAN_POINT('Ctrl Pts',(-0.232776251062751,0.0670191407203674,
0.96));
#67829=CARTESIAN_POINT('Ctrl Pts',(-0.210095491632819,0.0893588423728943,
0.96));
#67830=CARTESIAN_POINT('Ctrl Pts',(-0.210095491632819,0.121759927272797,
0.96));
#67831=CARTESIAN_POINT('Ctrl Pts',(-0.290927674993873,0.0446794390678406,
1.));
#67832=CARTESIAN_POINT('Ctrl Pts',(-0.290927674993873,0.0446794390678406,
0.96));
#67833=CARTESIAN_POINT('Ctrl Pts',(-0.255457010492682,0.0446794390678406,
1.));
#67834=CARTESIAN_POINT('Ctrl Pts',(-0.255457010492682,0.0446794390678406,
0.96));
#67835=CARTESIAN_POINT('Ctrl Pts',(-0.232776251062751,0.0670191407203674,
1.));
#67836=CARTESIAN_POINT('Ctrl Pts',(-0.232776251062751,0.0670191407203674,
0.96));
#67837=CARTESIAN_POINT('',(-0.290927674993873,0.0446794390678406,1.));
#67838=CARTESIAN_POINT('Ctrl Pts',(-0.290927674993873,0.0446794390678406,
1.));
#67839=CARTESIAN_POINT('Ctrl Pts',(-0.255457010492682,0.0446794390678406,
1.));
#67840=CARTESIAN_POINT('Ctrl Pts',(-0.232776251062751,0.0670191407203674,
1.));
#67841=CARTESIAN_POINT('',(-0.290927674993873,0.0446794390678406,0.96));
#67842=CARTESIAN_POINT('',(-0.290927674993873,0.0446794390678406,1.));
#67843=CARTESIAN_POINT('Ctrl Pts',(-0.290927674993873,0.0446794390678406,
0.96));
#67844=CARTESIAN_POINT('Ctrl Pts',(-0.255457010492682,0.0446794390678406,
0.96));
#67845=CARTESIAN_POINT('Ctrl Pts',(-0.232776251062751,0.0670191407203674,
0.96));
#67846=CARTESIAN_POINT('Ctrl Pts',(-0.350272860750556,0.0671896696090698,
1.));
#67847=CARTESIAN_POINT('Ctrl Pts',(-0.350272860750556,0.0671896696090698,
0.96));
#67848=CARTESIAN_POINT('Ctrl Pts',(-0.3274215426296,0.0446794390678406,
1.));
#67849=CARTESIAN_POINT('Ctrl Pts',(-0.3274215426296,0.0446794390678406,
0.96));
#67850=CARTESIAN_POINT('Ctrl Pts',(-0.290927674993873,0.0446794390678406,
1.));
#67851=CARTESIAN_POINT('Ctrl Pts',(-0.290927674993873,0.0446794390678406,
0.96));
#67852=CARTESIAN_POINT('',(-0.350272860750556,0.0671896696090698,1.));
#67853=CARTESIAN_POINT('Ctrl Pts',(-0.350272860750556,0.0671896696090698,
1.));
#67854=CARTESIAN_POINT('Ctrl Pts',(-0.3274215426296,0.0446794390678406,
1.));
#67855=CARTESIAN_POINT('Ctrl Pts',(-0.290927674993873,0.0446794390678406,
1.));
#67856=CARTESIAN_POINT('',(-0.350272860750556,0.0671896696090698,0.96));
#67857=CARTESIAN_POINT('',(-0.350272860750556,0.0671896696090698,1.));
#67858=CARTESIAN_POINT('Ctrl Pts',(-0.350272860750556,0.0671896696090698,
0.96));
#67859=CARTESIAN_POINT('Ctrl Pts',(-0.3274215426296,0.0446794390678406,
0.96));
#67860=CARTESIAN_POINT('Ctrl Pts',(-0.290927674993873,0.0446794390678406,
0.96));
#67861=CARTESIAN_POINT('Ctrl Pts',(-0.37312414906919,0.125170594453812,
1.));
#67862=CARTESIAN_POINT('Ctrl Pts',(-0.37312414906919,0.125170594453812,
0.96));
#67863=CARTESIAN_POINT('Ctrl Pts',(-0.37312414906919,0.0896999001502991,
1.));
#67864=CARTESIAN_POINT('Ctrl Pts',(-0.37312414906919,0.0896999001502991,
0.96));
#67865=CARTESIAN_POINT('Ctrl Pts',(-0.350272860750556,0.0671896696090698,
1.));
#67866=CARTESIAN_POINT('Ctrl Pts',(-0.350272860750556,0.0671896696090698,
0.96));
#67867=CARTESIAN_POINT('',(-0.37312414906919,0.125170594453812,1.));
#67868=CARTESIAN_POINT('Ctrl Pts',(-0.37312414906919,0.125170594453812,
1.));
#67869=CARTESIAN_POINT('Ctrl Pts',(-0.37312414906919,0.0896999001502991,
1.));
#67870=CARTESIAN_POINT('Ctrl Pts',(-0.350272860750556,0.0671896696090698,
1.));
#67871=CARTESIAN_POINT('',(-0.37312414906919,0.125170594453812,0.96));
#67872=CARTESIAN_POINT('',(-0.37312414906919,0.125170594453812,1.));
#67873=CARTESIAN_POINT('Ctrl Pts',(-0.37312414906919,0.125170594453812,
0.96));
#67874=CARTESIAN_POINT('Ctrl Pts',(-0.37312414906919,0.0896999001502991,
0.96));
#67875=CARTESIAN_POINT('Ctrl Pts',(-0.350272860750556,0.0671896696090698,
0.96));
#67876=CARTESIAN_POINT('Ctrl Pts',(-0.349931773170829,0.179058706760406,
1.));
#67877=CARTESIAN_POINT('Ctrl Pts',(-0.349931773170829,0.179058706760406,
0.96));
#67878=CARTESIAN_POINT('Ctrl Pts',(-0.37312414906919,0.156548476219177,
1.));
#67879=CARTESIAN_POINT('Ctrl Pts',(-0.37312414906919,0.156548476219177,
0.96));
#67880=CARTESIAN_POINT('Ctrl Pts',(-0.37312414906919,0.125170594453812,
1.));
#67881=CARTESIAN_POINT('Ctrl Pts',(-0.37312414906919,0.125170594453812,
0.96));
#67882=CARTESIAN_POINT('Ctrl Pts',(-0.349931773170829,0.179058706760406,
1.));
#67883=CARTESIAN_POINT('Ctrl Pts',(-0.37312414906919,0.156548476219177,
1.));
#67884=CARTESIAN_POINT('Ctrl Pts',(-0.37312414906919,0.125170594453812,
1.));
#67885=CARTESIAN_POINT('Ctrl Pts',(-0.349931773170829,0.179058706760406,
0.96));
#67886=CARTESIAN_POINT('Ctrl Pts',(-0.37312414906919,0.156548476219177,
0.96));
#67887=CARTESIAN_POINT('Ctrl Pts',(-0.37312414906919,0.125170594453812,
0.96));
#67888=CARTESIAN_POINT('Ctrl Pts',(-0.292633023485541,-0.00545700788497927,
1.));
#67889=CARTESIAN_POINT('Ctrl Pts',(-0.292633023485541,-0.00545700788497927,
0.96));
#67890=CARTESIAN_POINT('Ctrl Pts',(-0.335948136076331,-0.00545700788497927,
1.));
#67891=CARTESIAN_POINT('Ctrl Pts',(-0.335948136076331,-0.00545700788497927,
0.96));
#67892=CARTESIAN_POINT('Ctrl Pts',(-0.364426996931434,-0.0341063976287842,
1.));
#67893=CARTESIAN_POINT('Ctrl Pts',(-0.364426996931434,-0.0341063976287842,
0.96));
#67894=CARTESIAN_POINT('',(-0.292633023485541,-0.00545700788497927,1.));
#67895=CARTESIAN_POINT('',(-0.364426996931434,-0.0341063976287842,1.));
#67896=CARTESIAN_POINT('Ctrl Pts',(-0.292633023485541,-0.00545700788497927,
1.));
#67897=CARTESIAN_POINT('Ctrl Pts',(-0.335948136076331,-0.00545700788497927,
1.));
#67898=CARTESIAN_POINT('Ctrl Pts',(-0.364426996931434,-0.0341063976287842,
1.));
#67899=CARTESIAN_POINT('',(-0.292633023485541,-0.00545700788497927,0.96));
#67900=CARTESIAN_POINT('',(-0.292633023485541,-0.00545700788497927,1.));
#67901=CARTESIAN_POINT('',(-0.364426996931434,-0.0341063976287842,0.96));
#67902=CARTESIAN_POINT('Ctrl Pts',(-0.292633023485541,-0.00545700788497927,
0.96));
#67903=CARTESIAN_POINT('Ctrl Pts',(-0.335948136076331,-0.00545700788497927,
0.96));
#67904=CARTESIAN_POINT('Ctrl Pts',(-0.364426996931434,-0.0341063976287842,
0.96));
#67905=CARTESIAN_POINT('',(-0.364426996931434,-0.0341063976287842,1.));
#67906=CARTESIAN_POINT('Ctrl Pts',(-0.218792613968253,-0.034447455406189,
1.));
#67907=CARTESIAN_POINT('Ctrl Pts',(-0.218792613968253,-0.034447455406189,
0.96));
#67908=CARTESIAN_POINT('Ctrl Pts',(-0.248294677957892,-0.00545700788497927,
1.));
#67909=CARTESIAN_POINT('Ctrl Pts',(-0.248294677957892,-0.00545700788497927,
0.96));
#67910=CARTESIAN_POINT('Ctrl Pts',(-0.292633023485541,-0.00545700788497927,
1.));
#67911=CARTESIAN_POINT('Ctrl Pts',(-0.292633023485541,-0.00545700788497927,
0.96));
#67912=CARTESIAN_POINT('',(-0.218792613968253,-0.034447455406189,1.));
#67913=CARTESIAN_POINT('Ctrl Pts',(-0.218792613968253,-0.034447455406189,
1.));
#67914=CARTESIAN_POINT('Ctrl Pts',(-0.248294677957892,-0.00545700788497927,
1.));
#67915=CARTESIAN_POINT('Ctrl Pts',(-0.292633023485541,-0.00545700788497927,
1.));
#67916=CARTESIAN_POINT('',(-0.218792613968253,-0.034447455406189,0.96));
#67917=CARTESIAN_POINT('',(-0.218792613968253,-0.034447455406189,1.));
#67918=CARTESIAN_POINT('Ctrl Pts',(-0.218792613968253,-0.034447455406189,
0.96));
#67919=CARTESIAN_POINT('Ctrl Pts',(-0.248294677957892,-0.00545700788497927,
0.96));
#67920=CARTESIAN_POINT('Ctrl Pts',(-0.292633023485541,-0.00545700788497927,
0.96));
#67921=CARTESIAN_POINT('Ctrl Pts',(-0.189290579780936,-0.107776248455048,
1.));
#67922=CARTESIAN_POINT('Ctrl Pts',(-0.189290579780936,-0.107776248455048,
0.96));
#67923=CARTESIAN_POINT('Ctrl Pts',(-0.189290579780936,-0.0634379029273987,
1.));
#67924=CARTESIAN_POINT('Ctrl Pts',(-0.189290579780936,-0.0634379029273987,
0.96));
#67925=CARTESIAN_POINT('Ctrl Pts',(-0.218792613968253,-0.034447455406189,
1.));
#67926=CARTESIAN_POINT('Ctrl Pts',(-0.218792613968253,-0.034447455406189,
0.96));
#67927=CARTESIAN_POINT('',(-0.189290579780936,-0.107776248455048,1.));
#67928=CARTESIAN_POINT('Ctrl Pts',(-0.189290579780936,-0.107776248455048,
1.));
#67929=CARTESIAN_POINT('Ctrl Pts',(-0.189290579780936,-0.0634379029273987,
1.));
#67930=CARTESIAN_POINT('Ctrl Pts',(-0.218792613968253,-0.034447455406189,
1.));
#67931=CARTESIAN_POINT('',(-0.189290579780936,-0.107776248455048,0.96));
#67932=CARTESIAN_POINT('',(-0.189290579780936,-0.107776248455048,1.));
#67933=CARTESIAN_POINT('Ctrl Pts',(-0.189290579780936,-0.107776248455048,
0.96));
#67934=CARTESIAN_POINT('Ctrl Pts',(-0.189290579780936,-0.0634379029273987,
0.96));
#67935=CARTESIAN_POINT('Ctrl Pts',(-0.218792613968253,-0.034447455406189,
0.96));
#67936=CARTESIAN_POINT('Ctrl Pts',(-0.217939969524741,-0.179740750789642,
1.));
#67937=CARTESIAN_POINT('Ctrl Pts',(-0.217939969524741,-0.179740750789642,
0.96));
#67938=CARTESIAN_POINT('Ctrl Pts',(-0.189290579780936,-0.151432418823242,
1.));
#67939=CARTESIAN_POINT('Ctrl Pts',(-0.189290579780936,-0.151432418823242,
0.96));
#67940=CARTESIAN_POINT('Ctrl Pts',(-0.189290579780936,-0.107776248455048,
1.));
#67941=CARTESIAN_POINT('Ctrl Pts',(-0.189290579780936,-0.107776248455048,
0.96));
#67942=CARTESIAN_POINT('',(-0.217939969524741,-0.179740750789642,1.));
#67943=CARTESIAN_POINT('Ctrl Pts',(-0.217939969524741,-0.179740750789642,
1.));
#67944=CARTESIAN_POINT('Ctrl Pts',(-0.189290579780936,-0.151432418823242,
1.));
#67945=CARTESIAN_POINT('Ctrl Pts',(-0.189290579780936,-0.107776248455048,
1.));
#67946=CARTESIAN_POINT('',(-0.217939969524741,-0.179740750789642,0.96));
#67947=CARTESIAN_POINT('',(-0.217939969524741,-0.179740750789642,1.));
#67948=CARTESIAN_POINT('Ctrl Pts',(-0.217939969524741,-0.179740750789642,
0.96));
#67949=CARTESIAN_POINT('Ctrl Pts',(-0.189290579780936,-0.151432418823242,
0.96));
#67950=CARTESIAN_POINT('Ctrl Pts',(-0.189290579780936,-0.107776248455048,
0.96));
#67951=CARTESIAN_POINT('Ctrl Pts',(-0.290586617216468,-0.208049082756043,
1.));
#67952=CARTESIAN_POINT('Ctrl Pts',(-0.290586617216468,-0.208049082756043,
0.96));
#67953=CARTESIAN_POINT('Ctrl Pts',(-0.246589359268546,-0.208049082756043,
1.));
#67954=CARTESIAN_POINT('Ctrl Pts',(-0.246589359268546,-0.208049082756043,
0.96));
#67955=CARTESIAN_POINT('Ctrl Pts',(-0.217939969524741,-0.179740750789642,
1.));
#67956=CARTESIAN_POINT('Ctrl Pts',(-0.217939969524741,-0.179740750789642,
0.96));
#67957=CARTESIAN_POINT('',(-0.290586617216468,-0.208049082756043,1.));
#67958=CARTESIAN_POINT('Ctrl Pts',(-0.290586617216468,-0.208049082756043,
1.));
#67959=CARTESIAN_POINT('Ctrl Pts',(-0.246589359268546,-0.208049082756043,
1.));
#67960=CARTESIAN_POINT('Ctrl Pts',(-0.217939969524741,-0.179740750789642,
1.));
#67961=CARTESIAN_POINT('',(-0.290586617216468,-0.208049082756043,0.96));
#67962=CARTESIAN_POINT('',(-0.290586617216468,-0.208049082756043,1.));
#67963=CARTESIAN_POINT('Ctrl Pts',(-0.290586617216468,-0.208049082756043,
0.96));
#67964=CARTESIAN_POINT('Ctrl Pts',(-0.246589359268546,-0.208049082756043,
0.96));
#67965=CARTESIAN_POINT('Ctrl Pts',(-0.217939969524741,-0.179740750789642,
0.96));
#67966=CARTESIAN_POINT('Ctrl Pts',(-0.343451556190848,-0.194577062129974,
1.));
#67967=CARTESIAN_POINT('Ctrl Pts',(-0.343451556190848,-0.194577062129974,
0.96));
#67968=CARTESIAN_POINT('Ctrl Pts',(-0.318894949182868,-0.208049082756043,
1.));
#67969=CARTESIAN_POINT('Ctrl Pts',(-0.318894949182868,-0.208049082756043,
0.96));
#67970=CARTESIAN_POINT('Ctrl Pts',(-0.290586617216468,-0.208049082756043,
1.));
#67971=CARTESIAN_POINT('Ctrl Pts',(-0.290586617216468,-0.208049082756043,
0.96));
#67972=CARTESIAN_POINT('',(-0.343451556190848,-0.194577062129974,1.));
#67973=CARTESIAN_POINT('Ctrl Pts',(-0.343451556190848,-0.194577062129974,
1.));
#67974=CARTESIAN_POINT('Ctrl Pts',(-0.318894949182868,-0.208049082756043,
1.));
#67975=CARTESIAN_POINT('Ctrl Pts',(-0.290586617216468,-0.208049082756043,
1.));
#67976=CARTESIAN_POINT('',(-0.343451556190848,-0.194577062129974,0.96));
#67977=CARTESIAN_POINT('',(-0.343451556190848,-0.194577062129974,1.));
#67978=CARTESIAN_POINT('Ctrl Pts',(-0.343451556190848,-0.194577062129974,
0.96));
#67979=CARTESIAN_POINT('Ctrl Pts',(-0.318894949182868,-0.208049082756043,
0.96));
#67980=CARTESIAN_POINT('Ctrl Pts',(-0.290586617216468,-0.208049082756043,
0.96));
#67981=CARTESIAN_POINT('Ctrl Pts',(-0.380457010492682,-0.156548404693604,
1.));
#67982=CARTESIAN_POINT('Ctrl Pts',(-0.380457010492682,-0.156548404693604,
0.96));
#67983=CARTESIAN_POINT('Ctrl Pts',(-0.368008163198829,-0.181104981899261,
1.));
#67984=CARTESIAN_POINT('Ctrl Pts',(-0.368008163198829,-0.181104981899261,
0.96));
#67985=CARTESIAN_POINT('Ctrl Pts',(-0.343451556190848,-0.194577062129974,
1.));
#67986=CARTESIAN_POINT('Ctrl Pts',(-0.343451556190848,-0.194577062129974,
0.96));
#67987=CARTESIAN_POINT('',(-0.380457010492682,-0.156548404693604,1.));
#67988=CARTESIAN_POINT('Ctrl Pts',(-0.380457010492682,-0.156548404693604,
1.));
#67989=CARTESIAN_POINT('Ctrl Pts',(-0.368008163198829,-0.181104981899261,
1.));
#67990=CARTESIAN_POINT('Ctrl Pts',(-0.343451556190848,-0.194577062129974,
1.));
#67991=CARTESIAN_POINT('',(-0.380457010492682,-0.156548404693604,0.96));
#67992=CARTESIAN_POINT('',(-0.380457010492682,-0.156548404693604,1.));
#67993=CARTESIAN_POINT('Ctrl Pts',(-0.380457010492682,-0.156548404693604,
0.96));
#67994=CARTESIAN_POINT('Ctrl Pts',(-0.368008163198829,-0.181104981899261,
0.96));
#67995=CARTESIAN_POINT('Ctrl Pts',(-0.343451556190848,-0.194577062129974,
0.96));
#67996=CARTESIAN_POINT('Ctrl Pts',(-0.392905857786536,-0.105729842185974,
1.));
#67997=CARTESIAN_POINT('Ctrl Pts',(-0.392905857786536,-0.105729842185974,
0.96));
#67998=CARTESIAN_POINT('Ctrl Pts',(-0.392905857786536,-0.131991767883301,
1.));
#67999=CARTESIAN_POINT('Ctrl Pts',(-0.392905857786536,-0.131991767883301,
0.96));
#68000=CARTESIAN_POINT('Ctrl Pts',(-0.380457010492682,-0.156548404693604,
1.));
#68001=CARTESIAN_POINT('Ctrl Pts',(-0.380457010492682,-0.156548404693604,
0.96));
#68002=CARTESIAN_POINT('',(-0.392905857786536,-0.105729842185974,1.));
#68003=CARTESIAN_POINT('Ctrl Pts',(-0.392905857786536,-0.105729842185974,
1.));
#68004=CARTESIAN_POINT('Ctrl Pts',(-0.392905857786536,-0.131991767883301,
1.));
#68005=CARTESIAN_POINT('Ctrl Pts',(-0.380457010492682,-0.156548404693604,
1.));
#68006=CARTESIAN_POINT('',(-0.392905857786536,-0.105729842185974,0.96));
#68007=CARTESIAN_POINT('',(-0.392905857786536,-0.105729842185974,1.));
#68008=CARTESIAN_POINT('Ctrl Pts',(-0.392905857786536,-0.105729842185974,
0.96));
#68009=CARTESIAN_POINT('Ctrl Pts',(-0.392905857786536,-0.131991767883301,
0.96));
#68010=CARTESIAN_POINT('Ctrl Pts',(-0.380457010492682,-0.156548404693604,
0.96));
#68011=CARTESIAN_POINT('Ctrl Pts',(-0.364426996931434,-0.0341063976287842,
1.));
#68012=CARTESIAN_POINT('Ctrl Pts',(-0.364426996931434,-0.0341063976287842,
0.96));
#68013=CARTESIAN_POINT('Ctrl Pts',(-0.392905857786536,-0.0627557873725891,
1.));
#68014=CARTESIAN_POINT('Ctrl Pts',(-0.392905857786536,-0.0627557873725891,
0.96));
#68015=CARTESIAN_POINT('Ctrl Pts',(-0.392905857786536,-0.105729842185974,
1.));
#68016=CARTESIAN_POINT('Ctrl Pts',(-0.392905857786536,-0.105729842185974,
0.96));
#68017=CARTESIAN_POINT('Ctrl Pts',(-0.364426996931434,-0.0341063976287842,
1.));
#68018=CARTESIAN_POINT('Ctrl Pts',(-0.392905857786536,-0.0627557873725891,
1.));
#68019=CARTESIAN_POINT('Ctrl Pts',(-0.392905857786536,-0.105729842185974,
1.));
#68020=CARTESIAN_POINT('Ctrl Pts',(-0.364426996931434,-0.0341063976287842,
0.96));
#68021=CARTESIAN_POINT('Ctrl Pts',(-0.392905857786536,-0.0627557873725891,
0.96));
#68022=CARTESIAN_POINT('Ctrl Pts',(-0.392905857786536,-0.105729842185974,
0.96));
#68023=CARTESIAN_POINT('Ctrl Pts',(-0.410641190037131,-0.214699828624725,
1.));
#68024=CARTESIAN_POINT('Ctrl Pts',(-0.410641190037131,-0.214699828624725,
0.96));
#68025=CARTESIAN_POINT('Ctrl Pts',(-0.456002723798156,-0.170873069763184,
1.));
#68026=CARTESIAN_POINT('Ctrl Pts',(-0.456002723798156,-0.170873069763184,
0.96));
#68027=CARTESIAN_POINT('Ctrl Pts',(-0.456002723798156,-0.105388784408569,
1.));
#68028=CARTESIAN_POINT('Ctrl Pts',(-0.456002723798156,-0.105388784408569,
0.96));
#68029=CARTESIAN_POINT('',(-0.410641190037131,-0.214699828624725,1.));
#68030=CARTESIAN_POINT('',(-0.456002723798156,-0.105388784408569,1.));
#68031=CARTESIAN_POINT('Ctrl Pts',(-0.410641190037131,-0.214699828624725,
1.));
#68032=CARTESIAN_POINT('Ctrl Pts',(-0.456002723798156,-0.170873069763184,
1.));
#68033=CARTESIAN_POINT('Ctrl Pts',(-0.456002723798156,-0.105388784408569,
1.));
#68034=CARTESIAN_POINT('',(-0.410641190037131,-0.214699828624725,0.96));
#68035=CARTESIAN_POINT('',(-0.410641190037131,-0.214699828624725,1.));
#68036=CARTESIAN_POINT('',(-0.456002723798156,-0.105388784408569,0.96));
#68037=CARTESIAN_POINT('Ctrl Pts',(-0.410641190037131,-0.214699828624725,
0.96));
#68038=CARTESIAN_POINT('Ctrl Pts',(-0.456002723798156,-0.170873069763184,
0.96));
#68039=CARTESIAN_POINT('Ctrl Pts',(-0.456002723798156,-0.105388784408569,
0.96));
#68040=CARTESIAN_POINT('',(-0.456002723798156,-0.105388784408569,1.));
#68041=CARTESIAN_POINT('Ctrl Pts',(-0.291268732771277,-0.258526587486267,
1.));
#68042=CARTESIAN_POINT('Ctrl Pts',(-0.291268732771277,-0.258526587486267,
0.96));
#68043=CARTESIAN_POINT('Ctrl Pts',(-0.365279641374946,-0.258526587486267,
1.));
#68044=CARTESIAN_POINT('Ctrl Pts',(-0.365279641374946,-0.258526587486267,
0.96));
#68045=CARTESIAN_POINT('Ctrl Pts',(-0.410641190037131,-0.214699828624725,
1.));
#68046=CARTESIAN_POINT('Ctrl Pts',(-0.410641190037131,-0.214699828624725,
0.96));
#68047=CARTESIAN_POINT('',(-0.291268732771277,-0.258526587486267,1.));
#68048=CARTESIAN_POINT('Ctrl Pts',(-0.291268732771277,-0.258526587486267,
1.));
#68049=CARTESIAN_POINT('Ctrl Pts',(-0.365279641374946,-0.258526587486267,
1.));
#68050=CARTESIAN_POINT('Ctrl Pts',(-0.410641190037131,-0.214699828624725,
1.));
#68051=CARTESIAN_POINT('',(-0.291268732771277,-0.258526587486267,0.96));
#68052=CARTESIAN_POINT('',(-0.291268732771277,-0.258526587486267,1.));
#68053=CARTESIAN_POINT('Ctrl Pts',(-0.291268732771277,-0.258526587486267,
0.96));
#68054=CARTESIAN_POINT('Ctrl Pts',(-0.365279641374946,-0.258526587486267,
0.96));
#68055=CARTESIAN_POINT('Ctrl Pts',(-0.410641190037131,-0.214699828624725,
0.96));
#68056=CARTESIAN_POINT('Ctrl Pts',(-0.171896305307746,-0.214870357513428,
1.));
#68057=CARTESIAN_POINT('Ctrl Pts',(-0.171896305307746,-0.214870357513428,
0.96));
#68058=CARTESIAN_POINT('Ctrl Pts',(-0.217257824167609,-0.258526587486267,
1.));
#68059=CARTESIAN_POINT('Ctrl Pts',(-0.217257824167609,-0.258526587486267,
0.96));
#68060=CARTESIAN_POINT('Ctrl Pts',(-0.291268732771277,-0.258526587486267,
1.));
#68061=CARTESIAN_POINT('Ctrl Pts',(-0.291268732771277,-0.258526587486267,
0.96));
#68062=CARTESIAN_POINT('',(-0.171896305307746,-0.214870357513428,1.));
#68063=CARTESIAN_POINT('Ctrl Pts',(-0.171896305307746,-0.214870357513428,
1.));
#68064=CARTESIAN_POINT('Ctrl Pts',(-0.217257824167609,-0.258526587486267,
1.));
#68065=CARTESIAN_POINT('Ctrl Pts',(-0.291268732771277,-0.258526587486267,
1.));
#68066=CARTESIAN_POINT('',(-0.171896305307746,-0.214870357513428,0.96));
#68067=CARTESIAN_POINT('',(-0.171896305307746,-0.214870357513428,1.));
#68068=CARTESIAN_POINT('Ctrl Pts',(-0.171896305307746,-0.214870357513428,
0.96));
#68069=CARTESIAN_POINT('Ctrl Pts',(-0.217257824167609,-0.258526587486267,
0.96));
#68070=CARTESIAN_POINT('Ctrl Pts',(-0.291268732771277,-0.258526587486267,
0.96));
#68071=CARTESIAN_POINT('Ctrl Pts',(-0.126534726843238,-0.107094132900238,
1.));
#68072=CARTESIAN_POINT('Ctrl Pts',(-0.126534726843238,-0.107094132900238,
0.96));
#68073=CARTESIAN_POINT('Ctrl Pts',(-0.126534726843238,-0.171214127540588,
1.));
#68074=CARTESIAN_POINT('Ctrl Pts',(-0.126534726843238,-0.171214127540588,
0.96));
#68075=CARTESIAN_POINT('Ctrl Pts',(-0.171896305307746,-0.214870357513428,
1.));
#68076=CARTESIAN_POINT('Ctrl Pts',(-0.171896305307746,-0.214870357513428,
0.96));
#68077=CARTESIAN_POINT('',(-0.126534726843238,-0.107094132900238,1.));
#68078=CARTESIAN_POINT('Ctrl Pts',(-0.126534726843238,-0.107094132900238,
1.));
#68079=CARTESIAN_POINT('Ctrl Pts',(-0.126534726843238,-0.171214127540588,
1.));
#68080=CARTESIAN_POINT('Ctrl Pts',(-0.171896305307746,-0.214870357513428,
1.));
#68081=CARTESIAN_POINT('',(-0.126534726843238,-0.107094132900238,0.96));
#68082=CARTESIAN_POINT('',(-0.126534726843238,-0.107094132900238,1.));
#68083=CARTESIAN_POINT('Ctrl Pts',(-0.126534726843238,-0.107094132900238,
0.96));
#68084=CARTESIAN_POINT('Ctrl Pts',(-0.126534726843238,-0.171214127540588,
0.96));
#68085=CARTESIAN_POINT('Ctrl Pts',(-0.171896305307746,-0.214870357513428,
0.96));
#68086=CARTESIAN_POINT('Ctrl Pts',(-0.150579776987433,-0.0272850632667542,
1.));
#68087=CARTESIAN_POINT('Ctrl Pts',(-0.150579776987433,-0.0272850632667542,
0.96));
#68088=CARTESIAN_POINT('Ctrl Pts',(-0.126534726843238,-0.0607093811035156,
1.));
#68089=CARTESIAN_POINT('Ctrl Pts',(-0.126534726843238,-0.0607093811035156,
0.96));
#68090=CARTESIAN_POINT('Ctrl Pts',(-0.126534726843238,-0.107094132900238,
1.));
#68091=CARTESIAN_POINT('Ctrl Pts',(-0.126534726843238,-0.107094132900238,
0.96));
#68092=CARTESIAN_POINT('',(-0.150579776987433,-0.0272850632667542,1.));
#68093=CARTESIAN_POINT('Ctrl Pts',(-0.150579776987433,-0.0272850632667542,
1.));
#68094=CARTESIAN_POINT('Ctrl Pts',(-0.126534726843238,-0.0607093811035156,
1.));
#68095=CARTESIAN_POINT('Ctrl Pts',(-0.126534726843238,-0.107094132900238,
1.));
#68096=CARTESIAN_POINT('',(-0.150579776987433,-0.0272850632667542,0.96));
#68097=CARTESIAN_POINT('',(-0.150579776987433,-0.0272850632667542,1.));
#68098=CARTESIAN_POINT('Ctrl Pts',(-0.150579776987433,-0.0272850632667542,
0.96));
#68099=CARTESIAN_POINT('Ctrl Pts',(-0.126534726843238,-0.0607093811035156,
0.96));
#68100=CARTESIAN_POINT('Ctrl Pts',(-0.126534726843238,-0.107094132900238,
0.96));
#68101=CARTESIAN_POINT('Ctrl Pts',(-0.220668461546302,0.021146035194397,
1.));
#68102=CARTESIAN_POINT('Ctrl Pts',(-0.220668461546302,0.021146035194397,
0.96));
#68103=CARTESIAN_POINT('Ctrl Pts',(-0.174624797329307,0.00613919496536253,
1.));
#68104=CARTESIAN_POINT('Ctrl Pts',(-0.174624797329307,0.00613919496536253,
0.96));
#68105=CARTESIAN_POINT('Ctrl Pts',(-0.150579776987433,-0.0272850632667542,
1.));
#68106=CARTESIAN_POINT('Ctrl Pts',(-0.150579776987433,-0.0272850632667542,
0.96));
#68107=CARTESIAN_POINT('',(-0.220668461546302,0.021146035194397,1.));
#68108=CARTESIAN_POINT('Ctrl Pts',(-0.220668461546302,0.021146035194397,
1.));
#68109=CARTESIAN_POINT('Ctrl Pts',(-0.174624797329307,0.00613919496536253,
1.));
#68110=CARTESIAN_POINT('Ctrl Pts',(-0.150579776987433,-0.0272850632667542,
1.));
#68111=CARTESIAN_POINT('',(-0.220668461546302,0.021146035194397,0.96));
#68112=CARTESIAN_POINT('',(-0.220668461546302,0.021146035194397,1.));
#68113=CARTESIAN_POINT('Ctrl Pts',(-0.220668461546302,0.021146035194397,
0.96));
#68114=CARTESIAN_POINT('Ctrl Pts',(-0.174624797329307,0.00613919496536253,
0.96));
#68115=CARTESIAN_POINT('Ctrl Pts',(-0.150579776987433,-0.0272850632667542,
0.96));
#68116=CARTESIAN_POINT('Ctrl Pts',(-0.165245559439063,0.0608799815177917,
1.));
#68117=CARTESIAN_POINT('Ctrl Pts',(-0.165245559439063,0.0608799815177917,
0.96));
#68118=CARTESIAN_POINT('Ctrl Pts',(-0.183492478355765,0.0351296424865722,
1.));
#68119=CARTESIAN_POINT('Ctrl Pts',(-0.183492478355765,0.0351296424865722,
0.96));
#68120=CARTESIAN_POINT('Ctrl Pts',(-0.220668461546302,0.021146035194397,
1.));
#68121=CARTESIAN_POINT('Ctrl Pts',(-0.220668461546302,0.021146035194397,
0.96));
#68122=CARTESIAN_POINT('',(-0.165245559439063,0.0608799815177917,1.));
#68123=CARTESIAN_POINT('Ctrl Pts',(-0.165245559439063,0.0608799815177917,
1.));
#68124=CARTESIAN_POINT('Ctrl Pts',(-0.183492478355765,0.0351296424865722,
1.));
#68125=CARTESIAN_POINT('Ctrl Pts',(-0.220668461546302,0.021146035194397,
1.));
#68126=CARTESIAN_POINT('',(-0.165245559439063,0.0608799815177917,0.96));
#68127=CARTESIAN_POINT('',(-0.165245559439063,0.0608799815177917,1.));
#68128=CARTESIAN_POINT('Ctrl Pts',(-0.165245559439063,0.0608799815177917,
0.96));
#68129=CARTESIAN_POINT('Ctrl Pts',(-0.183492478355765,0.0351296424865722,
0.96));
#68130=CARTESIAN_POINT('Ctrl Pts',(-0.220668461546302,0.021146035194397,
0.96));
#68131=CARTESIAN_POINT('Ctrl Pts',(-0.146998610720038,0.121418869495392,
1.));
#68132=CARTESIAN_POINT('Ctrl Pts',(-0.146998610720038,0.121418869495392,
0.96));
#68133=CARTESIAN_POINT('Ctrl Pts',(-0.146998610720038,0.0866303205490112,
1.));
#68134=CARTESIAN_POINT('Ctrl Pts',(-0.146998610720038,0.0866303205490112,
0.96));
#68135=CARTESIAN_POINT('Ctrl Pts',(-0.165245559439063,0.0608799815177917,
1.));
#68136=CARTESIAN_POINT('Ctrl Pts',(-0.165245559439063,0.0608799815177917,
0.96));
#68137=CARTESIAN_POINT('',(-0.146998610720038,0.121418869495392,1.));
#68138=CARTESIAN_POINT('Ctrl Pts',(-0.146998610720038,0.121418869495392,
1.));
#68139=CARTESIAN_POINT('Ctrl Pts',(-0.146998610720038,0.0866303205490112,
1.));
#68140=CARTESIAN_POINT('Ctrl Pts',(-0.165245559439063,0.0608799815177917,
1.));
#68141=CARTESIAN_POINT('',(-0.146998610720038,0.121418869495392,0.96));
#68142=CARTESIAN_POINT('',(-0.146998610720038,0.121418869495392,1.));
#68143=CARTESIAN_POINT('Ctrl Pts',(-0.146998610720038,0.121418869495392,
0.96));
#68144=CARTESIAN_POINT('Ctrl Pts',(-0.146998610720038,0.0866303205490112,
0.96));
#68145=CARTESIAN_POINT('Ctrl Pts',(-0.165245559439063,0.0608799815177917,
0.96));
#68146=CARTESIAN_POINT('Ctrl Pts',(-0.186903115734458,0.214017784595489,
1.));
#68147=CARTESIAN_POINT('Ctrl Pts',(-0.186903115734458,0.214017784595489,
0.96));
#68148=CARTESIAN_POINT('Ctrl Pts',(-0.146998610720038,0.175989127159119,
1.));
#68149=CARTESIAN_POINT('Ctrl Pts',(-0.146998610720038,0.175989127159119,
0.96));
#68150=CARTESIAN_POINT('Ctrl Pts',(-0.146998610720038,0.121418869495392,
1.));
#68151=CARTESIAN_POINT('Ctrl Pts',(-0.146998610720038,0.121418869495392,
0.96));
#68152=CARTESIAN_POINT('',(-0.186903115734458,0.214017784595489,1.));
#68153=CARTESIAN_POINT('Ctrl Pts',(-0.186903115734458,0.214017784595489,
1.));
#68154=CARTESIAN_POINT('Ctrl Pts',(-0.146998610720038,0.175989127159119,
1.));
#68155=CARTESIAN_POINT('Ctrl Pts',(-0.146998610720038,0.121418869495392,
1.));
#68156=CARTESIAN_POINT('',(-0.186903115734458,0.214017784595489,0.96));
#68157=CARTESIAN_POINT('',(-0.186903115734458,0.214017784595489,1.));
#68158=CARTESIAN_POINT('Ctrl Pts',(-0.186903115734458,0.214017784595489,
0.96));
#68159=CARTESIAN_POINT('Ctrl Pts',(-0.146998610720038,0.175989127159119,
0.96));
#68160=CARTESIAN_POINT('Ctrl Pts',(-0.146998610720038,0.121418869495392,
0.96));
#68161=CARTESIAN_POINT('Ctrl Pts',(-0.292291965708137,0.252046382427216,
1.));
#68162=CARTESIAN_POINT('Ctrl Pts',(-0.292291965708137,0.252046382427216,
0.96));
#68163=CARTESIAN_POINT('Ctrl Pts',(-0.226807620748878,0.252046382427216,
1.));
#68164=CARTESIAN_POINT('Ctrl Pts',(-0.226807620748878,0.252046382427216,
0.96));
#68165=CARTESIAN_POINT('Ctrl Pts',(-0.186903115734458,0.214017784595489,
1.));
#68166=CARTESIAN_POINT('Ctrl Pts',(-0.186903115734458,0.214017784595489,
0.96));
#68167=CARTESIAN_POINT('',(-0.292291965708137,0.252046382427216,1.));
#68168=CARTESIAN_POINT('Ctrl Pts',(-0.292291965708137,0.252046382427216,
1.));
#68169=CARTESIAN_POINT('Ctrl Pts',(-0.226807620748878,0.252046382427216,
1.));
#68170=CARTESIAN_POINT('Ctrl Pts',(-0.186903115734458,0.214017784595489,
1.));
#68171=CARTESIAN_POINT('',(-0.292291965708137,0.252046382427216,0.96));
#68172=CARTESIAN_POINT('',(-0.292291965708137,0.252046382427216,1.));
#68173=CARTESIAN_POINT('Ctrl Pts',(-0.292291965708137,0.252046382427216,
0.96));
#68174=CARTESIAN_POINT('Ctrl Pts',(-0.226807620748878,0.252046382427216,
0.96));
#68175=CARTESIAN_POINT('Ctrl Pts',(-0.186903115734458,0.214017784595489,
0.96));
#68176=CARTESIAN_POINT('Ctrl Pts',(-0.396657552942634,0.214870429039001,
1.));
#68177=CARTESIAN_POINT('Ctrl Pts',(-0.396657552942634,0.214870429039001,
0.96));
#68178=CARTESIAN_POINT('Ctrl Pts',(-0.357435193285346,0.252046382427216,
1.));
#68179=CARTESIAN_POINT('Ctrl Pts',(-0.357435193285346,0.252046382427216,
0.96));
#68180=CARTESIAN_POINT('Ctrl Pts',(-0.292291965708137,0.252046382427216,
1.));
#68181=CARTESIAN_POINT('Ctrl Pts',(-0.292291965708137,0.252046382427216,
0.96));
#68182=CARTESIAN_POINT('',(-0.396657552942634,0.214870429039001,1.));
#68183=CARTESIAN_POINT('Ctrl Pts',(-0.396657552942634,0.214870429039001,
1.));
#68184=CARTESIAN_POINT('Ctrl Pts',(-0.357435193285346,0.252046382427216,
1.));
#68185=CARTESIAN_POINT('Ctrl Pts',(-0.292291965708137,0.252046382427216,
1.));
#68186=CARTESIAN_POINT('',(-0.396657552942634,0.214870429039001,0.96));
#68187=CARTESIAN_POINT('',(-0.396657552942634,0.214870429039001,1.));
#68188=CARTESIAN_POINT('Ctrl Pts',(-0.396657552942634,0.214870429039001,
0.96));
#68189=CARTESIAN_POINT('Ctrl Pts',(-0.357435193285346,0.252046382427216,
0.96));
#68190=CARTESIAN_POINT('Ctrl Pts',(-0.292291965708137,0.252046382427216,
0.96));
#68191=CARTESIAN_POINT('Ctrl Pts',(-0.435879942402244,0.123124188184738,
1.));
#68192=CARTESIAN_POINT('Ctrl Pts',(-0.435879942402244,0.123124188184738,
0.96));
#68193=CARTESIAN_POINT('Ctrl Pts',(-0.435879942402244,0.177694445848465,
1.));
#68194=CARTESIAN_POINT('Ctrl Pts',(-0.435879942402244,0.177694445848465,
0.96));
#68195=CARTESIAN_POINT('Ctrl Pts',(-0.396657552942634,0.214870429039001,
1.));
#68196=CARTESIAN_POINT('Ctrl Pts',(-0.396657552942634,0.214870429039001,
0.96));
#68197=CARTESIAN_POINT('',(-0.435879942402244,0.123124188184738,1.));
#68198=CARTESIAN_POINT('Ctrl Pts',(-0.435879942402244,0.123124188184738,
1.));
#68199=CARTESIAN_POINT('Ctrl Pts',(-0.435879942402244,0.177694445848465,
1.));
#68200=CARTESIAN_POINT('Ctrl Pts',(-0.396657552942634,0.214870429039001,
1.));
#68201=CARTESIAN_POINT('',(-0.435879942402244,0.123124188184738,0.96));
#68202=CARTESIAN_POINT('',(-0.435879942402244,0.123124188184738,1.));
#68203=CARTESIAN_POINT('Ctrl Pts',(-0.435879942402244,0.123124188184738,
0.96));
#68204=CARTESIAN_POINT('Ctrl Pts',(-0.435879942402244,0.177694445848465,
0.96));
#68205=CARTESIAN_POINT('Ctrl Pts',(-0.396657552942634,0.214870429039001,
0.96));
#68206=CARTESIAN_POINT('Ctrl Pts',(-0.417462464794517,0.0610505104064941,
1.));
#68207=CARTESIAN_POINT('Ctrl Pts',(-0.417462464794517,0.0610505104064941,
0.96));
#68208=CARTESIAN_POINT('Ctrl Pts',(-0.435879942402244,0.0869714081287384,
1.));
#68209=CARTESIAN_POINT('Ctrl Pts',(-0.435879942402244,0.0869714081287384,
0.96));
#68210=CARTESIAN_POINT('Ctrl Pts',(-0.435879942402244,0.123124188184738,
1.));
#68211=CARTESIAN_POINT('Ctrl Pts',(-0.435879942402244,0.123124188184738,
0.96));
#68212=CARTESIAN_POINT('',(-0.417462464794517,0.0610505104064941,1.));
#68213=CARTESIAN_POINT('Ctrl Pts',(-0.417462464794517,0.0610505104064941,
1.));
#68214=CARTESIAN_POINT('Ctrl Pts',(-0.435879942402244,0.0869714081287384,
1.));
#68215=CARTESIAN_POINT('Ctrl Pts',(-0.435879942402244,0.123124188184738,
1.));
#68216=CARTESIAN_POINT('',(-0.417462464794517,0.0610505104064941,0.96));
#68217=CARTESIAN_POINT('',(-0.417462464794517,0.0610505104064941,1.));
#68218=CARTESIAN_POINT('Ctrl Pts',(-0.417462464794517,0.0610505104064941,
0.96));
#68219=CARTESIAN_POINT('Ctrl Pts',(-0.435879942402244,0.0869714081287384,
0.96));
#68220=CARTESIAN_POINT('Ctrl Pts',(-0.435879942402244,0.123124188184738,
0.96));
#68221=CARTESIAN_POINT('Ctrl Pts',(-0.360845830664039,0.021146035194397,
1.));
#68222=CARTESIAN_POINT('Ctrl Pts',(-0.360845830664039,0.021146035194397,
0.96));
#68223=CARTESIAN_POINT('Ctrl Pts',(-0.399045016989112,0.0351296424865722,
1.));
#68224=CARTESIAN_POINT('Ctrl Pts',(-0.399045016989112,0.0351296424865722,
0.96));
#68225=CARTESIAN_POINT('Ctrl Pts',(-0.417462464794517,0.0610505104064941,
1.));
#68226=CARTESIAN_POINT('Ctrl Pts',(-0.417462464794517,0.0610505104064941,
0.96));
#68227=CARTESIAN_POINT('',(-0.360845830664039,0.021146035194397,1.));
#68228=CARTESIAN_POINT('Ctrl Pts',(-0.360845830664039,0.021146035194397,
1.));
#68229=CARTESIAN_POINT('Ctrl Pts',(-0.399045016989112,0.0351296424865722,
1.));
#68230=CARTESIAN_POINT('Ctrl Pts',(-0.417462464794517,0.0610505104064941,
1.));
#68231=CARTESIAN_POINT('',(-0.360845830664039,0.021146035194397,0.96));
#68232=CARTESIAN_POINT('',(-0.360845830664039,0.021146035194397,1.));
#68233=CARTESIAN_POINT('Ctrl Pts',(-0.360845830664039,0.021146035194397,
0.96));
#68234=CARTESIAN_POINT('Ctrl Pts',(-0.399045016989112,0.0351296424865722,
0.96));
#68235=CARTESIAN_POINT('Ctrl Pts',(-0.417462464794517,0.0610505104064941,
0.96));
#68236=CARTESIAN_POINT('Ctrl Pts',(-0.431275573000312,-0.0237038969993592,
1.));
#68237=CARTESIAN_POINT('Ctrl Pts',(-0.431275573000312,-0.0237038969993592,
0.96));
#68238=CARTESIAN_POINT('Ctrl Pts',(-0.406548422202468,0.00920877456665037,
1.));
#68239=CARTESIAN_POINT('Ctrl Pts',(-0.406548422202468,0.00920877456665037,
0.96));
#68240=CARTESIAN_POINT('Ctrl Pts',(-0.360845830664039,0.021146035194397,
1.));
#68241=CARTESIAN_POINT('Ctrl Pts',(-0.360845830664039,0.021146035194397,
0.96));
#68242=CARTESIAN_POINT('',(-0.431275573000312,-0.0237038969993592,1.));
#68243=CARTESIAN_POINT('Ctrl Pts',(-0.431275573000312,-0.0237038969993592,
1.));
#68244=CARTESIAN_POINT('Ctrl Pts',(-0.406548422202468,0.00920877456665037,
1.));
#68245=CARTESIAN_POINT('Ctrl Pts',(-0.360845830664039,0.021146035194397,
1.));
#68246=CARTESIAN_POINT('',(-0.431275573000312,-0.0237038969993592,0.96));
#68247=CARTESIAN_POINT('',(-0.431275573000312,-0.0237038969993592,1.));
#68248=CARTESIAN_POINT('Ctrl Pts',(-0.431275573000312,-0.0237038969993592,
0.96));
#68249=CARTESIAN_POINT('Ctrl Pts',(-0.406548422202468,0.00920877456665037,
0.96));
#68250=CARTESIAN_POINT('Ctrl Pts',(-0.360845830664039,0.021146035194397,
0.96));
#68251=CARTESIAN_POINT('Ctrl Pts',(-0.456002723798156,-0.105388784408569,
1.));
#68252=CARTESIAN_POINT('Ctrl Pts',(-0.456002723798156,-0.105388784408569,
0.96));
#68253=CARTESIAN_POINT('Ctrl Pts',(-0.456002723798156,-0.0566166281700134,
1.));
#68254=CARTESIAN_POINT('Ctrl Pts',(-0.456002723798156,-0.0566166281700134,
0.96));
#68255=CARTESIAN_POINT('Ctrl Pts',(-0.431275573000312,-0.0237038969993592,
1.));
#68256=CARTESIAN_POINT('Ctrl Pts',(-0.431275573000312,-0.0237038969993592,
0.96));
#68257=CARTESIAN_POINT('Ctrl Pts',(-0.456002723798156,-0.105388784408569,
1.));
#68258=CARTESIAN_POINT('Ctrl Pts',(-0.456002723798156,-0.0566166281700134,
1.));
#68259=CARTESIAN_POINT('Ctrl Pts',(-0.431275573000312,-0.0237038969993592,
1.));
#68260=CARTESIAN_POINT('Ctrl Pts',(-0.456002723798156,-0.105388784408569,
0.96));
#68261=CARTESIAN_POINT('Ctrl Pts',(-0.456002723798156,-0.0566166281700134,
0.96));
#68262=CARTESIAN_POINT('Ctrl Pts',(-0.431275573000312,-0.0237038969993592,
0.96));
#68263=CARTESIAN_POINT('Origin',(-0.291268725320697,-0.00324010252952578,
0.96));
#68264=CARTESIAN_POINT('Origin',(-0.0324011113494634,-0.180081808567047,
1.));
#68265=CARTESIAN_POINT('',(-0.0324011113494634,-0.180081808567047,1.));
#68266=CARTESIAN_POINT('',(0.0375170443207026,-0.180081808567047,1.));
#68267=CARTESIAN_POINT('',(-0.0162005556747317,-0.180081808567047,1.));
#68268=CARTESIAN_POINT('',(-0.0324011113494634,-0.180081808567047,0.96));
#68269=CARTESIAN_POINT('',(-0.0324011113494634,-0.180081808567047,1.));
#68270=CARTESIAN_POINT('',(0.0375170443207026,-0.180081808567047,0.96));
#68271=CARTESIAN_POINT('',(-0.0324011113494634,-0.180081808567047,0.96));
#68272=CARTESIAN_POINT('',(0.0375170443207026,-0.180081808567047,1.));
#68273=CARTESIAN_POINT('Origin',(-0.0324011113494634,-0.249999964237213,
1.));
#68274=CARTESIAN_POINT('',(-0.0324011113494634,-0.249999964237213,1.));
#68275=CARTESIAN_POINT('',(-0.0324011113494634,-0.124999982118607,1.));
#68276=CARTESIAN_POINT('',(-0.0324011113494634,-0.249999964237213,0.96));
#68277=CARTESIAN_POINT('',(-0.0324011113494634,-0.249999964237213,1.));
#68278=CARTESIAN_POINT('',(-0.0324011113494634,-0.249999964237213,0.96));
#68279=CARTESIAN_POINT('Origin',(0.0375170443207026,-0.249999964237213,
1.));
#68280=CARTESIAN_POINT('',(0.0375170443207026,-0.249999964237213,1.));
#68281=CARTESIAN_POINT('',(0.0187585221603513,-0.249999964237213,1.));
#68282=CARTESIAN_POINT('',(0.0375170443207026,-0.249999964237213,0.96));
#68283=CARTESIAN_POINT('',(0.0375170443207026,-0.249999964237213,1.));
#68284=CARTESIAN_POINT('',(0.0375170443207026,-0.249999964237213,0.96));
#68285=CARTESIAN_POINT('Origin',(0.0375170443207026,-0.180081808567047,
1.));
#68286=CARTESIAN_POINT('',(0.0375170443207026,-0.0900409042835236,1.));
#68287=CARTESIAN_POINT('',(0.0375170443207026,-0.180081808567047,0.96));
#68288=CARTESIAN_POINT('Origin',(0.00255796648561957,-0.21504088640213,
0.96));
#68289=CARTESIAN_POINT('Ctrl Pts',(0.29092774130404,0.201568937301636,1.));
#68290=CARTESIAN_POINT('Ctrl Pts',(0.29092774130404,0.201568937301636,0.96));
#68291=CARTESIAN_POINT('Ctrl Pts',(0.25579807497561,0.201568937301636,1.));
#68292=CARTESIAN_POINT('Ctrl Pts',(0.25579807497561,0.201568937301636,0.96));
#68293=CARTESIAN_POINT('Ctrl Pts',(0.232605788484216,0.179058706760406,
1.));
#68294=CARTESIAN_POINT('Ctrl Pts',(0.232605788484216,0.179058706760406,
0.96));
#68295=CARTESIAN_POINT('',(0.29092774130404,0.201568937301636,1.));
#68296=CARTESIAN_POINT('',(0.232605788484216,0.179058706760406,1.));
#68297=CARTESIAN_POINT('Ctrl Pts',(0.29092774130404,0.201568937301636,1.));
#68298=CARTESIAN_POINT('Ctrl Pts',(0.25579807497561,0.201568937301636,1.));
#68299=CARTESIAN_POINT('Ctrl Pts',(0.232605788484216,0.179058706760406,
1.));
#68300=CARTESIAN_POINT('',(0.29092774130404,0.201568937301636,0.96));
#68301=CARTESIAN_POINT('',(0.29092774130404,0.201568937301636,1.));
#68302=CARTESIAN_POINT('',(0.232605788484216,0.179058706760406,0.96));
#68303=CARTESIAN_POINT('Ctrl Pts',(0.29092774130404,0.201568937301636,0.96));
#68304=CARTESIAN_POINT('Ctrl Pts',(0.25579807497561,0.201568937301636,0.96));
#68305=CARTESIAN_POINT('Ctrl Pts',(0.232605788484216,0.179058706760406,
0.96));
#68306=CARTESIAN_POINT('',(0.232605788484216,0.179058706760406,1.));
#68307=CARTESIAN_POINT('Ctrl Pts',(0.349079224839807,0.178547120094299,
1.));
#68308=CARTESIAN_POINT('Ctrl Pts',(0.349079224839807,0.178547120094299,
0.96));
#68309=CARTESIAN_POINT('Ctrl Pts',(0.325716230645776,0.201568937301636,
1.));
#68310=CARTESIAN_POINT('Ctrl Pts',(0.325716230645776,0.201568937301636,
0.96));
#68311=CARTESIAN_POINT('Ctrl Pts',(0.29092774130404,0.201568937301636,1.));
#68312=CARTESIAN_POINT('Ctrl Pts',(0.29092774130404,0.201568937301636,0.96));
#68313=CARTESIAN_POINT('',(0.349079224839807,0.178547120094299,1.));
#68314=CARTESIAN_POINT('Ctrl Pts',(0.349079224839807,0.178547120094299,
1.));
#68315=CARTESIAN_POINT('Ctrl Pts',(0.325716230645776,0.201568937301636,
1.));
#68316=CARTESIAN_POINT('Ctrl Pts',(0.29092774130404,0.201568937301636,1.));
#68317=CARTESIAN_POINT('',(0.349079224839807,0.178547120094299,0.96));
#68318=CARTESIAN_POINT('',(0.349079224839807,0.178547120094299,1.));
#68319=CARTESIAN_POINT('Ctrl Pts',(0.349079224839807,0.178547120094299,
0.96));
#68320=CARTESIAN_POINT('Ctrl Pts',(0.325716230645776,0.201568937301636,
0.96));
#68321=CARTESIAN_POINT('Ctrl Pts',(0.29092774130404,0.201568937301636,0.96));
#68322=CARTESIAN_POINT('Ctrl Pts',(0.372442099824548,0.121759927272797,
1.));
#68323=CARTESIAN_POINT('Ctrl Pts',(0.372442099824548,0.121759927272797,
0.96));
#68324=CARTESIAN_POINT('Ctrl Pts',(0.372442099824548,0.15552527308464,1.));
#68325=CARTESIAN_POINT('Ctrl Pts',(0.372442099824548,0.15552527308464,0.96));
#68326=CARTESIAN_POINT('Ctrl Pts',(0.349079224839807,0.178547120094299,
1.));
#68327=CARTESIAN_POINT('Ctrl Pts',(0.349079224839807,0.178547120094299,
0.96));
#68328=CARTESIAN_POINT('',(0.372442099824548,0.121759927272797,1.));
#68329=CARTESIAN_POINT('Ctrl Pts',(0.372442099824548,0.121759927272797,
1.));
#68330=CARTESIAN_POINT('Ctrl Pts',(0.372442099824548,0.15552527308464,1.));
#68331=CARTESIAN_POINT('Ctrl Pts',(0.349079224839807,0.178547120094299,
1.));
#68332=CARTESIAN_POINT('',(0.372442099824548,0.121759927272797,0.96));
#68333=CARTESIAN_POINT('',(0.372442099824548,0.121759927272797,1.));
#68334=CARTESIAN_POINT('Ctrl Pts',(0.372442099824548,0.121759927272797,
0.96));
#68335=CARTESIAN_POINT('Ctrl Pts',(0.372442099824548,0.15552527308464,0.96));
#68336=CARTESIAN_POINT('Ctrl Pts',(0.349079224839807,0.178547120094299,
0.96));
#68337=CARTESIAN_POINT('Ctrl Pts',(0.349761340394616,0.0670191407203674,
1.));
#68338=CARTESIAN_POINT('Ctrl Pts',(0.349761340394616,0.0670191407203674,
0.96));
#68339=CARTESIAN_POINT('Ctrl Pts',(0.372442099824548,0.0893588423728943,
1.));
#68340=CARTESIAN_POINT('Ctrl Pts',(0.372442099824548,0.0893588423728943,
0.96));
#68341=CARTESIAN_POINT('Ctrl Pts',(0.372442099824548,0.121759927272797,
1.));
#68342=CARTESIAN_POINT('Ctrl Pts',(0.372442099824548,0.121759927272797,
0.96));
#68343=CARTESIAN_POINT('',(0.349761340394616,0.0670191407203674,1.));
#68344=CARTESIAN_POINT('Ctrl Pts',(0.349761340394616,0.0670191407203674,
1.));
#68345=CARTESIAN_POINT('Ctrl Pts',(0.372442099824548,0.0893588423728943,
1.));
#68346=CARTESIAN_POINT('Ctrl Pts',(0.372442099824548,0.121759927272797,
1.));
#68347=CARTESIAN_POINT('',(0.349761340394616,0.0670191407203674,0.96));
#68348=CARTESIAN_POINT('',(0.349761340394616,0.0670191407203674,1.));
#68349=CARTESIAN_POINT('Ctrl Pts',(0.349761340394616,0.0670191407203674,
0.96));
#68350=CARTESIAN_POINT('Ctrl Pts',(0.372442099824548,0.0893588423728943,
0.96));
#68351=CARTESIAN_POINT('Ctrl Pts',(0.372442099824548,0.121759927272797,
0.96));
#68352=CARTESIAN_POINT('Ctrl Pts',(0.29160985685885,0.0446794390678406,
1.));
#68353=CARTESIAN_POINT('Ctrl Pts',(0.29160985685885,0.0446794390678406,
0.96));
#68354=CARTESIAN_POINT('Ctrl Pts',(0.327080580964685,0.0446794390678406,
1.));
#68355=CARTESIAN_POINT('Ctrl Pts',(0.327080580964685,0.0446794390678406,
0.96));
#68356=CARTESIAN_POINT('Ctrl Pts',(0.349761340394616,0.0670191407203674,
1.));
#68357=CARTESIAN_POINT('Ctrl Pts',(0.349761340394616,0.0670191407203674,
0.96));
#68358=CARTESIAN_POINT('',(0.29160985685885,0.0446794390678406,1.));
#68359=CARTESIAN_POINT('Ctrl Pts',(0.29160985685885,0.0446794390678406,
1.));
#68360=CARTESIAN_POINT('Ctrl Pts',(0.327080580964685,0.0446794390678406,
1.));
#68361=CARTESIAN_POINT('Ctrl Pts',(0.349761340394616,0.0670191407203674,
1.));
#68362=CARTESIAN_POINT('',(0.29160985685885,0.0446794390678406,0.96));
#68363=CARTESIAN_POINT('',(0.29160985685885,0.0446794390678406,1.));
#68364=CARTESIAN_POINT('Ctrl Pts',(0.29160985685885,0.0446794390678406,
0.96));
#68365=CARTESIAN_POINT('Ctrl Pts',(0.327080580964685,0.0446794390678406,
0.96));
#68366=CARTESIAN_POINT('Ctrl Pts',(0.349761340394616,0.0670191407203674,
0.96));
#68367=CARTESIAN_POINT('Ctrl Pts',(0.232264730706811,0.0671896696090698,
1.));
#68368=CARTESIAN_POINT('Ctrl Pts',(0.232264730706811,0.0671896696090698,
0.96));
#68369=CARTESIAN_POINT('Ctrl Pts',(0.2551159594208,0.0446794390678406,1.));
#68370=CARTESIAN_POINT('Ctrl Pts',(0.2551159594208,0.0446794390678406,0.96));
#68371=CARTESIAN_POINT('Ctrl Pts',(0.29160985685885,0.0446794390678406,
1.));
#68372=CARTESIAN_POINT('Ctrl Pts',(0.29160985685885,0.0446794390678406,
0.96));
#68373=CARTESIAN_POINT('',(0.232264730706811,0.0671896696090698,1.));
#68374=CARTESIAN_POINT('Ctrl Pts',(0.232264730706811,0.0671896696090698,
1.));
#68375=CARTESIAN_POINT('Ctrl Pts',(0.2551159594208,0.0446794390678406,1.));
#68376=CARTESIAN_POINT('Ctrl Pts',(0.29160985685885,0.0446794390678406,
1.));
#68377=CARTESIAN_POINT('',(0.232264730706811,0.0671896696090698,0.96));
#68378=CARTESIAN_POINT('',(0.232264730706811,0.0671896696090698,1.));
#68379=CARTESIAN_POINT('Ctrl Pts',(0.232264730706811,0.0671896696090698,
0.96));
#68380=CARTESIAN_POINT('Ctrl Pts',(0.2551159594208,0.0446794390678406,0.96));
#68381=CARTESIAN_POINT('Ctrl Pts',(0.29160985685885,0.0446794390678406,
0.96));
#68382=CARTESIAN_POINT('Ctrl Pts',(0.209413382783532,0.125170594453812,
1.));
#68383=CARTESIAN_POINT('Ctrl Pts',(0.209413382783532,0.125170594453812,
0.96));
#68384=CARTESIAN_POINT('Ctrl Pts',(0.209413382783532,0.0896999001502991,
1.));
#68385=CARTESIAN_POINT('Ctrl Pts',(0.209413382783532,0.0896999001502991,
0.96));
#68386=CARTESIAN_POINT('Ctrl Pts',(0.232264730706811,0.0671896696090698,
1.));
#68387=CARTESIAN_POINT('Ctrl Pts',(0.232264730706811,0.0671896696090698,
0.96));
#68388=CARTESIAN_POINT('',(0.209413382783532,0.125170594453812,1.));
#68389=CARTESIAN_POINT('Ctrl Pts',(0.209413382783532,0.125170594453812,
1.));
#68390=CARTESIAN_POINT('Ctrl Pts',(0.209413382783532,0.0896999001502991,
1.));
#68391=CARTESIAN_POINT('Ctrl Pts',(0.232264730706811,0.0671896696090698,
1.));
#68392=CARTESIAN_POINT('',(0.209413382783532,0.125170594453812,0.96));
#68393=CARTESIAN_POINT('',(0.209413382783532,0.125170594453812,1.));
#68394=CARTESIAN_POINT('Ctrl Pts',(0.209413382783532,0.125170594453812,
0.96));
#68395=CARTESIAN_POINT('Ctrl Pts',(0.209413382783532,0.0896999001502991,
0.96));
#68396=CARTESIAN_POINT('Ctrl Pts',(0.232264730706811,0.0671896696090698,
0.96));
#68397=CARTESIAN_POINT('Ctrl Pts',(0.232605788484216,0.179058706760406,
1.));
#68398=CARTESIAN_POINT('Ctrl Pts',(0.232605788484216,0.179058706760406,
0.96));
#68399=CARTESIAN_POINT('Ctrl Pts',(0.209413382783532,0.156548476219177,
1.));
#68400=CARTESIAN_POINT('Ctrl Pts',(0.209413382783532,0.156548476219177,
0.96));
#68401=CARTESIAN_POINT('Ctrl Pts',(0.209413382783532,0.125170594453812,
1.));
#68402=CARTESIAN_POINT('Ctrl Pts',(0.209413382783532,0.125170594453812,
0.96));
#68403=CARTESIAN_POINT('Ctrl Pts',(0.232605788484216,0.179058706760406,
1.));
#68404=CARTESIAN_POINT('Ctrl Pts',(0.209413382783532,0.156548476219177,
1.));
#68405=CARTESIAN_POINT('Ctrl Pts',(0.209413382783532,0.125170594453812,
1.));
#68406=CARTESIAN_POINT('Ctrl Pts',(0.232605788484216,0.179058706760406,
0.96));
#68407=CARTESIAN_POINT('Ctrl Pts',(0.209413382783532,0.156548476219177,
0.96));
#68408=CARTESIAN_POINT('Ctrl Pts',(0.209413382783532,0.125170594453812,
0.96));
#68409=CARTESIAN_POINT('Ctrl Pts',(0.289904567971826,-0.00545700788497927,
1.));
#68410=CARTESIAN_POINT('Ctrl Pts',(0.289904567971826,-0.00545700788497927,
0.96));
#68411=CARTESIAN_POINT('Ctrl Pts',(0.246589395776391,-0.00545700788497927,
1.));
#68412=CARTESIAN_POINT('Ctrl Pts',(0.246589395776391,-0.00545700788497927,
0.96));
#68413=CARTESIAN_POINT('Ctrl Pts',(0.218110534921289,-0.0341063976287842,
1.));
#68414=CARTESIAN_POINT('Ctrl Pts',(0.218110534921289,-0.0341063976287842,
0.96));
#68415=CARTESIAN_POINT('',(0.289904567971826,-0.00545700788497927,1.));
#68416=CARTESIAN_POINT('',(0.218110534921289,-0.0341063976287842,1.));
#68417=CARTESIAN_POINT('Ctrl Pts',(0.289904567971826,-0.00545700788497927,
1.));
#68418=CARTESIAN_POINT('Ctrl Pts',(0.246589395776391,-0.00545700788497927,
1.));
#68419=CARTESIAN_POINT('Ctrl Pts',(0.218110534921289,-0.0341063976287842,
1.));
#68420=CARTESIAN_POINT('',(0.289904567971826,-0.00545700788497927,0.96));
#68421=CARTESIAN_POINT('',(0.289904567971826,-0.00545700788497927,1.));
#68422=CARTESIAN_POINT('',(0.218110534921289,-0.0341063976287842,0.96));
#68423=CARTESIAN_POINT('Ctrl Pts',(0.289904567971826,-0.00545700788497927,
0.96));
#68424=CARTESIAN_POINT('Ctrl Pts',(0.246589395776391,-0.00545700788497927,
0.96));
#68425=CARTESIAN_POINT('Ctrl Pts',(0.218110534921289,-0.0341063976287842,
0.96));
#68426=CARTESIAN_POINT('',(0.218110534921289,-0.0341063976287842,1.));
#68427=CARTESIAN_POINT('Ctrl Pts',(0.363744947686791,-0.034447455406189,
1.));
#68428=CARTESIAN_POINT('Ctrl Pts',(0.363744947686791,-0.034447455406189,
0.96));
#68429=CARTESIAN_POINT('Ctrl Pts',(0.334242913499475,-0.00545700788497927,
1.));
#68430=CARTESIAN_POINT('Ctrl Pts',(0.334242913499475,-0.00545700788497927,
0.96));
#68431=CARTESIAN_POINT('Ctrl Pts',(0.289904567971826,-0.00545700788497927,
1.));
#68432=CARTESIAN_POINT('Ctrl Pts',(0.289904567971826,-0.00545700788497927,
0.96));
#68433=CARTESIAN_POINT('',(0.363744947686791,-0.034447455406189,1.));
#68434=CARTESIAN_POINT('Ctrl Pts',(0.363744947686791,-0.034447455406189,
1.));
#68435=CARTESIAN_POINT('Ctrl Pts',(0.334242913499475,-0.00545700788497927,
1.));
#68436=CARTESIAN_POINT('Ctrl Pts',(0.289904567971826,-0.00545700788497927,
1.));
#68437=CARTESIAN_POINT('',(0.363744947686791,-0.034447455406189,0.96));
#68438=CARTESIAN_POINT('',(0.363744947686791,-0.034447455406189,1.));
#68439=CARTESIAN_POINT('Ctrl Pts',(0.363744947686791,-0.034447455406189,
0.96));
#68440=CARTESIAN_POINT('Ctrl Pts',(0.334242913499475,-0.00545700788497927,
0.96));
#68441=CARTESIAN_POINT('Ctrl Pts',(0.289904567971826,-0.00545700788497927,
0.96));
#68442=CARTESIAN_POINT('Ctrl Pts',(0.393246981874108,-0.107776248455048,
1.));
#68443=CARTESIAN_POINT('Ctrl Pts',(0.393246981874108,-0.107776248455048,
0.96));
#68444=CARTESIAN_POINT('Ctrl Pts',(0.393246981874108,-0.0634379029273987,
1.));
#68445=CARTESIAN_POINT('Ctrl Pts',(0.393246981874108,-0.0634379029273987,
0.96));
#68446=CARTESIAN_POINT('Ctrl Pts',(0.363744947686791,-0.034447455406189,
1.));
#68447=CARTESIAN_POINT('Ctrl Pts',(0.363744947686791,-0.034447455406189,
0.96));
#68448=CARTESIAN_POINT('',(0.393246981874108,-0.107776248455048,1.));
#68449=CARTESIAN_POINT('Ctrl Pts',(0.393246981874108,-0.107776248455048,
1.));
#68450=CARTESIAN_POINT('Ctrl Pts',(0.393246981874108,-0.0634379029273987,
1.));
#68451=CARTESIAN_POINT('Ctrl Pts',(0.363744947686791,-0.034447455406189,
1.));
#68452=CARTESIAN_POINT('',(0.393246981874108,-0.107776248455048,0.96));
#68453=CARTESIAN_POINT('',(0.393246981874108,-0.107776248455048,1.));
#68454=CARTESIAN_POINT('Ctrl Pts',(0.393246981874108,-0.107776248455048,
0.96));
#68455=CARTESIAN_POINT('Ctrl Pts',(0.393246981874108,-0.0634379029273987,
0.96));
#68456=CARTESIAN_POINT('Ctrl Pts',(0.363744947686791,-0.034447455406189,
0.96));
#68457=CARTESIAN_POINT('Ctrl Pts',(0.364597532525659,-0.179740750789642,
1.));
#68458=CARTESIAN_POINT('Ctrl Pts',(0.364597532525659,-0.179740750789642,
0.96));
#68459=CARTESIAN_POINT('Ctrl Pts',(0.393246981874108,-0.151432418823242,
1.));
#68460=CARTESIAN_POINT('Ctrl Pts',(0.393246981874108,-0.151432418823242,
0.96));
#68461=CARTESIAN_POINT('Ctrl Pts',(0.393246981874108,-0.107776248455048,
1.));
#68462=CARTESIAN_POINT('Ctrl Pts',(0.393246981874108,-0.107776248455048,
0.96));
#68463=CARTESIAN_POINT('',(0.364597532525659,-0.179740750789642,1.));
#68464=CARTESIAN_POINT('Ctrl Pts',(0.364597532525659,-0.179740750789642,
1.));
#68465=CARTESIAN_POINT('Ctrl Pts',(0.393246981874108,-0.151432418823242,
1.));
#68466=CARTESIAN_POINT('Ctrl Pts',(0.393246981874108,-0.107776248455048,
1.));
#68467=CARTESIAN_POINT('',(0.364597532525659,-0.179740750789642,0.96));
#68468=CARTESIAN_POINT('',(0.364597532525659,-0.179740750789642,1.));
#68469=CARTESIAN_POINT('Ctrl Pts',(0.364597532525659,-0.179740750789642,
0.96));
#68470=CARTESIAN_POINT('Ctrl Pts',(0.393246981874108,-0.151432418823242,
0.96));
#68471=CARTESIAN_POINT('Ctrl Pts',(0.393246981874108,-0.107776248455048,
0.96));
#68472=CARTESIAN_POINT('Ctrl Pts',(0.291950914636254,-0.208049082756043,
1.));
#68473=CARTESIAN_POINT('Ctrl Pts',(0.291950914636254,-0.208049082756043,
0.96));
#68474=CARTESIAN_POINT('Ctrl Pts',(0.335948202386498,-0.208049082756043,
1.));
#68475=CARTESIAN_POINT('Ctrl Pts',(0.335948202386498,-0.208049082756043,
0.96));
#68476=CARTESIAN_POINT('Ctrl Pts',(0.364597532525659,-0.179740750789642,
1.));
#68477=CARTESIAN_POINT('Ctrl Pts',(0.364597532525659,-0.179740750789642,
0.96));
#68478=CARTESIAN_POINT('',(0.291950914636254,-0.208049082756043,1.));
#68479=CARTESIAN_POINT('Ctrl Pts',(0.291950914636254,-0.208049082756043,
1.));
#68480=CARTESIAN_POINT('Ctrl Pts',(0.335948202386498,-0.208049082756043,
1.));
#68481=CARTESIAN_POINT('Ctrl Pts',(0.364597532525659,-0.179740750789642,
1.));
#68482=CARTESIAN_POINT('',(0.291950914636254,-0.208049082756043,0.96));
#68483=CARTESIAN_POINT('',(0.291950914636254,-0.208049082756043,1.));
#68484=CARTESIAN_POINT('Ctrl Pts',(0.291950914636254,-0.208049082756043,
0.96));
#68485=CARTESIAN_POINT('Ctrl Pts',(0.335948202386498,-0.208049082756043,
0.96));
#68486=CARTESIAN_POINT('Ctrl Pts',(0.364597532525659,-0.179740750789642,
0.96));
#68487=CARTESIAN_POINT('Ctrl Pts',(0.239086005464196,-0.194577062129974,
1.));
#68488=CARTESIAN_POINT('Ctrl Pts',(0.239086005464196,-0.194577062129974,
0.96));
#68489=CARTESIAN_POINT('Ctrl Pts',(0.263642642274499,-0.208049082756043,
1.));
#68490=CARTESIAN_POINT('Ctrl Pts',(0.263642642274499,-0.208049082756043,
0.96));
#68491=CARTESIAN_POINT('Ctrl Pts',(0.291950914636254,-0.208049082756043,
1.));
#68492=CARTESIAN_POINT('Ctrl Pts',(0.291950914636254,-0.208049082756043,
0.96));
#68493=CARTESIAN_POINT('',(0.239086005464196,-0.194577062129974,1.));
#68494=CARTESIAN_POINT('Ctrl Pts',(0.239086005464196,-0.194577062129974,
1.));
#68495=CARTESIAN_POINT('Ctrl Pts',(0.263642642274499,-0.208049082756043,
1.));
#68496=CARTESIAN_POINT('Ctrl Pts',(0.291950914636254,-0.208049082756043,
1.));
#68497=CARTESIAN_POINT('',(0.239086005464196,-0.194577062129974,0.96));
#68498=CARTESIAN_POINT('',(0.239086005464196,-0.194577062129974,1.));
#68499=CARTESIAN_POINT('Ctrl Pts',(0.239086005464196,-0.194577062129974,
0.96));
#68500=CARTESIAN_POINT('Ctrl Pts',(0.263642642274499,-0.208049082756043,
0.96));
#68501=CARTESIAN_POINT('Ctrl Pts',(0.291950914636254,-0.208049082756043,
0.96));
#68502=CARTESIAN_POINT('Ctrl Pts',(0.202080580964685,-0.156548404693604,
1.));
#68503=CARTESIAN_POINT('Ctrl Pts',(0.202080580964685,-0.156548404693604,
0.96));
#68504=CARTESIAN_POINT('Ctrl Pts',(0.214529368653893,-0.181104981899261,
1.));
#68505=CARTESIAN_POINT('Ctrl Pts',(0.214529368653893,-0.181104981899261,
0.96));
#68506=CARTESIAN_POINT('Ctrl Pts',(0.239086005464196,-0.194577062129974,
1.));
#68507=CARTESIAN_POINT('Ctrl Pts',(0.239086005464196,-0.194577062129974,
0.96));
#68508=CARTESIAN_POINT('',(0.202080580964685,-0.156548404693604,1.));
#68509=CARTESIAN_POINT('Ctrl Pts',(0.202080580964685,-0.156548404693604,
1.));
#68510=CARTESIAN_POINT('Ctrl Pts',(0.214529368653893,-0.181104981899261,
1.));
#68511=CARTESIAN_POINT('Ctrl Pts',(0.239086005464196,-0.194577062129974,
1.));
#68512=CARTESIAN_POINT('',(0.202080580964685,-0.156548404693604,0.96));
#68513=CARTESIAN_POINT('',(0.202080580964685,-0.156548404693604,1.));
#68514=CARTESIAN_POINT('Ctrl Pts',(0.202080580964685,-0.156548404693604,
0.96));
#68515=CARTESIAN_POINT('Ctrl Pts',(0.214529368653893,-0.181104981899261,
0.96));
#68516=CARTESIAN_POINT('Ctrl Pts',(0.239086005464196,-0.194577062129974,
0.96));
#68517=CARTESIAN_POINT('Ctrl Pts',(0.189631674066186,-0.105729842185974,
1.));
#68518=CARTESIAN_POINT('Ctrl Pts',(0.189631674066186,-0.105729842185974,
0.96));
#68519=CARTESIAN_POINT('Ctrl Pts',(0.189631674066186,-0.131991767883301,
1.));
#68520=CARTESIAN_POINT('Ctrl Pts',(0.189631674066186,-0.131991767883301,
0.96));
#68521=CARTESIAN_POINT('Ctrl Pts',(0.202080580964685,-0.156548404693604,
1.));
#68522=CARTESIAN_POINT('Ctrl Pts',(0.202080580964685,-0.156548404693604,
0.96));
#68523=CARTESIAN_POINT('',(0.189631674066186,-0.105729842185974,1.));
#68524=CARTESIAN_POINT('Ctrl Pts',(0.189631674066186,-0.105729842185974,
1.));
#68525=CARTESIAN_POINT('Ctrl Pts',(0.189631674066186,-0.131991767883301,
1.));
#68526=CARTESIAN_POINT('Ctrl Pts',(0.202080580964685,-0.156548404693604,
1.));
#68527=CARTESIAN_POINT('',(0.189631674066186,-0.105729842185974,0.96));
#68528=CARTESIAN_POINT('',(0.189631674066186,-0.105729842185974,1.));
#68529=CARTESIAN_POINT('Ctrl Pts',(0.189631674066186,-0.105729842185974,
0.96));
#68530=CARTESIAN_POINT('Ctrl Pts',(0.189631674066186,-0.131991767883301,
0.96));
#68531=CARTESIAN_POINT('Ctrl Pts',(0.202080580964685,-0.156548404693604,
0.96));
#68532=CARTESIAN_POINT('Ctrl Pts',(0.218110534921289,-0.0341063976287842,
1.));
#68533=CARTESIAN_POINT('Ctrl Pts',(0.218110534921289,-0.0341063976287842,
0.96));
#68534=CARTESIAN_POINT('Ctrl Pts',(0.189631674066186,-0.0627557873725891,
1.));
#68535=CARTESIAN_POINT('Ctrl Pts',(0.189631674066186,-0.0627557873725891,
0.96));
#68536=CARTESIAN_POINT('Ctrl Pts',(0.189631674066186,-0.105729842185974,
1.));
#68537=CARTESIAN_POINT('Ctrl Pts',(0.189631674066186,-0.105729842185974,
0.96));
#68538=CARTESIAN_POINT('Ctrl Pts',(0.218110534921289,-0.0341063976287842,
1.));
#68539=CARTESIAN_POINT('Ctrl Pts',(0.189631674066186,-0.0627557873725891,
1.));
#68540=CARTESIAN_POINT('Ctrl Pts',(0.189631674066186,-0.105729842185974,
1.));
#68541=CARTESIAN_POINT('Ctrl Pts',(0.218110534921289,-0.0341063976287842,
0.96));
#68542=CARTESIAN_POINT('Ctrl Pts',(0.189631674066186,-0.0627557873725891,
0.96));
#68543=CARTESIAN_POINT('Ctrl Pts',(0.189631674066186,-0.105729842185974,
0.96));
#68544=CARTESIAN_POINT('Ctrl Pts',(0.171896312013268,-0.214699828624725,
1.));
#68545=CARTESIAN_POINT('Ctrl Pts',(0.171896312013268,-0.214699828624725,
0.96));
#68546=CARTESIAN_POINT('Ctrl Pts',(0.126534793153405,-0.170873069763184,
1.));
#68547=CARTESIAN_POINT('Ctrl Pts',(0.126534793153405,-0.170873069763184,
0.96));
#68548=CARTESIAN_POINT('Ctrl Pts',(0.126534793153405,-0.105388784408569,
1.));
#68549=CARTESIAN_POINT('Ctrl Pts',(0.126534793153405,-0.105388784408569,
0.96));
#68550=CARTESIAN_POINT('',(0.171896312013268,-0.214699828624725,1.));
#68551=CARTESIAN_POINT('',(0.126534793153405,-0.105388784408569,1.));
#68552=CARTESIAN_POINT('Ctrl Pts',(0.171896312013268,-0.214699828624725,
1.));
#68553=CARTESIAN_POINT('Ctrl Pts',(0.126534793153405,-0.170873069763184,
1.));
#68554=CARTESIAN_POINT('Ctrl Pts',(0.126534793153405,-0.105388784408569,
1.));
#68555=CARTESIAN_POINT('',(0.171896312013268,-0.214699828624725,0.96));
#68556=CARTESIAN_POINT('',(0.171896312013268,-0.214699828624725,1.));
#68557=CARTESIAN_POINT('',(0.126534793153405,-0.105388784408569,0.96));
#68558=CARTESIAN_POINT('Ctrl Pts',(0.171896312013268,-0.214699828624725,
0.96));
#68559=CARTESIAN_POINT('Ctrl Pts',(0.126534793153405,-0.170873069763184,
0.96));
#68560=CARTESIAN_POINT('Ctrl Pts',(0.126534793153405,-0.105388784408569,
0.96));
#68561=CARTESIAN_POINT('',(0.126534793153405,-0.105388784408569,1.));
#68562=CARTESIAN_POINT('Ctrl Pts',(0.291268799081445,-0.258526587486267,
1.));
#68563=CARTESIAN_POINT('Ctrl Pts',(0.291268799081445,-0.258526587486267,
0.96));
#68564=CARTESIAN_POINT('Ctrl Pts',(0.217257830873132,-0.258526587486267,
1.));
#68565=CARTESIAN_POINT('Ctrl Pts',(0.217257830873132,-0.258526587486267,
0.96));
#68566=CARTESIAN_POINT('Ctrl Pts',(0.171896312013268,-0.214699828624725,
1.));
#68567=CARTESIAN_POINT('Ctrl Pts',(0.171896312013268,-0.214699828624725,
0.96));
#68568=CARTESIAN_POINT('',(0.291268799081445,-0.258526587486267,1.));
#68569=CARTESIAN_POINT('Ctrl Pts',(0.291268799081445,-0.258526587486267,
1.));
#68570=CARTESIAN_POINT('Ctrl Pts',(0.217257830873132,-0.258526587486267,
1.));
#68571=CARTESIAN_POINT('Ctrl Pts',(0.171896312013268,-0.214699828624725,
1.));
#68572=CARTESIAN_POINT('',(0.291268799081445,-0.258526587486267,0.96));
#68573=CARTESIAN_POINT('',(0.291268799081445,-0.258526587486267,1.));
#68574=CARTESIAN_POINT('Ctrl Pts',(0.291268799081445,-0.258526587486267,
0.96));
#68575=CARTESIAN_POINT('Ctrl Pts',(0.217257830873132,-0.258526587486267,
0.96));
#68576=CARTESIAN_POINT('Ctrl Pts',(0.171896312013268,-0.214699828624725,
0.96));
#68577=CARTESIAN_POINT('Ctrl Pts',(0.410641286149621,-0.214870357513428,
1.));
#68578=CARTESIAN_POINT('Ctrl Pts',(0.410641286149621,-0.214870357513428,
0.96));
#68579=CARTESIAN_POINT('Ctrl Pts',(0.365279767289758,-0.258526587486267,
1.));
#68580=CARTESIAN_POINT('Ctrl Pts',(0.365279767289758,-0.258526587486267,
0.96));
#68581=CARTESIAN_POINT('Ctrl Pts',(0.291268799081445,-0.258526587486267,
1.));
#68582=CARTESIAN_POINT('Ctrl Pts',(0.291268799081445,-0.258526587486267,
0.96));
#68583=CARTESIAN_POINT('',(0.410641286149621,-0.214870357513428,1.));
#68584=CARTESIAN_POINT('Ctrl Pts',(0.410641286149621,-0.214870357513428,
1.));
#68585=CARTESIAN_POINT('Ctrl Pts',(0.365279767289758,-0.258526587486267,
1.));
#68586=CARTESIAN_POINT('Ctrl Pts',(0.291268799081445,-0.258526587486267,
1.));
#68587=CARTESIAN_POINT('',(0.410641286149621,-0.214870357513428,0.96));
#68588=CARTESIAN_POINT('',(0.410641286149621,-0.214870357513428,1.));
#68589=CARTESIAN_POINT('Ctrl Pts',(0.410641286149621,-0.214870357513428,
0.96));
#68590=CARTESIAN_POINT('Ctrl Pts',(0.365279767289758,-0.258526587486267,
0.96));
#68591=CARTESIAN_POINT('Ctrl Pts',(0.291268799081445,-0.258526587486267,
0.96));
#68592=CARTESIAN_POINT('Ctrl Pts',(0.456002805009484,-0.107094132900238,
1.));
#68593=CARTESIAN_POINT('Ctrl Pts',(0.456002805009484,-0.107094132900238,
0.96));
#68594=CARTESIAN_POINT('Ctrl Pts',(0.456002805009484,-0.171214127540588,
1.));
#68595=CARTESIAN_POINT('Ctrl Pts',(0.456002805009484,-0.171214127540588,
0.96));
#68596=CARTESIAN_POINT('Ctrl Pts',(0.410641286149621,-0.214870357513428,
1.));
#68597=CARTESIAN_POINT('Ctrl Pts',(0.410641286149621,-0.214870357513428,
0.96));
#68598=CARTESIAN_POINT('',(0.456002805009484,-0.107094132900238,1.));
#68599=CARTESIAN_POINT('Ctrl Pts',(0.456002805009484,-0.107094132900238,
1.));
#68600=CARTESIAN_POINT('Ctrl Pts',(0.456002805009484,-0.171214127540588,
1.));
#68601=CARTESIAN_POINT('Ctrl Pts',(0.410641286149621,-0.214870357513428,
1.));
#68602=CARTESIAN_POINT('',(0.456002805009484,-0.107094132900238,0.96));
#68603=CARTESIAN_POINT('',(0.456002805009484,-0.107094132900238,1.));
#68604=CARTESIAN_POINT('Ctrl Pts',(0.456002805009484,-0.107094132900238,
0.96));
#68605=CARTESIAN_POINT('Ctrl Pts',(0.456002805009484,-0.171214127540588,
0.96));
#68606=CARTESIAN_POINT('Ctrl Pts',(0.410641286149621,-0.214870357513428,
0.96));
#68607=CARTESIAN_POINT('Ctrl Pts',(0.431957814469934,-0.0272850632667542,
1.));
#68608=CARTESIAN_POINT('Ctrl Pts',(0.431957814469934,-0.0272850632667542,
0.96));
#68609=CARTESIAN_POINT('Ctrl Pts',(0.456002805009484,-0.0607093811035156,
1.));
#68610=CARTESIAN_POINT('Ctrl Pts',(0.456002805009484,-0.0607093811035156,
0.96));
#68611=CARTESIAN_POINT('Ctrl Pts',(0.456002805009484,-0.107094132900238,
1.));
#68612=CARTESIAN_POINT('Ctrl Pts',(0.456002805009484,-0.107094132900238,
0.96));
#68613=CARTESIAN_POINT('',(0.431957814469934,-0.0272850632667542,1.));
#68614=CARTESIAN_POINT('Ctrl Pts',(0.431957814469934,-0.0272850632667542,
1.));
#68615=CARTESIAN_POINT('Ctrl Pts',(0.456002805009484,-0.0607093811035156,
1.));
#68616=CARTESIAN_POINT('Ctrl Pts',(0.456002805009484,-0.107094132900238,
1.));
#68617=CARTESIAN_POINT('',(0.431957814469934,-0.0272850632667542,0.96));
#68618=CARTESIAN_POINT('',(0.431957814469934,-0.0272850632667542,1.));
#68619=CARTESIAN_POINT('Ctrl Pts',(0.431957814469934,-0.0272850632667542,
0.96));
#68620=CARTESIAN_POINT('Ctrl Pts',(0.456002805009484,-0.0607093811035156,
0.96));
#68621=CARTESIAN_POINT('Ctrl Pts',(0.456002805009484,-0.107094132900238,
0.96));
#68622=CARTESIAN_POINT('Ctrl Pts',(0.36186907030642,0.021146035194397,1.));
#68623=CARTESIAN_POINT('Ctrl Pts',(0.36186907030642,0.021146035194397,0.96));
#68624=CARTESIAN_POINT('Ctrl Pts',(0.407912704721093,0.00613919496536253,
1.));
#68625=CARTESIAN_POINT('Ctrl Pts',(0.407912704721093,0.00613919496536253,
0.96));
#68626=CARTESIAN_POINT('Ctrl Pts',(0.431957814469934,-0.0272850632667542,
1.));
#68627=CARTESIAN_POINT('Ctrl Pts',(0.431957814469934,-0.0272850632667542,
0.96));
#68628=CARTESIAN_POINT('',(0.36186907030642,0.021146035194397,1.));
#68629=CARTESIAN_POINT('Ctrl Pts',(0.36186907030642,0.021146035194397,1.));
#68630=CARTESIAN_POINT('Ctrl Pts',(0.407912704721093,0.00613919496536253,
1.));
#68631=CARTESIAN_POINT('Ctrl Pts',(0.431957814469934,-0.0272850632667542,
1.));
#68632=CARTESIAN_POINT('',(0.36186907030642,0.021146035194397,0.96));
#68633=CARTESIAN_POINT('',(0.36186907030642,0.021146035194397,1.));
#68634=CARTESIAN_POINT('Ctrl Pts',(0.36186907030642,0.021146035194397,0.96));
#68635=CARTESIAN_POINT('Ctrl Pts',(0.407912704721093,0.00613919496536253,
0.96));
#68636=CARTESIAN_POINT('Ctrl Pts',(0.431957814469934,-0.0272850632667542,
0.96));
#68637=CARTESIAN_POINT('Ctrl Pts',(0.417291972413659,0.0608799815177917,
1.));
#68638=CARTESIAN_POINT('Ctrl Pts',(0.417291972413659,0.0608799815177917,
0.96));
#68639=CARTESIAN_POINT('Ctrl Pts',(0.399045083299279,0.0351296424865722,
1.));
#68640=CARTESIAN_POINT('Ctrl Pts',(0.399045083299279,0.0351296424865722,
0.96));
#68641=CARTESIAN_POINT('Ctrl Pts',(0.36186907030642,0.021146035194397,1.));
#68642=CARTESIAN_POINT('Ctrl Pts',(0.36186907030642,0.021146035194397,0.96));
#68643=CARTESIAN_POINT('',(0.417291972413659,0.0608799815177917,1.));
#68644=CARTESIAN_POINT('Ctrl Pts',(0.417291972413659,0.0608799815177917,
1.));
#68645=CARTESIAN_POINT('Ctrl Pts',(0.399045083299279,0.0351296424865722,
1.));
#68646=CARTESIAN_POINT('Ctrl Pts',(0.36186907030642,0.021146035194397,1.));
#68647=CARTESIAN_POINT('',(0.417291972413659,0.0608799815177917,0.96));
#68648=CARTESIAN_POINT('',(0.417291972413659,0.0608799815177917,1.));
#68649=CARTESIAN_POINT('Ctrl Pts',(0.417291972413659,0.0608799815177917,
0.96));
#68650=CARTESIAN_POINT('Ctrl Pts',(0.399045083299279,0.0351296424865722,
0.96));
#68651=CARTESIAN_POINT('Ctrl Pts',(0.36186907030642,0.021146035194397,0.96));
#68652=CARTESIAN_POINT('Ctrl Pts',(0.435538980737329,0.121418869495392,
1.));
#68653=CARTESIAN_POINT('Ctrl Pts',(0.435538980737329,0.121418869495392,
0.96));
#68654=CARTESIAN_POINT('Ctrl Pts',(0.435538980737329,0.0866303205490112,
1.));
#68655=CARTESIAN_POINT('Ctrl Pts',(0.435538980737329,0.0866303205490112,
0.96));
#68656=CARTESIAN_POINT('Ctrl Pts',(0.417291972413659,0.0608799815177917,
1.));
#68657=CARTESIAN_POINT('Ctrl Pts',(0.417291972413659,0.0608799815177917,
0.96));
#68658=CARTESIAN_POINT('',(0.435538980737329,0.121418869495392,1.));
#68659=CARTESIAN_POINT('Ctrl Pts',(0.435538980737329,0.121418869495392,
1.));
#68660=CARTESIAN_POINT('Ctrl Pts',(0.435538980737329,0.0866303205490112,
1.));
#68661=CARTESIAN_POINT('Ctrl Pts',(0.417291972413659,0.0608799815177917,
1.));
#68662=CARTESIAN_POINT('',(0.435538980737329,0.121418869495392,0.96));
#68663=CARTESIAN_POINT('',(0.435538980737329,0.121418869495392,1.));
#68664=CARTESIAN_POINT('Ctrl Pts',(0.435538980737329,0.121418869495392,
0.96));
#68665=CARTESIAN_POINT('Ctrl Pts',(0.435538980737329,0.0866303205490112,
0.96));
#68666=CARTESIAN_POINT('Ctrl Pts',(0.417291972413659,0.0608799815177917,
0.96));
#68667=CARTESIAN_POINT('Ctrl Pts',(0.395634386315942,0.214017784595489,
1.));
#68668=CARTESIAN_POINT('Ctrl Pts',(0.395634386315942,0.214017784595489,
0.96));
#68669=CARTESIAN_POINT('Ctrl Pts',(0.435538980737329,0.175989127159119,
1.));
#68670=CARTESIAN_POINT('Ctrl Pts',(0.435538980737329,0.175989127159119,
0.96));
#68671=CARTESIAN_POINT('Ctrl Pts',(0.435538980737329,0.121418869495392,
1.));
#68672=CARTESIAN_POINT('Ctrl Pts',(0.435538980737329,0.121418869495392,
0.96));
#68673=CARTESIAN_POINT('',(0.395634386315942,0.214017784595489,1.));
#68674=CARTESIAN_POINT('Ctrl Pts',(0.395634386315942,0.214017784595489,
1.));
#68675=CARTESIAN_POINT('Ctrl Pts',(0.435538980737329,0.175989127159119,
1.));
#68676=CARTESIAN_POINT('Ctrl Pts',(0.435538980737329,0.121418869495392,
1.));
#68677=CARTESIAN_POINT('',(0.395634386315942,0.214017784595489,0.96));
#68678=CARTESIAN_POINT('',(0.395634386315942,0.214017784595489,1.));
#68679=CARTESIAN_POINT('Ctrl Pts',(0.395634386315942,0.214017784595489,
0.96));
#68680=CARTESIAN_POINT('Ctrl Pts',(0.435538980737329,0.175989127159119,
0.96));
#68681=CARTESIAN_POINT('Ctrl Pts',(0.435538980737329,0.121418869495392,
0.96));
#68682=CARTESIAN_POINT('Ctrl Pts',(0.29024562574923,0.252046382427216,1.));
#68683=CARTESIAN_POINT('Ctrl Pts',(0.29024562574923,0.252046382427216,0.96));
#68684=CARTESIAN_POINT('Ctrl Pts',(0.355729911103845,0.252046382427216,
1.));
#68685=CARTESIAN_POINT('Ctrl Pts',(0.355729911103845,0.252046382427216,
0.96));
#68686=CARTESIAN_POINT('Ctrl Pts',(0.395634386315942,0.214017784595489,
1.));
#68687=CARTESIAN_POINT('Ctrl Pts',(0.395634386315942,0.214017784595489,
0.96));
#68688=CARTESIAN_POINT('',(0.29024562574923,0.252046382427216,1.));
#68689=CARTESIAN_POINT('Ctrl Pts',(0.29024562574923,0.252046382427216,1.));
#68690=CARTESIAN_POINT('Ctrl Pts',(0.355729911103845,0.252046382427216,
1.));
#68691=CARTESIAN_POINT('Ctrl Pts',(0.395634386315942,0.214017784595489,
1.));
#68692=CARTESIAN_POINT('',(0.29024562574923,0.252046382427216,0.96));
#68693=CARTESIAN_POINT('',(0.29024562574923,0.252046382427216,1.));
#68694=CARTESIAN_POINT('Ctrl Pts',(0.29024562574923,0.252046382427216,0.96));
#68695=CARTESIAN_POINT('Ctrl Pts',(0.355729911103845,0.252046382427216,
0.96));
#68696=CARTESIAN_POINT('Ctrl Pts',(0.395634386315942,0.214017784595489,
0.96));
#68697=CARTESIAN_POINT('Ctrl Pts',(0.185880038514733,0.214870429039001,
1.));
#68698=CARTESIAN_POINT('Ctrl Pts',(0.185880038514733,0.214870429039001,
0.96));
#68699=CARTESIAN_POINT('Ctrl Pts',(0.225102398172021,0.252046382427216,
1.));
#68700=CARTESIAN_POINT('Ctrl Pts',(0.225102398172021,0.252046382427216,
0.96));
#68701=CARTESIAN_POINT('Ctrl Pts',(0.29024562574923,0.252046382427216,1.));
#68702=CARTESIAN_POINT('Ctrl Pts',(0.29024562574923,0.252046382427216,0.96));
#68703=CARTESIAN_POINT('',(0.185880038514733,0.214870429039001,1.));
#68704=CARTESIAN_POINT('Ctrl Pts',(0.185880038514733,0.214870429039001,
1.));
#68705=CARTESIAN_POINT('Ctrl Pts',(0.225102398172021,0.252046382427216,
1.));
#68706=CARTESIAN_POINT('Ctrl Pts',(0.29024562574923,0.252046382427216,1.));
#68707=CARTESIAN_POINT('',(0.185880038514733,0.214870429039001,0.96));
#68708=CARTESIAN_POINT('',(0.185880038514733,0.214870429039001,1.));
#68709=CARTESIAN_POINT('Ctrl Pts',(0.185880038514733,0.214870429039001,
0.96));
#68710=CARTESIAN_POINT('Ctrl Pts',(0.225102398172021,0.252046382427216,
0.96));
#68711=CARTESIAN_POINT('Ctrl Pts',(0.29024562574923,0.252046382427216,0.96));
#68712=CARTESIAN_POINT('Ctrl Pts',(0.146657559648156,0.123124188184738,
1.));
#68713=CARTESIAN_POINT('Ctrl Pts',(0.146657559648156,0.123124188184738,
0.96));
#68714=CARTESIAN_POINT('Ctrl Pts',(0.146657559648156,0.177694445848465,
1.));
#68715=CARTESIAN_POINT('Ctrl Pts',(0.146657559648156,0.177694445848465,
0.96));
#68716=CARTESIAN_POINT('Ctrl Pts',(0.185880038514733,0.214870429039001,
1.));
#68717=CARTESIAN_POINT('Ctrl Pts',(0.185880038514733,0.214870429039001,
0.96));
#68718=CARTESIAN_POINT('',(0.146657559648156,0.123124188184738,1.));
#68719=CARTESIAN_POINT('Ctrl Pts',(0.146657559648156,0.123124188184738,
1.));
#68720=CARTESIAN_POINT('Ctrl Pts',(0.146657559648156,0.177694445848465,
1.));
#68721=CARTESIAN_POINT('Ctrl Pts',(0.185880038514733,0.214870429039001,
1.));
#68722=CARTESIAN_POINT('',(0.146657559648156,0.123124188184738,0.96));
#68723=CARTESIAN_POINT('',(0.146657559648156,0.123124188184738,1.));
#68724=CARTESIAN_POINT('Ctrl Pts',(0.146657559648156,0.123124188184738,
0.96));
#68725=CARTESIAN_POINT('Ctrl Pts',(0.146657559648156,0.177694445848465,
0.96));
#68726=CARTESIAN_POINT('Ctrl Pts',(0.185880038514733,0.214870429039001,
0.96));
#68727=CARTESIAN_POINT('Ctrl Pts',(0.165075037255883,0.0610505104064941,
1.));
#68728=CARTESIAN_POINT('Ctrl Pts',(0.165075037255883,0.0610505104064941,
0.96));
#68729=CARTESIAN_POINT('Ctrl Pts',(0.146657559648156,0.0869714081287384,
1.));
#68730=CARTESIAN_POINT('Ctrl Pts',(0.146657559648156,0.0869714081287384,
0.96));
#68731=CARTESIAN_POINT('Ctrl Pts',(0.146657559648156,0.123124188184738,
1.));
#68732=CARTESIAN_POINT('Ctrl Pts',(0.146657559648156,0.123124188184738,
0.96));
#68733=CARTESIAN_POINT('',(0.165075037255883,0.0610505104064941,1.));
#68734=CARTESIAN_POINT('Ctrl Pts',(0.165075037255883,0.0610505104064941,
1.));
#68735=CARTESIAN_POINT('Ctrl Pts',(0.146657559648156,0.0869714081287384,
1.));
#68736=CARTESIAN_POINT('Ctrl Pts',(0.146657559648156,0.123124188184738,
1.));
#68737=CARTESIAN_POINT('',(0.165075037255883,0.0610505104064941,0.96));
#68738=CARTESIAN_POINT('',(0.165075037255883,0.0610505104064941,1.));
#68739=CARTESIAN_POINT('Ctrl Pts',(0.165075037255883,0.0610505104064941,
0.96));
#68740=CARTESIAN_POINT('Ctrl Pts',(0.146657559648156,0.0869714081287384,
0.96));
#68741=CARTESIAN_POINT('Ctrl Pts',(0.146657559648156,0.123124188184738,
0.96));
#68742=CARTESIAN_POINT('Ctrl Pts',(0.221691701188684,0.021146035194397,
1.));
#68743=CARTESIAN_POINT('Ctrl Pts',(0.221691701188684,0.021146035194397,
0.96));
#68744=CARTESIAN_POINT('Ctrl Pts',(0.18349251486361,0.0351296424865722,
1.));
#68745=CARTESIAN_POINT('Ctrl Pts',(0.18349251486361,0.0351296424865722,
0.96));
#68746=CARTESIAN_POINT('Ctrl Pts',(0.165075037255883,0.0610505104064941,
1.));
#68747=CARTESIAN_POINT('Ctrl Pts',(0.165075037255883,0.0610505104064941,
0.96));
#68748=CARTESIAN_POINT('',(0.221691701188684,0.021146035194397,1.));
#68749=CARTESIAN_POINT('Ctrl Pts',(0.221691701188684,0.021146035194397,
1.));
#68750=CARTESIAN_POINT('Ctrl Pts',(0.18349251486361,0.0351296424865722,
1.));
#68751=CARTESIAN_POINT('Ctrl Pts',(0.165075037255883,0.0610505104064941,
1.));
#68752=CARTESIAN_POINT('',(0.221691701188684,0.021146035194397,0.96));
#68753=CARTESIAN_POINT('',(0.221691701188684,0.021146035194397,1.));
#68754=CARTESIAN_POINT('Ctrl Pts',(0.221691701188684,0.021146035194397,
0.96));
#68755=CARTESIAN_POINT('Ctrl Pts',(0.18349251486361,0.0351296424865722,
0.96));
#68756=CARTESIAN_POINT('Ctrl Pts',(0.165075037255883,0.0610505104064941,
0.96));
#68757=CARTESIAN_POINT('Ctrl Pts',(0.151262018457055,-0.0237038969993592,
1.));
#68758=CARTESIAN_POINT('Ctrl Pts',(0.151262018457055,-0.0237038969993592,
0.96));
#68759=CARTESIAN_POINT('Ctrl Pts',(0.175989124551415,0.00920877456665037,
1.));
#68760=CARTESIAN_POINT('Ctrl Pts',(0.175989124551415,0.00920877456665037,
0.96));
#68761=CARTESIAN_POINT('Ctrl Pts',(0.221691701188684,0.021146035194397,
1.));
#68762=CARTESIAN_POINT('Ctrl Pts',(0.221691701188684,0.021146035194397,
0.96));
#68763=CARTESIAN_POINT('',(0.151262018457055,-0.0237038969993592,1.));
#68764=CARTESIAN_POINT('Ctrl Pts',(0.151262018457055,-0.0237038969993592,
1.));
#68765=CARTESIAN_POINT('Ctrl Pts',(0.175989124551415,0.00920877456665037,
1.));
#68766=CARTESIAN_POINT('Ctrl Pts',(0.221691701188684,0.021146035194397,
1.));
#68767=CARTESIAN_POINT('',(0.151262018457055,-0.0237038969993592,0.96));
#68768=CARTESIAN_POINT('',(0.151262018457055,-0.0237038969993592,1.));
#68769=CARTESIAN_POINT('Ctrl Pts',(0.151262018457055,-0.0237038969993592,
0.96));
#68770=CARTESIAN_POINT('Ctrl Pts',(0.175989124551415,0.00920877456665037,
0.96));
#68771=CARTESIAN_POINT('Ctrl Pts',(0.221691701188684,0.021146035194397,
0.96));
#68772=CARTESIAN_POINT('Ctrl Pts',(0.126534793153405,-0.105388784408569,
1.));
#68773=CARTESIAN_POINT('Ctrl Pts',(0.126534793153405,-0.105388784408569,
0.96));
#68774=CARTESIAN_POINT('Ctrl Pts',(0.126534793153405,-0.0566166281700134,
1.));
#68775=CARTESIAN_POINT('Ctrl Pts',(0.126534793153405,-0.0566166281700134,
0.96));
#68776=CARTESIAN_POINT('Ctrl Pts',(0.151262018457055,-0.0237038969993592,
1.));
#68777=CARTESIAN_POINT('Ctrl Pts',(0.151262018457055,-0.0237038969993592,
0.96));
#68778=CARTESIAN_POINT('Ctrl Pts',(0.126534793153405,-0.105388784408569,
1.));
#68779=CARTESIAN_POINT('Ctrl Pts',(0.126534793153405,-0.0566166281700134,
1.));
#68780=CARTESIAN_POINT('Ctrl Pts',(0.151262018457055,-0.0237038969993592,
1.));
#68781=CARTESIAN_POINT('Ctrl Pts',(0.126534793153405,-0.105388784408569,
0.96));
#68782=CARTESIAN_POINT('Ctrl Pts',(0.126534793153405,-0.0566166281700134,
0.96));
#68783=CARTESIAN_POINT('Ctrl Pts',(0.151262018457055,-0.0237038969993592,
0.96));
#68784=CARTESIAN_POINT('Origin',(0.291268799081445,-0.00324010252952578,
0.96));
#68785=CARTESIAN_POINT('Origin',(0.,0.,1.));
#68786=CARTESIAN_POINT('Origin',(0.,0.,1.));
#68787=CARTESIAN_POINT('Origin',(0.,0.,1.));
#68788=CARTESIAN_POINT('Origin',(0.,0.,1.));
#68789=CARTESIAN_POINT('Origin',(1.87869726832665E-16,-4.25270154953079E-17,
-0.0599999999999998));
#68790=CARTESIAN_POINT('Ctrl Pts',(0.564220937616133,0.373642629516334,
-0.0599999999999999));
#68791=CARTESIAN_POINT('Ctrl Pts',(0.554999902806836,0.390417265728263,
-0.06));
#68792=CARTESIAN_POINT('Ctrl Pts',(0.545076539942756,0.406773487088272,
-0.0599999999999998));
#68793=CARTESIAN_POINT('Ctrl Pts',(0.534474770141273,0.422664239409727,
-0.0599999999999997));
#68794=CARTESIAN_POINT('Ctrl Pts',(0.518439430377503,0.446699246521537,
-0.0599999999999996));
#68795=CARTESIAN_POINT('Ctrl Pts',(0.500853434182984,0.469670265905156,
-0.0600000000000004));
#68796=CARTESIAN_POINT('Ctrl Pts',(0.4818657358897,0.49147811068534,-0.0600000000000005));
#68797=CARTESIAN_POINT('Ctrl Pts',(0.475405651424852,0.498897678718297,
-0.0600000000000005));
#68798=CARTESIAN_POINT('Ctrl Pts',(0.46878307560605,0.506182489986116,-0.0600000000000007));
#68799=CARTESIAN_POINT('Ctrl Pts',(0.462003176886937,0.513328228135021,
-0.0600000000000008));
#68800=CARTESIAN_POINT('Ctrl Pts',(0.456208383549552,0.519435705183202,
-0.0600000000000009));
#68801=CARTESIAN_POINT('Ctrl Pts',(0.45029960428802,0.525440374114255,-0.06));
#68802=CARTESIAN_POINT('Ctrl Pts',(0.444288945418066,0.531331357726455,
-0.06));
#68803=CARTESIAN_POINT('Ctrl Pts',(0.419805435115621,0.555327388957209,
-0.0600000000000001));
#68804=CARTESIAN_POINT('Ctrl Pts',(0.393598452075611,0.577478902722108,
-0.0600000000000002));
#68805=CARTESIAN_POINT('Ctrl Pts',(0.365904584686211,0.597621427333679,
-0.0600000000000005));
#68806=CARTESIAN_POINT('Ctrl Pts',(0.355326984662029,0.605314811786729,
-0.0600000000000006));
#68807=CARTESIAN_POINT('Ctrl Pts',(0.344531984117663,0.612714798138308,
-0.0599999999999995));
#68808=CARTESIAN_POINT('Ctrl Pts',(0.33353112873019,0.619810852933279,-0.0599999999999995));
#68809=CARTESIAN_POINT('Ctrl Pts',(0.326461355727503,0.624371179821331,
-0.0599999999999995));
#68810=CARTESIAN_POINT('Ctrl Pts',(0.319305261975003,0.628806725629368,
-0.0600000000000005));
#68811=CARTESIAN_POINT('Ctrl Pts',(0.312069750178058,0.633112118087385,
-0.0600000000000004));
#68812=CARTESIAN_POINT('Ctrl Pts',(0.301086781020382,0.639647383857811,
-0.0600000000000004));
#68813=CARTESIAN_POINT('Ctrl Pts',(0.289938770881977,0.645872277100329,
-0.0599999999999999));
#68814=CARTESIAN_POINT('Ctrl Pts',(0.278638203951252,0.651779354610587,
-0.0599999999999998));
#68815=CARTESIAN_POINT('Ctrl Pts',(0.248488006514047,0.667539586314266,
-0.0599999999999998));
#68816=CARTESIAN_POINT('Ctrl Pts',(0.217254479547028,0.681040528771996,
-0.0600000000000008));
#68817=CARTESIAN_POINT('Ctrl Pts',(0.185214713477108,0.692275549523078,
-0.0600000000000008));
#68818=CARTESIAN_POINT('Ctrl Pts',(0.163435758734888,0.699912528143077,
-0.0600000000000008));
#68819=CARTESIAN_POINT('Ctrl Pts',(0.141283364114538,0.706501731226335,
-0.0600000000000006));
#68820=CARTESIAN_POINT('Ctrl Pts',(0.118836930295083,0.71202966809404,-0.0600000000000005));
#68821=CARTESIAN_POINT('Ctrl Pts',(0.101600177236571,0.716274604437963,
-0.0600000000000005));
#68822=CARTESIAN_POINT('Ctrl Pts',(0.0841898961222066,0.719893553076916,
-0.06));
#68823=CARTESIAN_POINT('Ctrl Pts',(0.066640643957318,0.722876340867067,
-0.0599999999999999));
#68824=CARTESIAN_POINT('Ctrl Pts',(0.0571917300477745,0.724482341212539,
-0.0599999999999999));
#68825=CARTESIAN_POINT('Ctrl Pts',(0.0476983252949259,0.725904193801259,
-0.0600000000000005));
#68826=CARTESIAN_POINT('Ctrl Pts',(0.0381937449141578,0.727136847640426,
-0.0600000000000004));
#68827=CARTESIAN_POINT('Ctrl Pts',(0.00262667264075837,0.731749559241503,
-0.0600000000000002));
#68828=CARTESIAN_POINT('Ctrl Pts',(-0.0331646305896378,0.733731011574693,
-0.06));
#68829=CARTESIAN_POINT('Ctrl Pts',(-0.0688851945093288,0.733054681865674,
-0.0599999999999999));
#68830=CARTESIAN_POINT('Ctrl Pts',(-0.100011196056527,0.732465345157086,
-0.0599999999999997));
#68831=CARTESIAN_POINT('Ctrl Pts',(-0.131084581015127,0.72985747823783,
-0.0600000000000001));
#68832=CARTESIAN_POINT('Ctrl Pts',(-0.161929396660483,0.725302428734695,
-0.0600000000000001));
#68833=CARTESIAN_POINT('Ctrl Pts',(-0.179884268169555,0.722650919013043,
-0.06));
#68834=CARTESIAN_POINT('Ctrl Pts',(-0.197761783439131,0.719338985371272,
-0.0600000000000004));
#68835=CARTESIAN_POINT('Ctrl Pts',(-0.215527051730703,0.715375574961876,
-0.0600000000000004));
#68836=CARTESIAN_POINT('Ctrl Pts',(-0.225777172638808,0.713088785072865,
-0.0600000000000004));
#68837=CARTESIAN_POINT('Ctrl Pts',(-0.235995395902091,0.710583358306907,
-0.0600000000000004));
#68838=CARTESIAN_POINT('Ctrl Pts',(-0.246143283251969,0.707869589519532,
-0.0600000000000003));
#68839=CARTESIAN_POINT('Ctrl Pts',(-0.280845547615335,0.698589439017892,
-0.0600000000000001));
#68840=CARTESIAN_POINT('Ctrl Pts',(-0.314784451676007,0.686866611325189,
-0.0600000000000013));
#68841=CARTESIAN_POINT('Ctrl Pts',(-0.347701200929954,0.672822676723929,
-0.0600000000000011));
#68842=CARTESIAN_POINT('Ctrl Pts',(-0.374455811938238,0.661407819066396,
-0.0600000000000009));
#68843=CARTESIAN_POINT('Ctrl Pts',(-0.400535660286788,0.648458458483484,
-0.0600000000000007));
#68844=CARTESIAN_POINT('Ctrl Pts',(-0.425798867633714,0.634014708143998,
-0.0600000000000007));
#68845=CARTESIAN_POINT('Ctrl Pts',(-0.440419184632767,0.625655824581885,
-0.0600000000000007));
#68846=CARTESIAN_POINT('Ctrl Pts',(-0.454765899488343,0.616796030051311,
-0.0600000000000007));
#68847=CARTESIAN_POINT('Ctrl Pts',(-0.468820720454222,0.607454901453629,
-0.0600000000000006));
#68848=CARTESIAN_POINT('Ctrl Pts',(-0.476475383557125,0.602367451916581,
-0.0600000000000006));
#68849=CARTESIAN_POINT('Ctrl Pts',(-0.484043443552845,0.597137188854445,
-0.0600000000000003));
#68850=CARTESIAN_POINT('Ctrl Pts',(-0.491521770420875,0.591767005742375,
-0.0600000000000004));
#68851=CARTESIAN_POINT('Ctrl Pts',(-0.497516875552335,0.58746192348264,
-0.0600000000000004));
#68852=CARTESIAN_POINT('Ctrl Pts',(-0.503453507366844,0.583067338002368,
-0.0600000000000002));
#68853=CARTESIAN_POINT('Ctrl Pts',(-0.509319859107208,0.578592953790838,
-0.0600000000000003));
#68854=CARTESIAN_POINT('Ctrl Pts',(-0.538206295805245,0.5565606887632,-0.0600000000000005));
#68855=CARTESIAN_POINT('Ctrl Pts',(-0.565457889840676,0.532549689384572,
-0.0600000000000006));
#68856=CARTESIAN_POINT('Ctrl Pts',(-0.590916862149367,0.506792766445156,
-0.0600000000000004));
#68857=CARTESIAN_POINT('Ctrl Pts',(-0.616583471997437,0.480825775949348,
-0.0600000000000003));
#68858=CARTESIAN_POINT('Ctrl Pts',(-0.640429074795126,0.45308353546991,
-0.0600000000000004));
#68859=CARTESIAN_POINT('Ctrl Pts',(-0.662265722032779,0.423759522339067,
-0.0600000000000004));
#68860=CARTESIAN_POINT('Ctrl Pts',(-0.676018847392074,0.405290715097877,
-0.0600000000000004));
#68861=CARTESIAN_POINT('Ctrl Pts',(-0.688974507348362,0.386193601376564,
-0.0600000000000005));
#68862=CARTESIAN_POINT('Ctrl Pts',(-0.701077753000059,0.366509473613423,
-0.0600000000000005));
#68863=CARTESIAN_POINT('',(0.7911,-9.68818082805471E-17,-0.0600000000000001));
#68864=CARTESIAN_POINT('Origin',(0.,0.,-0.0600000000000001));
#68865=CARTESIAN_POINT('',(-0.724732793080687,-0.317244732932517,-0.0599999999999999));
#68866=CARTESIAN_POINT('Origin',(0.,0.,-0.0600000000000001));
#68867=CARTESIAN_POINT('Ctrl Pts',(-0.724732793080687,-0.317244732932517,
-0.0599999999999997));
#68868=CARTESIAN_POINT('Ctrl Pts',(-0.714450380759048,-0.336937903853692,
-0.0599999999999997));
#68869=CARTESIAN_POINT('Ctrl Pts',(-0.703349785215869,-0.356164574870145,
-0.0599999999999997));
#68870=CARTESIAN_POINT('Ctrl Pts',(-0.69144548414381,-0.37486759263711,
-0.0599999999999997));
#68871=CARTESIAN_POINT('Ctrl Pts',(-0.674201669809379,-0.401959596099963,
-0.0599999999999997));
#68872=CARTESIAN_POINT('Ctrl Pts',(-0.655272167225403,-0.427953990204327,
-0.0600000000000001));
#68873=CARTESIAN_POINT('Ctrl Pts',(-0.634786796513414,-0.452716544678885,
-0.0599999999999998));
#68874=CARTESIAN_POINT('Ctrl Pts',(-0.625943879110367,-0.463405793459665,
-0.0599999999999997));
#68875=CARTESIAN_POINT('Ctrl Pts',(-0.616810792269047,-0.473865214589598,
-0.0599999999999995));
#68876=CARTESIAN_POINT('Ctrl Pts',(-0.607396992666966,-0.484082568711768,
-0.0599999999999995));
#68877=CARTESIAN_POINT('Ctrl Pts',(-0.600762905540228,-0.491282936290893,
-0.0599999999999995));
#68878=CARTESIAN_POINT('Ctrl Pts',(-0.59399520773963,-0.498356663864347,
-0.0599999999999999));
#68879=CARTESIAN_POINT('Ctrl Pts',(-0.587101581912719,-0.50529629740727,
-0.0599999999999999));
#68880=CARTESIAN_POINT('Ctrl Pts',(-0.561447885223103,-0.531121205593067,
-0.06));
#68881=CARTESIAN_POINT('Ctrl Pts',(-0.534036253371049,-0.555110192383224,
-0.0599999999999992));
#68882=CARTESIAN_POINT('Ctrl Pts',(-0.505053708225385,-0.577058137884389,
-0.0599999999999991));
#68883=CARTESIAN_POINT('Ctrl Pts',(-0.494424541121948,-0.585107409580043,
-0.0599999999999991));
#68884=CARTESIAN_POINT('Ctrl Pts',(-0.483583822744001,-0.592881716994318,
-0.0600000000000003));
#68885=CARTESIAN_POINT('Ctrl Pts',(-0.472540016063593,-0.60036928753405,
-0.0600000000000004));
#68886=CARTESIAN_POINT('Ctrl Pts',(-0.465321436044098,-0.605263399560527,
-0.0600000000000005));
#68887=CARTESIAN_POINT('Ctrl Pts',(-0.458016082683304,-0.610034988697207,
-0.0599999999999998));
#68888=CARTESIAN_POINT('Ctrl Pts',(-0.450626256800085,-0.614680536634416,
-0.0599999999999998));
#68889=CARTESIAN_POINT('Ctrl Pts',(-0.44377928707728,-0.618984822902397,
-0.0599999999999998));
#68890=CARTESIAN_POINT('Ctrl Pts',(-0.436867759283859,-0.623175873324015,
-0.06));
#68891=CARTESIAN_POINT('Ctrl Pts',(-0.429895671529333,-0.627250594422087,
-0.06));
#68892=CARTESIAN_POINT('Ctrl Pts',(-0.424514176663148,-0.630395719876964,
-0.06));
#68893=CARTESIAN_POINT('Ctrl Pts',(-0.419096249028614,-0.633471758380428,
-0.0600000000000006));
#68894=CARTESIAN_POINT('Ctrl Pts',(-0.41364286935094,-0.636477760421398,
-0.0600000000000006));
#68895=CARTESIAN_POINT('Ctrl Pts',(-0.382437517006967,-0.653678718062254,
-0.0600000000000007));
#68896=CARTESIAN_POINT('Ctrl Pts',(-0.35007282615117,-0.668590450667035,
-0.0600000000000001));
#68897=CARTESIAN_POINT('Ctrl Pts',(-0.316814221808171,-0.681152839764513,
-0.0600000000000002));
#68898=CARTESIAN_POINT('Ctrl Pts',(-0.283852732529365,-0.69360300301497,
-0.0600000000000004));
#68899=CARTESIAN_POINT('Ctrl Pts',(-0.250011984261866,-0.703745755096182,
-0.0600000000000001));
#68900=CARTESIAN_POINT('Ctrl Pts',(-0.215543393032759,-0.711472512578678,
-0.0599999999999999));
#68901=CARTESIAN_POINT('Ctrl Pts',(-0.204674264783505,-0.713909024052846,
-0.0599999999999999));
#68902=CARTESIAN_POINT('Ctrl Pts',(-0.193742728782231,-0.716104914100372,
-0.0600000000000004));
#68903=CARTESIAN_POINT('Ctrl Pts',(-0.182756823721076,-0.718055695088162,
-0.0600000000000004));
#68904=CARTESIAN_POINT('Ctrl Pts',(-0.175918855215345,-0.719269921761507,
-0.0600000000000004));
#68905=CARTESIAN_POINT('Ctrl Pts',(-0.169063474904282,-0.720388450438065,
-0.0600000000000006));
#68906=CARTESIAN_POINT('Ctrl Pts',(-0.162200941898156,-0.72140941413215,
-0.0600000000000006));
#68907=CARTESIAN_POINT('Ctrl Pts',(-0.127449530315254,-0.726579506503682,
-0.0600000000000006));
#68908=CARTESIAN_POINT('Ctrl Pts',(-0.0924516067775416,-0.729263481555391,
-0.0600000000000014));
#68909=CARTESIAN_POINT('Ctrl Pts',(-0.0574594945934324,-0.72938133341839,
-0.0600000000000012));
#68910=CARTESIAN_POINT('Ctrl Pts',(-0.027630035940758,-0.729481797696052,
-0.060000000000001));
#68911=CARTESIAN_POINT('Ctrl Pts',(0.00219580972971492,-0.727716416426016,
-0.0600000000000007));
#68912=CARTESIAN_POINT('Ctrl Pts',(0.0318469521835107,-0.724114769434076,
-0.0600000000000006));
#68913=CARTESIAN_POINT('Ctrl Pts',(0.0479356243986104,-0.72216052035318,
-0.0600000000000005));
#68914=CARTESIAN_POINT('Ctrl Pts',(0.0639727227373624,-0.719665181752117,
-0.0599999999999997));
#68915=CARTESIAN_POINT('Ctrl Pts',(0.0799293665208594,-0.716630325957448,
-0.0599999999999997));
#68916=CARTESIAN_POINT('Ctrl Pts',(0.0871442683202932,-0.715258095880054,
-0.0599999999999997));
#68917=CARTESIAN_POINT('Ctrl Pts',(0.0943427028482492,-0.713775535082417,
-0.0600000000000005));
#68918=CARTESIAN_POINT('Ctrl Pts',(0.101521897140979,-0.712182649561427,
-0.0600000000000005));
#68919=CARTESIAN_POINT('Ctrl Pts',(0.108504253187729,-0.710633437575268,
-0.0600000000000005));
#68920=CARTESIAN_POINT('Ctrl Pts',(0.115459879835767,-0.708981734404333,
-0.0600000000000009));
#68921=CARTESIAN_POINT('Ctrl Pts',(0.122383960481882,-0.707228903035257,
-0.0600000000000009));
#68922=CARTESIAN_POINT('Ctrl Pts',(0.155299370056219,-0.698896365420998,
-0.0600000000000008));
#68923=CARTESIAN_POINT('Ctrl Pts',(0.187522320328344,-0.688278118088817,
-0.0599999999999995));
#68924=CARTESIAN_POINT('Ctrl Pts',(0.218802043739288,-0.675429950655413,
-0.0599999999999997));
#68925=CARTESIAN_POINT('Ctrl Pts',(0.241942213387686,-0.66592511040558,
-0.0599999999999999));
#68926=CARTESIAN_POINT('Ctrl Pts',(0.264566024515351,-0.65519881750284,
-0.06));
#68927=CARTESIAN_POINT('Ctrl Pts',(0.286562207485726,-0.643258021344417,
-0.0600000000000002));
#68928=CARTESIAN_POINT('Ctrl Pts',(0.300602246187078,-0.635636278953248,
-0.0600000000000002));
#68929=CARTESIAN_POINT('Ctrl Pts',(0.314386374989223,-0.62751943179706,
-0.0600000000000001));
#68930=CARTESIAN_POINT('Ctrl Pts',(0.327891021984824,-0.618923601513977,
-0.06));
#68931=CARTESIAN_POINT('Ctrl Pts',(0.335107601460311,-0.614330183232413,
-0.06));
#68932=CARTESIAN_POINT('Ctrl Pts',(0.342244337517139,-0.609599960851706,
-0.0600000000000004));
#68933=CARTESIAN_POINT('Ctrl Pts',(0.349297374951807,-0.604735234968208,
-0.0600000000000003));
#68934=CARTESIAN_POINT('Ctrl Pts',(0.354530483740722,-0.60112577733915,
-0.0600000000000003));
#68935=CARTESIAN_POINT('Ctrl Pts',(0.359715650922231,-0.597443457431399,
-0.0600000000000008));
#68936=CARTESIAN_POINT('Ctrl Pts',(0.364844366648222,-0.593694722470919,
-0.0600000000000007));
#68937=CARTESIAN_POINT('Ctrl Pts',(0.391762620975772,-0.574019348271211,
-0.0600000000000006));
#68938=CARTESIAN_POINT('Ctrl Pts',(0.417186617116553,-0.552477930138312,
-0.0600000000000008));
#68939=CARTESIAN_POINT('Ctrl Pts',(0.44093118569783,-0.529249758345641,
-0.0600000000000006));
#68940=CARTESIAN_POINT('Ctrl Pts',(0.464233432423963,-0.506454288794062,
-0.0600000000000004));
#68941=CARTESIAN_POINT('Ctrl Pts',(0.485918907142877,-0.482033324451575,
-0.0600000000000005));
#68942=CARTESIAN_POINT('Ctrl Pts',(0.50577214775514,-0.456128464695498,
-0.0600000000000006));
#68943=CARTESIAN_POINT('Ctrl Pts',(0.516780263536972,-0.441764880378141,
-0.0600000000000006));
#68944=CARTESIAN_POINT('Ctrl Pts',(0.527224294979779,-0.426944672942178,
-0.06));
#68945=CARTESIAN_POINT('Ctrl Pts',(0.5370608629359,-0.411689834101531,-0.0600000000000001));
#68946=CARTESIAN_POINT('Ctrl Pts',(-0.292601934307104,0.610169646934147,
-2.97494887079529));
#68947=CARTESIAN_POINT('Ctrl Pts',(-0.393827994997909,0.561627505729252,
-2.96966816631922));
#68948=CARTESIAN_POINT('Ctrl Pts',(-0.571555357247122,0.41324396405726,
-2.95910675736706));
#68949=CARTESIAN_POINT('Ctrl Pts',(-0.6994873117981,0.0901905791434185,
-2.94326464393882));
#68950=CARTESIAN_POINT('Ctrl Pts',(-0.657692280887251,-0.254657867677908,
-2.92742253051059));
#68951=CARTESIAN_POINT('Ctrl Pts',(-0.456327777700922,-0.537761889174431,
-2.91158041708236));
#68952=CARTESIAN_POINT('Ctrl Pts',(-0.14424191559841,-0.690367492084008,
-2.89573830365411));
#68953=CARTESIAN_POINT('Ctrl Pts',(0.202839712455166,-0.675480941669175,
-2.87989619022589));
#68954=CARTESIAN_POINT('Ctrl Pts',(0.500707301958,-0.496697430942489,-2.86405407679764));
#68955=CARTESIAN_POINT('Ctrl Pts',(0.677088347387025,-0.197403558953597,
-2.84821196336941));
#68956=CARTESIAN_POINT('Ctrl Pts',(0.689188274048217,0.149787622898873,
-2.83236984994118));
#68957=CARTESIAN_POINT('Ctrl Pts',(0.534070984426596,0.460635224458885,
-2.81652773651294));
#68958=CARTESIAN_POINT('Ctrl Pts',(0.249372597829536,0.659719708601146,
-2.80068562308471));
#68959=CARTESIAN_POINT('Ctrl Pts',(-0.095830858278809,0.69873681536456,
-2.78484350965647));
#68960=CARTESIAN_POINT('Ctrl Pts',(-0.417782948255712,0.568220153665686,
-2.76900139622824));
#68961=CARTESIAN_POINT('Ctrl Pts',(-0.638368754645892,0.299836710863442,
-2.7531592828));
#68962=CARTESIAN_POINT('Ctrl Pts',(-0.704067736716126,-0.0412958101518603,
-2.73731716937176));
#68963=CARTESIAN_POINT('Ctrl Pts',(-0.598939416511963,-0.372408780057021,
-2.72147505594353));
#68964=CARTESIAN_POINT('Ctrl Pts',(-0.348490978460388,-0.613164545241514,
-2.7056329425153));
#68965=CARTESIAN_POINT('Ctrl Pts',(-0.0134884969402019,-0.705148767075711,
-2.68979082908706));
#68966=CARTESIAN_POINT('Ctrl Pts',(0.324786686361382,-0.626043393699459,
-2.67394871565883));
#68967=CARTESIAN_POINT('Ctrl Pts',(0.584259176083316,-0.395041691351842,
-2.65810660223059));
#68968=CARTESIAN_POINT('Ctrl Pts',(0.701973402101012,-0.068191388181339,
-2.64226448880235));
#68969=CARTESIAN_POINT('Ctrl Pts',(0.649368470484853,0.275204128232534,
-2.62642237537412));
#68970=CARTESIAN_POINT('Ctrl Pts',(0.439207867209178,0.551827121547341,
-2.61058026194588));
#68971=CARTESIAN_POINT('Ctrl Pts',(0.122482665136422,0.69456081044579,-2.59473814851765));
#68972=CARTESIAN_POINT('Ctrl Pts',(-0.223960392743318,0.668773852033162,
-2.57889603508941));
#68973=CARTESIAN_POINT('Ctrl Pts',(-0.516064147577321,0.480722912143853,
-2.56305392166118));
#68974=CARTESIAN_POINT('Ctrl Pts',(-0.682955735366548,0.176034616500302,
-2.54721180823294));
#68975=CARTESIAN_POINT('Ctrl Pts',(-0.684142404452695,-0.171364795411006,
-2.53136969480471));
#68976=CARTESIAN_POINT('Ctrl Pts',(-0.519336234411588,-0.477186125430353,
-2.51552758137647));
#68977=CARTESIAN_POINT('Ctrl Pts',(-0.228523993923267,-0.667228226979231,
-2.49968546794824));
#68978=CARTESIAN_POINT('Ctrl Pts',(0.117734811948404,-0.69538136064443,
-2.48384335452));
#68979=CARTESIAN_POINT('Ctrl Pts',(0.435427729238652,-0.554814757632145,
-2.46800124109176));
#68980=CARTESIAN_POINT('Ctrl Pts',(0.647473219121237,-0.279633962881997,
-2.45215912766353));
#68981=CARTESIAN_POINT('Ctrl Pts',(0.702422880414448,0.0633941617704607,
-2.43631701423529));
#68982=CARTESIAN_POINT('Ctrl Pts',(0.586944327597745,0.391041019558242,
-2.42047490080706));
#68983=CARTESIAN_POINT('Ctrl Pts',(0.329056015185207,0.623809956274138,
-2.40463278737882));
#68984=CARTESIAN_POINT('Ctrl Pts',(-0.0086708539911011,0.705224459989427,
-2.38879067395059));
#68985=CARTESIAN_POINT('Ctrl Pts',(-0.344293921879448,0.615531004932474,
-2.37294856052235));
#68986=CARTESIAN_POINT('Ctrl Pts',(-0.5963812737897,0.376491831185336,-2.35710644709412));
#68987=CARTESIAN_POINT('Ctrl Pts',(-0.70376918857369,0.0461047924910424,
-2.34126433366588));
#68988=CARTESIAN_POINT('Ctrl Pts',(-0.640402235743698,-0.295468609383107,
-2.32542222023765));
#68989=CARTESIAN_POINT('Ctrl Pts',(-0.42165508048436,-0.565352735712883,
-2.30958010680941));
#68990=CARTESIAN_POINT('Ctrl Pts',(-0.100602142852268,-0.698065850425191,
-2.29373799338118));
#68991=CARTESIAN_POINT('Ctrl Pts',(0.244859799696957,-0.661407893185951,
-2.27789587995294));
#68992=CARTESIAN_POINT('Ctrl Pts',(0.530911635409909,-0.46427315027114,
-2.26205376652471));
#68993=CARTESIAN_POINT('Ctrl Pts',(0.688148871832329,-0.154492242110101,
-2.24621165309647));
#68994=CARTESIAN_POINT('Ctrl Pts',(0.678421183651292,0.192772975931516,
-2.23036953966824));
#68995=CARTESIAN_POINT('Ctrl Pts',(0.50408879085726,0.493265865034647,-2.21452742624));
#68996=CARTESIAN_POINT('Ctrl Pts',(0.207449800749737,0.674078113311214,
-2.19868531281176));
#68997=CARTESIAN_POINT('Ctrl Pts',(-0.13952254273371,0.691339412116387,
-2.18284319938353));
#68998=CARTESIAN_POINT('Ctrl Pts',(-0.45264266065732,0.540861668478527,
-2.1670010859553));
#68999=CARTESIAN_POINT('Ctrl Pts',(-0.655938508277729,0.259155158225147,
-2.15115897252706));
#69000=CARTESIAN_POINT('Ctrl Pts',(-0.700084602026596,-0.0854299284886501,
-2.13531685909882));
#69001=CARTESIAN_POINT('Ctrl Pts',(-0.574369815989129,-0.409287230630185,
-2.11947474567059));
#69002=CARTESIAN_POINT('Ctrl Pts',(-0.309296212482741,-0.633839550375444,
-2.10363263224235));
#69003=CARTESIAN_POINT('Ctrl Pts',(0.0308216451249593,-0.704603965975287,
-2.08779051881412));
#69004=CARTESIAN_POINT('Ctrl Pts',(0.363461275469507,-0.60441097269192,
-2.07194840538588));
#69005=CARTESIAN_POINT('Ctrl Pts',(0.607914632553942,-0.357570303860817,
-2.05610629195764));
#69006=CARTESIAN_POINT('Ctrl Pts',(0.704870224337332,-0.0239726827650286,
-2.04026417852942));
#69007=CARTESIAN_POINT('Ctrl Pts',(0.630803805217274,0.315441408188147,
-2.02442206510117));
#69008=CARTESIAN_POINT('Ctrl Pts',(0.403686041993089,0.578320241887024,
-2.00857995167294));
#69009=CARTESIAN_POINT('Ctrl Pts',(0.0786223075935471,0.700881769933403,
-1.9927378382447));
#69010=CARTESIAN_POINT('Ctrl Pts',(-0.265517484613883,0.653389002081171,
-1.97689572481647));
#69011=CARTESIAN_POINT('Ctrl Pts',(-0.545235014990942,0.44736506468894,
-1.96105361138823));
#69012=CARTESIAN_POINT('Ctrl Pts',(-0.692662677731179,0.132797355224364,
-1.94521149796));
#69013=CARTESIAN_POINT('Ctrl Pts',(-0.672030235315574,-0.213990853771854,
-1.92936938453176));
#69014=CARTESIAN_POINT('Ctrl Pts',(-0.488343718173467,-0.50885865974436,
-1.91352727110353));
#69015=CARTESIAN_POINT('Ctrl Pts',(-0.186170816147377,-0.680262559524874,
-1.8976851576753));
#69016=CARTESIAN_POINT('Ctrl Pts',(0.161172538892235,-0.686614983366474,
-1.88184304424706));
#69017=CARTESIAN_POINT('Ctrl Pts',(0.469410749818722,-0.526374648545063,
-1.86600093081882));
#69018=CARTESIAN_POINT('Ctrl Pts',(0.663756264470278,-0.238420519361853,
-1.85015881739059));
#69019=CARTESIAN_POINT('Ctrl Pts',(0.697055210292531,0.107381360022812,
-1.83431670396235));
#69020=CARTESIAN_POINT('Ctrl Pts',(0.561228294844321,0.427129399295399,
-1.81847459053412));
#69021=CARTESIAN_POINT('Ctrl Pts',(0.289231077053685,0.643243427282921,
-1.80263247710588));
#69022=CARTESIAN_POINT('Ctrl Pts',(-0.0529420095786137,0.703287897164517,
-1.78679036367765));
#69023=CARTESIAN_POINT('Ctrl Pts',(-0.382269825369864,0.592694274721806,
-1.77094825024941));
#69024=CARTESIAN_POINT('Ctrl Pts',(-0.618847866826519,0.338295788328172,
-1.75510613682118));
#69025=CARTESIAN_POINT('Ctrl Pts',(-0.705275422457957,0.00181690755493101,
-1.73926402339294));
#69026=CARTESIAN_POINT('Ctrl Pts',(-0.62058265434053,-0.335102807818698,
-1.72342190996471));
#69027=CARTESIAN_POINT('Ctrl Pts',(-0.385318490507109,-0.590716838721934,
-1.70757979653647));
#69028=CARTESIAN_POINT('Ctrl Pts',(-0.0565648575352245,-0.70300578914283,
-1.69173768310824));
#69029=CARTESIAN_POINT('Ctrl Pts',(0.285913054528226,-0.644725094847914,
-1.67589556968));
#69030=CARTESIAN_POINT('Ctrl Pts',(0.559020146487969,-0.430015346815531,
-1.66005345625177));
#69031=CARTESIAN_POINT('Ctrl Pts',(0.696492697099633,-0.110971372719233,
-1.64421134282353));
#69032=CARTESIAN_POINT('Ctrl Pts',(0.664975868496808,0.234997482950838,
-1.6283692293953));
#69033=CARTESIAN_POINT('Ctrl Pts',(0.472116559667202,0.523949116579385,
-1.61252711596706));
#69034=CARTESIAN_POINT('Ctrl Pts',(0.164708046420555,0.685775460424648,
-1.59668500253882));
#69035=CARTESIAN_POINT('Ctrl Pts',(-0.182663427862365,0.681212738282163,
-1.58084288911059));
#69036=CARTESIAN_POINT('Ctrl Pts',(-0.4857154435089,0.51136799920729,-1.56500077568235));
#69037=CARTESIAN_POINT('Ctrl Pts',(-0.670918770123565,0.217450515226326,
-1.54915866225412));
#69038=CARTESIAN_POINT('Ctrl Pts',(-0.693337695783756,-0.129226786238709,
-1.53331654882588));
#69039=CARTESIAN_POINT('Ctrl Pts',(-0.54753273728204,-0.444549912024228,
-1.51747443539765));
#69040=CARTESIAN_POINT('Ctrl Pts',(-0.268880416908177,-0.652012303625934,
-1.50163232196941));
#69041=CARTESIAN_POINT('Ctrl Pts',(0.0750101104497115,-0.701277552761128,
-1.48579020854118));
#69042=CARTESIAN_POINT('Ctrl Pts',(0.400701004053372,-0.580392477576107,
-1.46994809511294));
#69043=CARTESIAN_POINT('Ctrl Pts',(0.629170183477428,-0.318687312109054,
-1.45410598168471));
#69044=CARTESIAN_POINT('Ctrl Pts',(0.70498438292987,0.0203406612799057,
-1.43826386825647));
#69045=CARTESIAN_POINT('Ctrl Pts',(0.609748873285091,0.354433398826739,
-1.42242175482824));
#69046=CARTESIAN_POINT('Ctrl Pts',(0.366570558206358,0.602530288477345,
-1.4065796414));
#69047=CARTESIAN_POINT('Ctrl Pts',(0.034451567471494,0.704435811252572,
-1.39073752797176));
#69048=CARTESIAN_POINT('Ctrl Pts',(-0.306026375229727,0.63542472436951,
-1.37489541454353));
#69049=CARTESIAN_POINT('Ctrl Pts',(-0.57225342141949,0.412241124040289,
-1.35905330111529));
#69050=CARTESIAN_POINT('Ctrl Pts',(-0.699635148998229,0.089035840887468,
-1.34321118768706));
#69051=CARTESIAN_POINT('Ctrl Pts',(-0.657265047163405,-0.255772126029403,
-1.32736907425882));
#69052=CARTESIAN_POINT('Ctrl Pts',(-0.455423334553543,-0.538522338460017,
-1.31152696083059));
#69053=CARTESIAN_POINT('Ctrl Pts',(-0.143082679303674,-0.690611373754874,
-1.29568484740235));
#69054=CARTESIAN_POINT('Ctrl Pts',(0.203973994150782,-0.675138009881304,
-1.27984273397412));
#69055=CARTESIAN_POINT('Ctrl Pts',(0.501540645971156,-0.495856534811379,
-1.26400062054588));
#69056=CARTESIAN_POINT('Ctrl Pts',(0.677418954516088,-0.196265847101944,
-1.24815850711765));
#69057=CARTESIAN_POINT('Ctrl Pts',(0.688935728376574,0.150944641649023,
-1.23231639368941));
#69058=CARTESIAN_POINT('Ctrl Pts',(0.533296663357694,0.461531571539655,
-1.21647428026118));
#69059=CARTESIAN_POINT('Ctrl Pts',(0.248264321922183,0.660137522897185,
-1.20063216683294));
#69060=CARTESIAN_POINT('Ctrl Pts',(-0.0970041624297474,0.698574917347893,
-1.1847900534047));
#69061=CARTESIAN_POINT('Ctrl Pts',(-0.418736616528254,0.567517725410213,
-1.16894793997647));
#69062=CARTESIAN_POINT('Ctrl Pts',(-0.638871392465658,0.298764232406262,
-1.15310582654823));
#69063=CARTESIAN_POINT('Ctrl Pts',(-0.703997393063064,-0.0424781501094858,
-1.13726371312));
#69064=CARTESIAN_POINT('Ctrl Pts',(-0.598313157002194,-0.373414098333714,
-1.12142159969176));
#69065=CARTESIAN_POINT('Ctrl Pts',(-0.347460752777172,-0.613748929087322,
-1.10557948626353));
#69066=CARTESIAN_POINT('Ctrl Pts',(-0.0123042673209635,-0.705170424565585,
-1.08973737283529));
#69067=CARTESIAN_POINT('Ctrl Pts',(0.32583759114047,-0.625497071836542,
-1.07389525940706));
#69068=CARTESIAN_POINT('Ctrl Pts',(0.584921776088787,-0.394059942817653,
-1.05805314597882));
#69069=CARTESIAN_POINT('Ctrl Pts',(0.702086931244113,-0.0670124141673551,
-1.04221103255059));
#69070=CARTESIAN_POINT('Ctrl Pts',(0.648905383326142,0.276294274581765,
-1.02636891912235));
#69071=CARTESIAN_POINT('Ctrl Pts',(0.438280522141762,0.552563938913369,
-1.01052680569412));
#69072=CARTESIAN_POINT('Ctrl Pts',(0.121316063044922,0.694765525572184,
-0.994684692265882));
#69073=CARTESIAN_POINT('Ctrl Pts',(-0.225083200276113,0.668396795047505,
-0.978842578837647));
#69074=CARTESIAN_POINT('Ctrl Pts',(-0.51687073479559,0.479855568049576,
-0.963000465409411));
#69075=CARTESIAN_POINT('Ctrl Pts',(-0.68325040076027,0.174887428185227,
-0.947158351981176));
#69076=CARTESIAN_POINT('Ctrl Pts',(-0.683853653629245,-0.172513486702478,
-0.931316238552941));
#69077=CARTESIAN_POINT('Ctrl Pts',(-0.518534126716599,-0.478057613794162,
-0.915474125124705));
#69078=CARTESIAN_POINT('Ctrl Pts',(-0.22740314400511,-0.66761106399827,
-0.89963201169647));
#69079=CARTESIAN_POINT('Ctrl Pts',(0.118902453310195,-0.695182658927227,
-0.883789898268235));
#69080=CARTESIAN_POINT('Ctrl Pts',(0.436358858299948,-0.55408272799238,
-0.86794778484));
#69081=CARTESIAN_POINT('Ctrl Pts',(0.647941916898673,-0.278546216994571,
-0.852105671411764));
#69082=CARTESIAN_POINT('Ctrl Pts',(0.702315427199591,0.0645737051265365,
-0.836263557983531));
#69083=CARTESIAN_POINT('Ctrl Pts',(0.586286794664772,0.392026168868892,
-0.820421444555292));
#69084=CARTESIAN_POINT('Ctrl Pts',(0.328007939141782,0.624361685672875,
-0.804579331127061));
#69085=CARTESIAN_POINT('Ctrl Pts',(-0.00985517942347469,0.705208903882278,
-0.788737217698822));
#69086=CARTESIAN_POINT('Ctrl Pts',(-0.345327144915973,0.614951937683339,
-0.772895104270589));
#69087=CARTESIAN_POINT('Ctrl Pts',(-0.597012704480207,0.375489751345548,
-0.757052990842353));
#69088=CARTESIAN_POINT('Ctrl Pts',(-0.703845623473477,0.044922833765742,
-0.741210877414119));
#69089=CARTESIAN_POINT('Ctrl Pts',(-0.639905129523691,-0.296543669441083,
-0.725368763985881));
#69090=CARTESIAN_POINT('Ctrl Pts',(-0.420705045567162,-0.56606005627552,
-0.709526650557648));
#69091=CARTESIAN_POINT('Ctrl Pts',(-0.0994296853315642,-0.69823381495827,
-0.693684537129411));
#69092=CARTESIAN_POINT('Ctrl Pts',(0.245970207536815,-0.660995748610087,
-0.677842423701176));
#69093=CARTESIAN_POINT('Ctrl Pts',(0.531690576341267,-0.46338089484376,
-0.662000310272941));
#69094=CARTESIAN_POINT('Ctrl Pts',(0.688407352137116,-0.153336362940691,
-0.646158196844705));
#69095=CARTESIAN_POINT('Ctrl Pts',(0.678096488492109,0.193912028948647,
-0.630316083416472));
#69096=CARTESIAN_POINT('Ctrl Pts',(0.503259700720423,0.494111724518966,
-0.614473969988234));
#69097=CARTESIAN_POINT('Ctrl Pts',(0.206317477008665,0.674425549158015,
-0.598631856560001));
#69098=CARTESIAN_POINT('Ctrl Pts',(-0.140683365416483,0.691104126287348,
-0.582789743131764));
#69099=CARTESIAN_POINT('Ctrl Pts',(-0.453550332947481,0.540100748156837,
-0.56694762970353));
#69100=CARTESIAN_POINT('Ctrl Pts',(-0.656372802486486,0.258053224805003,
-0.551105516275294));
#69101=CARTESIAN_POINT('Ctrl Pts',(-0.699940145751841,-0.086605513920196,
-0.535263402847059));
#69102=CARTESIAN_POINT('Ctrl Pts',(-0.573681658522724,-0.410251236866699,
-0.519421289418823));
#69103=CARTESIAN_POINT('Ctrl Pts',(-0.308231320835643,-0.634358081474877,
-0.503579175990589));
#69104=CARTESIAN_POINT('Ctrl Pts',(0.032004897278945,-0.704551211216498,
-0.487737062562353));
#69105=CARTESIAN_POINT('Ctrl Pts',(0.364475796750062,-0.603799731912975,
-0.471894949134118));
#69106=CARTESIAN_POINT('Ctrl Pts',(0.60851427060865,-0.356548881847406,
-0.456052835705882));
#69107=CARTESIAN_POINT('Ctrl Pts',(0.704909489523639,-0.0227889061948828,
-0.440210722277648));
#69108=CARTESIAN_POINT('Ctrl Pts',(0.630273170690079,0.316500320697992,
-0.424368608849411));
#69109=CARTESIAN_POINT('Ctrl Pts',(0.402714255056845,0.578997367377502,
-0.408526495421177));
#69110=CARTESIAN_POINT('Ctrl Pts',(0.0774451521325488,0.701012818064358,
-0.39268438199294));
#69111=CARTESIAN_POINT('Ctrl Pts',(-0.26661439669049,0.652942176782176,
-0.376842268564707));
#69112=CARTESIAN_POINT('Ctrl Pts',(-0.545985540464761,0.446448778736983,
-0.36100015513647));
#69113=CARTESIAN_POINT('Ctrl Pts',(-0.692884718193416,0.131633926296123,
-0.345158041708236));
#69114=CARTESIAN_POINT('Ctrl Pts',(-0.671669915542376,-0.21511914411509,
-0.32931592828));
#69115=CARTESIAN_POINT('Ctrl Pts',(-0.487488465654378,-0.509678055216417,
-0.313473814851765));
#69116=CARTESIAN_POINT('Ctrl Pts',(-0.185028133270616,-0.680574251437019,
-0.297631701423529));
#69117=CARTESIAN_POINT('Ctrl Pts',(0.162325390816526,-0.68634334526228,
-0.281789587995294));
#69118=CARTESIAN_POINT('Ctrl Pts',(0.470294081325063,-0.525585589562447,
-0.265947474567059));
#69119=CARTESIAN_POINT('Ctrl Pts',(0.664155702788206,-0.237305484551378,
-0.250105361138824));
#69120=CARTESIAN_POINT('Ctrl Pts',(0.696873939840873,0.108551823732687,
-0.234263247710588));
#69121=CARTESIAN_POINT('Ctrl Pts',(0.560510101409974,0.428071317231208,
-0.218421134282353));
#69122=CARTESIAN_POINT('Ctrl Pts',(0.288150599099951,0.643728235591383,
-0.202579020854118));
#69123=CARTESIAN_POINT('Ctrl Pts',(-0.0541233696112858,0.703198020558049,
-0.186736907425882));
#69124=CARTESIAN_POINT('Ctrl Pts',(-0.383263958328779,0.592051415322255,
-0.170894793997647));
#69125=CARTESIAN_POINT('Ctrl Pts',(-0.61941646401829,0.337256127609639,
-0.155052680569412));
#69126=CARTESIAN_POINT('Ctrl Pts',(-0.70527484326665,0.000632295077805697,
-0.139210567141176));
#69127=CARTESIAN_POINT('Ctrl Pts',(-0.620024187785913,-0.33614416060722,
-0.123368453712941));
#69128=CARTESIAN_POINT('Ctrl Pts',(-0.384315741505486,-0.591363827723695,
-0.107526340284706));
#69129=CARTESIAN_POINT('Ctrl Pts',(-0.055404374357266,-0.703098282770509,
-0.091684226856471));
#69130=CARTESIAN_POINT('Ctrl Pts',(0.287037892597339,-0.644247893625522,
-0.0758421134282355));
#69131=CARTESIAN_POINT('Ctrl Pts',(0.468762250669717,-0.500787277377127,
-0.0652807044760785));
#69132=CARTESIAN_POINT('Ctrl Pts',(0.5370608629359,-0.411689834101531,-0.0600000000000001));
#69133=CARTESIAN_POINT('Ctrl Pts',(-0.309090610374651,0.644553868208601,
-2.9529325805302));
#69134=CARTESIAN_POINT('Ctrl Pts',(-0.416020952304324,0.593276284929997,
-2.94765187605412));
#69135=CARTESIAN_POINT('Ctrl Pts',(-0.603763589782005,0.436531048185212,
-2.93709046710196));
#69136=CARTESIAN_POINT('Ctrl Pts',(-0.738904753534814,0.0952729899872264,
-2.92124835367373));
#69137=CARTESIAN_POINT('Ctrl Pts',(-0.694754493060791,-0.269008323351198,
-2.90540624024549));
#69138=CARTESIAN_POINT('Ctrl Pts',(-0.482042716752689,-0.568065795445821,
-2.88956412681726));
#69139=CARTESIAN_POINT('Ctrl Pts',(-0.152370222156937,-0.729271014617091,
-2.87372201338902));
#69140=CARTESIAN_POINT('Ctrl Pts',(0.21427011642781,-0.713545578744666,
-2.85787989996079));
#69141=CARTESIAN_POINT('Ctrl Pts',(0.528923111693477,-0.524687276812066,
-2.84203778653255));
#69142=CARTESIAN_POINT('Ctrl Pts',(0.715243564834969,-0.208527625326828,
-2.82619567310431));
#69143=CARTESIAN_POINT('Ctrl Pts',(0.728025345399933,0.158228440621952,
-2.81035355967608));
#69144=CARTESIAN_POINT('Ctrl Pts',(0.564166901188532,0.486592896336179,
-2.79451144624784));
#69145=CARTESIAN_POINT('Ctrl Pts',(0.263425218484532,0.696896170186273,
-2.77866933281961));
#69146=CARTESIAN_POINT('Ctrl Pts',(-0.101231109590118,0.738111965198415,
-2.76282721939137));
#69147=CARTESIAN_POINT('Ctrl Pts',(-0.441325812784774,0.600240441129041,
-2.74698510596314));
#69148=CARTESIAN_POINT('Ctrl Pts',(-0.674342049326689,0.316733080363853,
-2.7311429925349));
#69149=CARTESIAN_POINT('Ctrl Pts',(-0.7437432941174,-0.0436229076748224,
-2.71530087910667));
#69150=CARTESIAN_POINT('Ctrl Pts',(-0.632690792921485,-0.393394723822608,
-2.69945876567843));
#69151=CARTESIAN_POINT('Ctrl Pts',(-0.368129108570174,-0.647717534737413,
-2.6836166522502));
#69152=CARTESIAN_POINT('Ctrl Pts',(-0.0142485994228211,-0.744885242595864,
-2.66777453882196));
#69153=CARTESIAN_POINT('Ctrl Pts',(0.343089034482034,-0.661322130825325,
-2.65193242539373));
#69154=CARTESIAN_POINT('Ctrl Pts',(0.617183292995749,-0.4173030427585,-2.63609031196549));
#69155=CARTESIAN_POINT('Ctrl Pts',(0.74153093975943,-0.0720341027313379,
-2.62024819853726));
#69156=CARTESIAN_POINT('Ctrl Pts',(0.685961620094956,0.290712404805016,
-2.60440608510902));
#69157=CARTESIAN_POINT('Ctrl Pts',(0.463958066711043,0.582923630440996,
-2.58856397168078));
#69158=CARTESIAN_POINT('Ctrl Pts',(0.12938479650513,0.733700634451997,-2.57272185825255));
#69159=CARTESIAN_POINT('Ctrl Pts',(-0.236580987260744,0.70646053183839,
-2.55687974482432));
#69160=CARTESIAN_POINT('Ctrl Pts',(-0.545145344800533,0.507812563466085,
-2.54103763139608));
#69161=CARTESIAN_POINT('Ctrl Pts',(-0.721441591297748,0.185954502283091,
-2.52519551796784));
#69162=CARTESIAN_POINT('Ctrl Pts',(-0.72269513144614,-0.181021527884781,
-2.50935340453961));
#69163=CARTESIAN_POINT('Ctrl Pts',(-0.548601819957467,-0.504076472087772,
-2.49351129111137));
#69164=CARTESIAN_POINT('Ctrl Pts',(-0.24140175605559,-0.704827807870036,
-2.47766917768314));
#69165=CARTESIAN_POINT('Ctrl Pts',(0.124369392750774,-0.734567424216532,
-2.4618270642549));
#69166=CARTESIAN_POINT('Ctrl Pts',(0.459964910769068,-0.586079625507186,
-2.44598495082667));
#69167=CARTESIAN_POINT('Ctrl Pts',(0.683959567708728,-0.295391869070711,
-2.43014283739843));
#69168=CARTESIAN_POINT('Ctrl Pts',(0.742005747031568,0.0669665434790141,
-2.41430072397019));
#69169=CARTESIAN_POINT('Ctrl Pts',(0.620019757910135,0.413076925492657,
-2.39845861054196));
#69170=CARTESIAN_POINT('Ctrl Pts',(0.347598948113237,0.658962834948961,
-2.38261649711372));
#69171=CARTESIAN_POINT('Ctrl Pts',(-0.00915947312147629,0.744965200949376,
-2.36677438368549));
#69172=CARTESIAN_POINT('Ctrl Pts',(-0.363695539860336,0.65021734893734,
-2.35093227025725));
#69173=CARTESIAN_POINT('Ctrl Pts',(-0.629988493986507,0.397707862655514,
-2.33509015682902));
#69174=CARTESIAN_POINT('Ctrl Pts',(-0.743427922218747,0.0487028853243916,
-2.31924804340078));
#69175=CARTESIAN_POINT('Ctrl Pts',(-0.676490120955796,-0.312118828048898,
-2.30340592997255));
#69176=CARTESIAN_POINT('Ctrl Pts',(-0.445416147036459,-0.597211438715468,
-2.28756381654432));
#69177=CARTESIAN_POINT('Ctrl Pts',(-0.106271265133095,-0.737403190107296,
-2.27172170311607));
#69178=CARTESIAN_POINT('Ctrl Pts',(0.258658115585497,-0.69867948718648,
-2.25587958968785));
#69179=CARTESIAN_POINT('Ctrl Pts',(0.560829516839833,-0.490435826194014,
-2.2400374762596));
#69180=CARTESIAN_POINT('Ctrl Pts',(0.726927370890315,-0.163198174082615,
-2.22419536283138));
#69181=CARTESIAN_POINT('Ctrl Pts',(0.716651508960247,0.203636100135525,
-2.20835324940314));
#69182=CARTESIAN_POINT('Ctrl Pts',(0.532495153930052,0.521062335632134,
-2.1925111359749));
#69183=CARTESIAN_POINT('Ctrl Pts',(0.21913999197469,0.712063698337962,-2.17666902254667));
#69184=CARTESIAN_POINT('Ctrl Pts',(-0.147384903646339,0.730297704193682,
-2.16082690911843));
#69185=CARTESIAN_POINT('Ctrl Pts',(-0.478149936347774,0.571340253215214,
-2.1449847956902));
#69186=CARTESIAN_POINT('Ctrl Pts',(-0.692901892025805,0.273759044782935,
-2.12914268226196));
#69187=CARTESIAN_POINT('Ctrl Pts',(-0.739535702204835,-0.0902440676045038,
-2.11330056883373));
#69188=CARTESIAN_POINT('Ctrl Pts',(-0.606736648632429,-0.4323513452965,
-2.09745845540549));
#69189=CARTESIAN_POINT('Ctrl Pts',(-0.326725642908844,-0.669557615772689,
-2.08161634197725));
#69190=CARTESIAN_POINT('Ctrl Pts',(0.0325585035074464,-0.744309740916213,
-2.06577422854902));
#69191=CARTESIAN_POINT('Ctrl Pts',(0.383943010316906,-0.63847068170919,
-2.04993211512078));
#69192=CARTESIAN_POINT('Ctrl Pts',(0.642171779474866,-0.377720071242564,
-2.03409000169255));
#69193=CARTESIAN_POINT('Ctrl Pts',(0.744591003443873,-0.0253235890791637,
-2.01824788826431));
#69194=CARTESIAN_POINT('Ctrl Pts',(0.666350800595265,0.333217132091755,
-2.00240577483608));
#69195=CARTESIAN_POINT('Ctrl Pts',(0.426434519015904,0.610909688550673,
-1.98656366140784));
#69196=CARTESIAN_POINT('Ctrl Pts',(0.0830528243112992,0.740377792040875,
-1.97072154797961));
#69197=CARTESIAN_POINT('Ctrl Pts',(-0.280479900376565,0.690208716301205,
-1.95487943455138));
#69198=CARTESIAN_POINT('Ctrl Pts',(-0.575960046129783,0.472574937798846,
-1.93903732112313));
#69199=CARTESIAN_POINT('Ctrl Pts',(-0.731695538345162,0.14028073901712,
-1.9231952076949));
#69200=CARTESIAN_POINT('Ctrl Pts',(-0.709900418518422,-0.226049645787761,
-1.90735309426667));
#69201=CARTESIAN_POINT('Ctrl Pts',(-0.515862816424316,-0.537533814010037,
-1.89151098083843));
#69202=CARTESIAN_POINT('Ctrl Pts',(-0.196661896078054,-0.71859664987,-1.8756688674102));
#69203=CARTESIAN_POINT('Ctrl Pts',(0.17025491830668,-0.725307044889122,
-1.85982675398196));
#69204=CARTESIAN_POINT('Ctrl Pts',(0.4958629392573,-0.556036862127428,-1.84398464055372));
#69205=CARTESIAN_POINT('Ctrl Pts',(0.701160193663617,-0.251855969544111,
-1.82814252712549));
#69206=CARTESIAN_POINT('Ctrl Pts',(0.736335598479057,0.113432504097785,
-1.81230041369725));
#69207=CARTESIAN_POINT('Ctrl Pts',(0.592854577751664,0.451198954134761,
-1.79645830026902));
#69208=CARTESIAN_POINT('Ctrl Pts',(0.305529798897411,0.679491419047446,
-1.78061618684078));
#69209=CARTESIAN_POINT('Ctrl Pts',(-0.055925392611856,0.742919509122363,
-1.76477407341255));
#69210=CARTESIAN_POINT('Ctrl Pts',(-0.403811457812752,0.626093725501658,
-1.74893195998431));
#69211=CARTESIAN_POINT('Ctrl Pts',(-0.653721122313909,0.357359400063925,
-1.73308984655608));
#69212=CARTESIAN_POINT('Ctrl Pts',(-0.745019035250031,0.00191929375476884,
-1.71724773312784));
#69213=CARTESIAN_POINT('Ctrl Pts',(-0.655553668407108,-0.353986489023787,
-1.70140561969961));
#69214=CARTESIAN_POINT('Ctrl Pts',(-0.407031921034679,-0.624004857218455,
-1.68556350627137));
#69215=CARTESIAN_POINT('Ctrl Pts',(-0.059752394948178,-0.742621503776561,
-1.66972139284314));
#69216=CARTESIAN_POINT('Ctrl Pts',(0.302024799485628,-0.681056581400599,
-1.6538792794149));
#69217=CARTESIAN_POINT('Ctrl Pts',(0.590521996031449,-0.45424753029206,
-1.63803716598667));
#69218=CARTESIAN_POINT('Ctrl Pts',(0.7357413865968,-0.117224820844492,-1.62219505255843));
#69219=CARTESIAN_POINT('Ctrl Pts',(0.702448524698983,0.248240038514392,
-1.6063529391302));
#69220=CARTESIAN_POINT('Ctrl Pts',(0.498721226642195,0.553474646817637,
-1.59051082570196));
#69221=CARTESIAN_POINT('Ctrl Pts',(0.173989658415294,0.724420213231198,
-1.57466871227373));
#69222=CARTESIAN_POINT('Ctrl Pts',(-0.192956859785644,0.719600373009261,
-1.55882659884549));
#69223=CARTESIAN_POINT('Ctrl Pts',(-0.513086433478563,0.540184559529105,
-1.54298448541725));
#69224=CARTESIAN_POINT('Ctrl Pts',(-0.708726320146782,0.229704265751867,
-1.52714237198902));
#69225=CARTESIAN_POINT('Ctrl Pts',(-0.732408594950133,-0.1365089616713,
-1.51130025856078));
#69226=CARTESIAN_POINT('Ctrl Pts',(-0.5783872494465,-0.469601145921851,
-1.49545814513255));
#69227=CARTESIAN_POINT('Ctrl Pts',(-0.284032340308158,-0.68875443826699,
-1.47961603170431));
#69228=CARTESIAN_POINT('Ctrl Pts',(0.0792370729813301,-0.740795877984452,
-1.46377391827608));
#69229=CARTESIAN_POINT('Ctrl Pts',(0.423281268505223,-0.613098698666059,
-1.44793180484784));
#69230=CARTESIAN_POINT('Ctrl Pts',(0.664625121160208,-0.336645948878317,
-1.43208969141961));
#69231=CARTESIAN_POINT('Ctrl Pts',(0.744711595090442,0.0214868962685335,
-1.41624757799137));
#69232=CARTESIAN_POINT('Ctrl Pts',(0.644109383163333,0.374406395637621,
-1.40040546456314));
#69233=CARTESIAN_POINT('Ctrl Pts',(0.387227507055584,0.636484017358584,
-1.3845633511349));
#69234=CARTESIAN_POINT('Ctrl Pts',(0.0363929788890332,0.744132110354732,
-1.36872123770667));
#69235=CARTESIAN_POINT('Ctrl Pts',(-0.323271544101347,0.671232117339253,
-1.35287912427843));
#69236=CARTESIAN_POINT('Ctrl Pts',(-0.604500991199494,0.435471696224031,
-1.3370370108502));
#69237=CARTESIAN_POINT('Ctrl Pts',(-0.739060921642629,0.0940531800321082,
-1.32119489742196));
#69238=CARTESIAN_POINT('Ctrl Pts',(-0.694303183903219,-0.270185372282176,
-1.30535278399373));
#69239=CARTESIAN_POINT('Ctrl Pts',(-0.481087306512033,-0.56886909749643,
-1.28951067056549));
#69240=CARTESIAN_POINT('Ctrl Pts',(-0.151145660689984,-0.729528639484422,
-1.27366855713725));
#69241=CARTESIAN_POINT('Ctrl Pts',(0.215468317056472,-0.713183322097661,
-1.25782644370902));
#69242=CARTESIAN_POINT('Ctrl Pts',(0.529803416228333,-0.523798994583028,
-1.24198433028078));
#69243=CARTESIAN_POINT('Ctrl Pts',(0.715592802305182,-0.207325801246306,
-1.22614221685255));
#69244=CARTESIAN_POINT('Ctrl Pts',(0.727758568298884,0.159450659581461,
-1.21030010342431));
#69245=CARTESIAN_POINT('Ctrl Pts',(0.563348945653209,0.487539754281456,
-1.19445798999608));
#69246=CARTESIAN_POINT('Ctrl Pts',(0.262254489119811,0.69733752911335,-1.17861587656784));
#69247=CARTESIAN_POINT('Ctrl Pts',(-0.102470531663754,0.737940943920278,
-1.16277376313961));
#69248=CARTESIAN_POINT('Ctrl Pts',(-0.442333222080111,0.599498429704058,
-1.14693164971137));
#69249=CARTESIAN_POINT('Ctrl Pts',(-0.674873011744545,0.315600165703775,
-1.13108953628314));
#69250=CARTESIAN_POINT('Ctrl Pts',(-0.743668986465564,-0.0448718747400542,
-1.1152474228549));
#69251=CARTESIAN_POINT('Ctrl Pts',(-0.632029242496039,-0.394456693698165,
-1.09940530942667));
#69252=CARTESIAN_POINT('Ctrl Pts',(-0.367040827708315,-0.64833484972551,
-1.08356319599843));
#69253=CARTESIAN_POINT('Ctrl Pts',(-0.0129976362099471,-0.744908120526524,
-1.0677210825702));
#69254=CARTESIAN_POINT('Ctrl Pts',(0.344199159746186,-0.66074502268532,
-1.05187896914196));
#69255=CARTESIAN_POINT('Ctrl Pts',(0.617883231773016,-0.416265970825311,
-1.03603685571372));
#69256=CARTESIAN_POINT('Ctrl Pts',(0.741650866485886,-0.07078869128708,
-1.02019474228549));
#69257=CARTESIAN_POINT('Ctrl Pts',(0.685472437093205,0.291863982976498,
-1.00435262885725));
#69258=CARTESIAN_POINT('Ctrl Pts',(0.462978463983554,0.583701968868388,
-0.988510515429021));
#69259=CARTESIAN_POINT('Ctrl Pts',(0.128152454164742,0.733916885665508,
-0.972668402000784));
#69260=CARTESIAN_POINT('Ctrl Pts',(-0.237767067135667,0.706062226973733,
-0.956826288572548));
#69261=CARTESIAN_POINT('Ctrl Pts',(-0.545997384744169,0.506896342880804,
-0.940984175144315));
#69262=CARTESIAN_POINT('Ctrl Pts',(-0.721752861647405,0.184742667722392,
-0.925142061716078));
#69263=CARTESIAN_POINT('Ctrl Pts',(-0.72239010896405,-0.182234950117461,
-0.909299948287843));
#69264=CARTESIAN_POINT('Ctrl Pts',(-0.547754511966775,-0.504997070480062,
-0.893457834859609));
#69265=CARTESIAN_POINT('Ctrl Pts',(-0.240217744110618,-0.705232218483962,
-0.877615721431371));
#69266=CARTESIAN_POINT('Ctrl Pts',(0.125602832926312,-0.734357525279266,
-0.861773608003138));
#69267=CARTESIAN_POINT('Ctrl Pts',(0.460948510725695,-0.585306344603549,
-0.845931494574901));
#69268=CARTESIAN_POINT('Ctrl Pts',(0.684454677498251,-0.294242826631626,
-0.830089381146668));
#69269=CARTESIAN_POINT('Ctrl Pts',(0.741892238623479,0.068212556348874,
-0.814247267718431));
#69270=CARTESIAN_POINT('Ctrl Pts',(0.619325171744547,0.414117589842537,
-0.798405154290196));
#69271=CARTESIAN_POINT('Ctrl Pts',(0.346491810989388,0.659545655349725,
-0.782563040861961));
#69272=CARTESIAN_POINT('Ctrl Pts',(-0.0104105375467384,0.744948768225972,
-0.766720927433726));
#69273=CARTESIAN_POINT('Ctrl Pts',(-0.364786986982069,0.649605650146261,
-0.75087881400549));
#69274=CARTESIAN_POINT('Ctrl Pts',(-0.630655506998571,0.396649313708947,
-0.735036700577256));
#69275=CARTESIAN_POINT('Ctrl Pts',(-0.743508664370658,0.047454320974652,
-0.719194587149019));
#69276=CARTESIAN_POINT('Ctrl Pts',(-0.675965001853878,-0.31325446978789,
-0.703352473720785));
#69277=CARTESIAN_POINT('Ctrl Pts',(-0.444412575842957,-0.597958618138441,
-0.687510360292549));
#69278=CARTESIAN_POINT('Ctrl Pts',(-0.105032737398919,-0.737580619761592,
-0.671668246864314));
#69279=CARTESIAN_POINT('Ctrl Pts',(0.259831097021177,-0.698244117479107,
-0.655826133436078));
#69280=CARTESIAN_POINT('Ctrl Pts',(0.561652352575658,-0.489493290474582,
-0.639984020007844));
#69281=CARTESIAN_POINT('Ctrl Pts',(0.727200417052382,-0.161977158921392,
-0.624141906579607));
#69282=CARTESIAN_POINT('Ctrl Pts',(0.716308516610675,0.204839340958754,
-0.608299793151373));
#69283=CARTESIAN_POINT('Ctrl Pts',(0.531619342985543,0.521955860908782,
-0.592457679723137));
#69284=CARTESIAN_POINT('Ctrl Pts',(0.217943859635038,0.712430712856194,
-0.576615566294903));
#69285=CARTESIAN_POINT('Ctrl Pts',(-0.148611140897316,0.730049159560228,
-0.560773452866666));
#69286=CARTESIAN_POINT('Ctrl Pts',(-0.479108757699555,0.57053645358472,
-0.544931339438432));
#69287=CARTESIAN_POINT('Ctrl Pts',(-0.693360659540056,0.272595015316652,
-0.529089226010196));
#69288=CARTESIAN_POINT('Ctrl Pts',(-0.739383105543975,-0.0914858995132521,
-0.513247112581961));
#69289=CARTESIAN_POINT('Ctrl Pts',(-0.606009712182644,-0.433369675119762,
-0.497404999153725));
#69290=CARTESIAN_POINT('Ctrl Pts',(-0.325600742590041,-0.670105367086779,
-0.481562885725491));
#69291=CARTESIAN_POINT('Ctrl Pts',(0.0338084341730408,-0.744254013326329,
-0.465720772297255));
#69292=CARTESIAN_POINT('Ctrl Pts',(0.385014701803114,-0.637824996348643,
-0.44987865886902));
#69293=CARTESIAN_POINT('Ctrl Pts',(0.642805208275577,-0.376641090154065,
-0.434036545440785));
#69294=CARTESIAN_POINT('Ctrl Pts',(0.744632481298183,-0.024073104445561,
-0.418194432012549));
#69295=CARTESIAN_POINT('Ctrl Pts',(0.665790263802216,0.334335716337538,
-0.402352318584314));
#69296=CARTESIAN_POINT('Ctrl Pts',(0.425407970035668,0.611624971351682,
-0.386510205156079));
#69297=CARTESIAN_POINT('Ctrl Pts',(0.0818093338989499,0.740516224983506,
-0.370668091727843));
#69298=CARTESIAN_POINT('Ctrl Pts',(-0.281638625537042,0.689736711545923,
-0.354825978299609));
#69299=CARTESIAN_POINT('Ctrl Pts',(-0.576752865142938,0.471607017389029,
-0.338983864871373));
#69300=CARTESIAN_POINT('Ctrl Pts',(-0.731930091210175,0.139051748653782,
-0.323141751443138));
#69301=CARTESIAN_POINT('Ctrl Pts',(-0.709519794040012,-0.227241517439931,
-0.307299638014902));
#69302=CARTESIAN_POINT('Ctrl Pts',(-0.514959368797507,-0.538399383976947,
-0.291457524586667));
#69303=CARTESIAN_POINT('Ctrl Pts',(-0.195454820845694,-0.71892590621481,
-0.275615411158432));
#69304=CARTESIAN_POINT('Ctrl Pts',(0.171472735631759,-0.725020099460598,
-0.259773297730196));
#69305=CARTESIAN_POINT('Ctrl Pts',(0.49679604817575,-0.555203338168894,
-0.243931184301961));
#69306=CARTESIAN_POINT('Ctrl Pts',(0.70158214109123,-0.25067810039921,-0.228089070873726));
#69307=CARTESIAN_POINT('Ctrl Pts',(0.736144113092337,0.114668925666095,
-0.21224695744549));
#69308=CARTESIAN_POINT('Ctrl Pts',(0.59209591274996,0.45219395093952,-0.196404844017255));
#69309=CARTESIAN_POINT('Ctrl Pts',(0.30438843395392,0.680003547227091,-0.18056273058902));
#69310=CARTESIAN_POINT('Ctrl Pts',(-0.0571733245314984,0.742824567798009,
-0.164720617160785));
#69311=CARTESIAN_POINT('Ctrl Pts',(-0.404861612056579,0.625414639751036,
-0.148878503732549));
#69312=CARTESIAN_POINT('Ctrl Pts',(-0.654321761039958,0.356261152484546,
-0.133036390304314));
#69313=CARTESIAN_POINT('Ctrl Pts',(-0.745018423420191,0.000667926109236243,
-0.117194276876079));
#69314=CARTESIAN_POINT('Ctrl Pts',(-0.654963731198904,-0.355086524024519,
-0.101352163447843));
#69315=CARTESIAN_POINT('Ctrl Pts',(-0.405972665217733,-0.624688305282234,
-0.0855100500196082));
#69316=CARTESIAN_POINT('Ctrl Pts',(-0.0585265163337596,-0.742719209596254,
-0.0696679365913732));
#69317=CARTESIAN_POINT('Ctrl Pts',(0.303213024321455,-0.680552488980807,
-0.0538258231631377));
#69318=CARTESIAN_POINT('Ctrl Pts',(0.495177895946605,-0.529007593879737,
-0.0432644142109807));
#69319=CARTESIAN_POINT('Ctrl Pts',(0.567325265044103,-0.434889340047653,
-0.0379837097349022));
#69320=CARTESIAN_POINT('Ctrl Pts',(-0.325579286442198,0.678938089483055,
-2.9309162902651));
#69321=CARTESIAN_POINT('Ctrl Pts',(-0.438213909610741,0.624925064130741,
-2.92563558578902));
#69322=CARTESIAN_POINT('Ctrl Pts',(-0.635971822316887,0.459818132313165,
-2.91507417683686));
#69323=CARTESIAN_POINT('Ctrl Pts',(-0.778322195271528,0.100355400831034,
-2.89923206340863));
#69324=CARTESIAN_POINT('Ctrl Pts',(-0.731816705234331,-0.283358779024489,
-2.88338994998039));
#69325=CARTESIAN_POINT('Ctrl Pts',(-0.507757655804455,-0.598369701717211,
-2.86754783655216));
#69326=CARTESIAN_POINT('Ctrl Pts',(-0.160498528715463,-0.768174537150173,
-2.85170572312392));
#69327=CARTESIAN_POINT('Ctrl Pts',(0.225700520400454,-0.751610215820158,
-2.83586360969569));
#69328=CARTESIAN_POINT('Ctrl Pts',(0.557138921428952,-0.552677122681642,
-2.82002149626745));
#69329=CARTESIAN_POINT('Ctrl Pts',(0.753398782282915,-0.21965169170006,
-2.80417938283922));
#69330=CARTESIAN_POINT('Ctrl Pts',(0.766862416751649,0.166669258345032,
-2.78833726941098));
#69331=CARTESIAN_POINT('Ctrl Pts',(0.594262817950469,0.512550568213471,
-2.77249515598275));
#69332=CARTESIAN_POINT('Ctrl Pts',(0.277477839139527,0.734072631771401,
-2.7566530425545));
#69333=CARTESIAN_POINT('Ctrl Pts',(-0.106631360901428,0.777487115032269,
-2.74081092912628));
#69334=CARTESIAN_POINT('Ctrl Pts',(-0.464868677313834,0.632260728592397,
-2.72496881569804));
#69335=CARTESIAN_POINT('Ctrl Pts',(-0.710315344007488,0.333629449864264,
-2.70912670226981));
#69336=CARTESIAN_POINT('Ctrl Pts',(-0.783418851518672,-0.0459500051977844,
-2.69328458884157));
#69337=CARTESIAN_POINT('Ctrl Pts',(-0.666442169331009,-0.414380667588194,
-2.67744247541334));
#69338=CARTESIAN_POINT('Ctrl Pts',(-0.387767238679958,-0.682270524233312,
-2.6616003619851));
#69339=CARTESIAN_POINT('Ctrl Pts',(-0.0150087019054416,-0.784621718116017,
-2.64575824855686));
#69340=CARTESIAN_POINT('Ctrl Pts',(0.361391382602686,-0.696600867951191,
-2.62991613512863));
#69341=CARTESIAN_POINT('Ctrl Pts',(0.65010740990818,-0.439564394165159,
-2.61407402170039));
#69342=CARTESIAN_POINT('Ctrl Pts',(0.781088477417849,-0.0758768172813364,
-2.59823190827216));
#69343=CARTESIAN_POINT('Ctrl Pts',(0.722554769705059,0.306220681377498,
-2.58238979484392));
#69344=CARTESIAN_POINT('Ctrl Pts',(0.488708266212908,0.614020139334652,
-2.56654768141569));
#69345=CARTESIAN_POINT('Ctrl Pts',(0.136286927873838,0.772840458458201,
-2.55070556798745));
#69346=CARTESIAN_POINT('Ctrl Pts',(-0.249201581778172,0.74414721164362,
-2.53486345455922));
#69347=CARTESIAN_POINT('Ctrl Pts',(-0.574226542023743,0.534902214788316,
-2.51902134113098));
#69348=CARTESIAN_POINT('Ctrl Pts',(-0.75992744722895,0.195874388065881,
-2.50317922770274));
#69349=CARTESIAN_POINT('Ctrl Pts',(-0.761247858439583,-0.190678260358557,
-2.48733711427451));
#69350=CARTESIAN_POINT('Ctrl Pts',(-0.577867405503348,-0.530966818745191,
-2.47149500084628));
#69351=CARTESIAN_POINT('Ctrl Pts',(-0.254279518187912,-0.74242738876084,
-2.45565288741804));
#69352=CARTESIAN_POINT('Ctrl Pts',(0.131003973553142,-0.773753487788634,
-2.43981077398981));
#69353=CARTESIAN_POINT('Ctrl Pts',(0.484502092299483,-0.617344493382228,
-2.42396866056157));
#69354=CARTESIAN_POINT('Ctrl Pts',(0.720445916296219,-0.311149775259424,
-2.40812654713334));
#69355=CARTESIAN_POINT('Ctrl Pts',(0.781588613648687,0.0705389251875665,
-2.3922844337051));
#69356=CARTESIAN_POINT('Ctrl Pts',(0.653095188222527,0.435112831427073,
-2.37644232027686));
#69357=CARTESIAN_POINT('Ctrl Pts',(0.366141881041268,0.694115713623784,
-2.36060020684863));
#69358=CARTESIAN_POINT('Ctrl Pts',(-0.00964809225185164,0.784705941909324,
-2.34475809342039));
#69359=CARTESIAN_POINT('Ctrl Pts',(-0.383097157841225,0.684903692942206,
-2.32891597999216));
#69360=CARTESIAN_POINT('Ctrl Pts',(-0.663595714183315,0.418923894125693,
-2.31307386656392));
#69361=CARTESIAN_POINT('Ctrl Pts',(-0.783086655863804,0.0513009781577409,
-2.29723175313568));
#69362=CARTESIAN_POINT('Ctrl Pts',(-0.712578006167895,-0.328769046714688,
-2.28138963970745));
#69363=CARTESIAN_POINT('Ctrl Pts',(-0.469177213588559,-0.629070141718054,
-2.26554752627922));
#69364=CARTESIAN_POINT('Ctrl Pts',(-0.111940387413922,-0.776740529789401,
-2.24970541285098));
#69365=CARTESIAN_POINT('Ctrl Pts',(0.272456431474037,-0.73595108118701,
-2.23386329942275));
#69366=CARTESIAN_POINT('Ctrl Pts',(0.590747398269758,-0.516598502116886,
-2.21802118599451));
#69367=CARTESIAN_POINT('Ctrl Pts',(0.7657058699483,-0.17190410605513,-2.20217907256628));
#69368=CARTESIAN_POINT('Ctrl Pts',(0.754881834269203,0.214499224339534,
-2.18633695913804));
#69369=CARTESIAN_POINT('Ctrl Pts',(0.560901517002844,0.548858806229622,
-2.17049484570981));
#69370=CARTESIAN_POINT('Ctrl Pts',(0.230830183199643,0.75004928336471,-2.15465273228157));
#69371=CARTESIAN_POINT('Ctrl Pts',(-0.155247264558969,0.769255996270977,
-2.13881061885334));
#69372=CARTESIAN_POINT('Ctrl Pts',(-0.503657212038229,0.601818837951901,
-2.1229685054251));
#69373=CARTESIAN_POINT('Ctrl Pts',(-0.729865275773881,0.288362931340722,
-2.10712639199686));
#69374=CARTESIAN_POINT('Ctrl Pts',(-0.778986802383074,-0.0950582067203571,
-2.09128427856863));
#69375=CARTESIAN_POINT('Ctrl Pts',(-0.639103481275727,-0.455415459962816,
-2.07544216514039));
#69376=CARTESIAN_POINT('Ctrl Pts',(-0.344155073334948,-0.705275681169934,
-2.05960005171216));
#69377=CARTESIAN_POINT('Ctrl Pts',(0.0342953618899345,-0.784015515857139,
-2.04375793828392));
#69378=CARTESIAN_POINT('Ctrl Pts',(0.404424745164305,-0.672530390726459,
-2.02791582485569));
#69379=CARTESIAN_POINT('Ctrl Pts',(0.67642892639579,-0.39786983862431,-2.01207371142745));
#69380=CARTESIAN_POINT('Ctrl Pts',(0.784311782550415,-0.0266744953932996,
-1.99623159799922));
#69381=CARTESIAN_POINT('Ctrl Pts',(0.701897795973256,0.350992855995365,
-1.98038948457098));
#69382=CARTESIAN_POINT('Ctrl Pts',(0.449182996038718,0.64349913521432,-1.96454737114274));
#69383=CARTESIAN_POINT('Ctrl Pts',(0.087483341029052,0.779873814148348,
-1.94870525771451));
#69384=CARTESIAN_POINT('Ctrl Pts',(-0.295442316139248,0.727028430521238,
-1.93286314428627));
#69385=CARTESIAN_POINT('Ctrl Pts',(-0.606685077268622,0.497784810908752,
-1.91702103085804));
#69386=CARTESIAN_POINT('Ctrl Pts',(-0.770728398959144,0.147764122809877,
-1.90117891742981));
#69387=CARTESIAN_POINT('Ctrl Pts',(-0.747770601721272,-0.238108437803669,
-1.88533680400157));
#69388=CARTESIAN_POINT('Ctrl Pts',(-0.543381914675166,-0.566208968275712,
-1.86949469057333));
#69389=CARTESIAN_POINT('Ctrl Pts',(-0.207152976008731,-0.75693074021513,
-1.8536525771451));
#69390=CARTESIAN_POINT('Ctrl Pts',(0.179337297721125,-0.763999106411768,
-1.83781046371686));
#69391=CARTESIAN_POINT('Ctrl Pts',(0.522315128695877,-0.585699075709795,
-1.82196835028863));
#69392=CARTESIAN_POINT('Ctrl Pts',(0.738564122856956,-0.265291419726369,
-1.80612623686039));
#69393=CARTESIAN_POINT('Ctrl Pts',(0.775615986665582,0.119483648172757,
-1.79028412343216));
#69394=CARTESIAN_POINT('Ctrl Pts',(0.624480860659006,0.475268508974123,
-1.77444201000392));
#69395=CARTESIAN_POINT('Ctrl Pts',(0.321828520741137,0.715739410811971,
-1.75859989657569));
#69396=CARTESIAN_POINT('Ctrl Pts',(-0.0589087756450992,0.782551121080208,
-1.74275778314745));
#69397=CARTESIAN_POINT('Ctrl Pts',(-0.425353090255639,0.659493176281511,
-1.72691566971922));
#69398=CARTESIAN_POINT('Ctrl Pts',(-0.6885943778013,0.376423011799676,-1.71107355629098));
#69399=CARTESIAN_POINT('Ctrl Pts',(-0.784762648042105,0.00202167995460736,
-1.69523144286274));
#69400=CARTESIAN_POINT('Ctrl Pts',(-0.690524682473687,-0.372870170228878,
-1.67938932943451));
#69401=CARTESIAN_POINT('Ctrl Pts',(-0.428745351562249,-0.657292875714973,
-1.66354721600628));
#69402=CARTESIAN_POINT('Ctrl Pts',(-0.0629399323611319,-0.782237218410294,
-1.64770510257804));
#69403=CARTESIAN_POINT('Ctrl Pts',(0.318136544443031,-0.717388067953282,
-1.6318629891498));
#69404=CARTESIAN_POINT('Ctrl Pts',(0.622023845574929,-0.478479713768591,
-1.61602087572157));
#69405=CARTESIAN_POINT('Ctrl Pts',(0.774990076093966,-0.123478268969749,
-1.60017876229333));
#69406=CARTESIAN_POINT('Ctrl Pts',(0.739921180901159,0.261482594077944,
-1.5843366488651));
#69407=CARTESIAN_POINT('Ctrl Pts',(0.525325893617189,0.583000177055891,
-1.56849453543686));
#69408=CARTESIAN_POINT('Ctrl Pts',(0.183271270410032,0.763064966037748,
-1.55265242200863));
#69409=CARTESIAN_POINT('Ctrl Pts',(-0.203250291708922,0.757988007736359,
-1.53681030858039));
#69410=CARTESIAN_POINT('Ctrl Pts',(-0.540457423448226,0.569001119850921,
-1.52096819515216));
#69411=CARTESIAN_POINT('Ctrl Pts',(-0.74653387017,0.241958016277407,-1.50512608172392));
#69412=CARTESIAN_POINT('Ctrl Pts',(-0.771479494116511,-0.14379113710389,
-1.48928396829569));
#69413=CARTESIAN_POINT('Ctrl Pts',(-0.609241761610959,-0.494652379819475,
-1.47344185486745));
#69414=CARTESIAN_POINT('Ctrl Pts',(-0.29918426370814,-0.725496572908043,
-1.45759974143922));
#69415=CARTESIAN_POINT('Ctrl Pts',(0.0834640355129492,-0.780314203207778,
-1.44175762801098));
#69416=CARTESIAN_POINT('Ctrl Pts',(0.445861532957072,-0.645804919756011,
-1.42591551458274));
#69417=CARTESIAN_POINT('Ctrl Pts',(0.70008005884299,-0.354604585647581,
-1.41007340115451));
#69418=CARTESIAN_POINT('Ctrl Pts',(0.784438807251015,0.0226331312571616,
-1.39423128772627));
#69419=CARTESIAN_POINT('Ctrl Pts',(0.678469893041574,0.394379392448504,
-1.37838917429804));
#69420=CARTESIAN_POINT('Ctrl Pts',(0.407884455904809,0.670437746239824,
-1.3625470608698));
#69421=CARTESIAN_POINT('Ctrl Pts',(0.0383343903065725,0.78382840945689,
-1.34670494744157));
#69422=CARTESIAN_POINT('Ctrl Pts',(-0.340516712972966,0.707039510308996,
-1.33086283401333));
#69423=CARTESIAN_POINT('Ctrl Pts',(-0.636748560979497,0.458702268407773,
-1.3150207205851));
#69424=CARTESIAN_POINT('Ctrl Pts',(-0.778486694287029,0.0990705191767479,
-1.29917860715686));
#69425=CARTESIAN_POINT('Ctrl Pts',(-0.731341320643033,-0.28459861853495,
-1.28333649372863));
#69426=CARTESIAN_POINT('Ctrl Pts',(-0.506751278470523,-0.599215856532842,
-1.26749438030039));
#69427=CARTESIAN_POINT('Ctrl Pts',(-0.159208642076294,-0.768445905213971,
-1.25165226687216));
#69428=CARTESIAN_POINT('Ctrl Pts',(0.226962639962163,-0.751228634314016,
-1.23581015344392));
#69429=CARTESIAN_POINT('Ctrl Pts',(0.558066186485511,-0.551741454354678,
-1.21996804001569));
#69430=CARTESIAN_POINT('Ctrl Pts',(0.753766650094275,-0.218385755390668,
-1.20412592658745));
#69431=CARTESIAN_POINT('Ctrl Pts',(0.766581408221195,0.167956677513898,
-1.18828381315922));
#69432=CARTESIAN_POINT('Ctrl Pts',(0.593401227948724,0.513547937023258,
-1.17244169973098));
#69433=CARTESIAN_POINT('Ctrl Pts',(0.27624465631744,0.734537535329514,-1.15659958630275));
#69434=CARTESIAN_POINT('Ctrl Pts',(-0.10793690089776,0.777306970492665,
-1.14075747287451));
#69435=CARTESIAN_POINT('Ctrl Pts',(-0.465929827631969,0.631479133997901,
-1.12491535944628));
#69436=CARTESIAN_POINT('Ctrl Pts',(-0.710874631023432,0.33243609900129,
-1.10907324601804));
#69437=CARTESIAN_POINT('Ctrl Pts',(-0.783340579868063,-0.0472655993706233,
-1.09323113258981));
#69438=CARTESIAN_POINT('Ctrl Pts',(-0.665745327989884,-0.415499289062616,
-1.07738901916157));
#69439=CARTESIAN_POINT('Ctrl Pts',(-0.386620902639458,-0.682920770363698,
-1.06154690573333));
#69440=CARTESIAN_POINT('Ctrl Pts',(-0.0136910050989311,-0.784645816487464,
-1.0457047923051));
#69441=CARTESIAN_POINT('Ctrl Pts',(0.362560728351902,-0.695992973534098,
-1.02986267887686));
#69442=CARTESIAN_POINT('Ctrl Pts',(0.650844687457245,-0.438471998832969,
-1.01402056544863));
#69443=CARTESIAN_POINT('Ctrl Pts',(0.781214801727662,-0.0745649684068042,
-0.998178452020392));
#69444=CARTESIAN_POINT('Ctrl Pts',(0.722039490860267,0.307433691371231,
-0.982336338592158));
#69445=CARTESIAN_POINT('Ctrl Pts',(0.487676405825348,0.614839998823407,
-0.966494225163922));
#69446=CARTESIAN_POINT('Ctrl Pts',(0.134988845284561,0.773068245758832,
-0.950652111735687));
#69447=CARTESIAN_POINT('Ctrl Pts',(-0.250450933995221,0.743727658899963,
-0.934809998307451));
#69448=CARTESIAN_POINT('Ctrl Pts',(-0.575124034692748,0.533937117712032,
-0.918967884879216));
#69449=CARTESIAN_POINT('Ctrl Pts',(-0.760255322534541,0.194597907259556,
-0.90312577145098));
#69450=CARTESIAN_POINT('Ctrl Pts',(-0.760926564298854,-0.191956413532444,
-0.887283658022745));
#69451=CARTESIAN_POINT('Ctrl Pts',(-0.576974897216953,-0.531936527165962,
-0.871441544594511));
#69452=CARTESIAN_POINT('Ctrl Pts',(-0.253032344216126,-0.742853372969652,
-0.855599431166274));
#69453=CARTESIAN_POINT('Ctrl Pts',(0.132303212542429,-0.773532391631306,
-0.83975731773804));
#69454=CARTESIAN_POINT('Ctrl Pts',(0.485538163151441,-0.616529961214717,
-0.823915204309804));
#69455=CARTESIAN_POINT('Ctrl Pts',(0.720967438097831,-0.309939436268682,
-0.808073090881569));
#69456=CARTESIAN_POINT('Ctrl Pts',(0.781469050047366,0.0718514075712125,
-0.792230977453334));
#69457=CARTESIAN_POINT('Ctrl Pts',(0.652363548824324,0.43620901081618,-0.776388864025098));
#69458=CARTESIAN_POINT('Ctrl Pts',(0.364975682836995,0.694729625026577,
-0.760546750596864));
#69459=CARTESIAN_POINT('Ctrl Pts',(-0.0109658956700025,0.784688632569665,
-0.744704637168627));
#69460=CARTESIAN_POINT('Ctrl Pts',(-0.384246829048165,0.684259362609184,
-0.728862523740393));
#69461=CARTESIAN_POINT('Ctrl Pts',(-0.664298309516936,0.417808876072346,
-0.713020410312157));
#69462=CARTESIAN_POINT('Ctrl Pts',(-0.783171705267838,0.0499858081835622,
-0.697178296883922));
#69463=CARTESIAN_POINT('Ctrl Pts',(-0.712024874184065,-0.329965270134697,
-0.681336183455686));
#69464=CARTESIAN_POINT('Ctrl Pts',(-0.46812010611875,-0.629857180001361,
-0.665494070027452));
#69465=CARTESIAN_POINT('Ctrl Pts',(-0.110635789466275,-0.776927424564915,
-0.649651956599216));
#69466=CARTESIAN_POINT('Ctrl Pts',(0.27369198650554,-0.735492486348126,
-0.633809843170981));
#69467=CARTESIAN_POINT('Ctrl Pts',(0.591614128810049,-0.515605686105404,
-0.617967729742745));
#69468=CARTESIAN_POINT('Ctrl Pts',(0.76599348196765,-0.170617954902095,
-0.60212561631451));
#69469=CARTESIAN_POINT('Ctrl Pts',(0.75452054472924,0.215766652968861,-0.586283502886275));
#69470=CARTESIAN_POINT('Ctrl Pts',(0.559978985250664,0.549799997298597,
-0.570441389458039));
#69471=CARTESIAN_POINT('Ctrl Pts',(0.22957024226141,0.750435876554373,-0.554599276029805));
#69472=CARTESIAN_POINT('Ctrl Pts',(-0.156538916378148,0.768994192833109,
-0.538757162601569));
#69473=CARTESIAN_POINT('Ctrl Pts',(-0.50466718245163,0.600972159012604,
-0.522915049173334));
#69474=CARTESIAN_POINT('Ctrl Pts',(-0.730348516593625,0.287136805828302,
-0.507072935745098));
#69475=CARTESIAN_POINT('Ctrl Pts',(-0.778826065336109,-0.0963662851063081,
-0.491230822316863));
#69476=CARTESIAN_POINT('Ctrl Pts',(-0.638337765842564,-0.456488113372826,
-0.475388708888627));
#69477=CARTESIAN_POINT('Ctrl Pts',(-0.342970164344439,-0.705852652698681,
-0.459546595460393));
#69478=CARTESIAN_POINT('Ctrl Pts',(0.0356119710671365,-0.78395681543616,
-0.443704482032157));
#69479=CARTESIAN_POINT('Ctrl Pts',(0.405553606856166,-0.67185026078431,
-0.427862368603922));
#69480=CARTESIAN_POINT('Ctrl Pts',(0.677096145942502,-0.396733298460725,
-0.412020255175687));
#69481=CARTESIAN_POINT('Ctrl Pts',(0.784355473072728,-0.0253573026962391,
-0.396178141747451));
#69482=CARTESIAN_POINT('Ctrl Pts',(0.701307356914353,0.352171111977085,
-0.380336028319216));
#69483=CARTESIAN_POINT('Ctrl Pts',(0.448101685014491,0.644252575325862,
-0.364493914890981));
#69484=CARTESIAN_POINT('Ctrl Pts',(0.0861735156653512,0.780019631902653,
-0.348651801462745));
#69485=CARTESIAN_POINT('Ctrl Pts',(-0.296662854383594,0.726531246309671,
-0.33280968803451));
#69486=CARTESIAN_POINT('Ctrl Pts',(-0.607520189821113,0.496765256041073,
-0.316967574606275));
#69487=CARTESIAN_POINT('Ctrl Pts',(-0.770975464226936,0.146469571011442,
-0.30112546117804));
#69488=CARTESIAN_POINT('Ctrl Pts',(-0.747369672537648,-0.239363890764772,
-0.285283347749805));
#69489=CARTESIAN_POINT('Ctrl Pts',(-0.542430271940636,-0.567120712737478,
-0.269441234321568));
#69490=CARTESIAN_POINT('Ctrl Pts',(-0.205881508420772,-0.7572775609926,
-0.253599120893334));
#69491=CARTESIAN_POINT('Ctrl Pts',(0.180620080446991,-0.763696853658917,
-0.237757007465098));
#69492=CARTESIAN_POINT('Ctrl Pts',(0.523298015026439,-0.584821086775341,
-0.221914894036863));
#69493=CARTESIAN_POINT('Ctrl Pts',(0.739008579394253,-0.264050716247043,
-0.206072780608628));
#69494=CARTESIAN_POINT('Ctrl Pts',(0.775414286343801,0.120786027599504,
-0.190230667180393));
#69495=CARTESIAN_POINT('Ctrl Pts',(0.623681724089946,0.476316584647831,
-0.174388553752157));
#69496=CARTESIAN_POINT('Ctrl Pts',(0.320626268807888,0.7162788588628,-0.158546440323922));
#69497=CARTESIAN_POINT('Ctrl Pts',(-0.060223279451711,0.782451115037967,
-0.142704326895687));
#69498=CARTESIAN_POINT('Ctrl Pts',(-0.426459265784379,0.658777864179818,
-0.126862213467451));
#69499=CARTESIAN_POINT('Ctrl Pts',(-0.689227058061626,0.375266177359453,
-0.111020100039216));
#69500=CARTESIAN_POINT('Ctrl Pts',(-0.784762003573733,0.000703557140667915,
-0.0951779866109806));
#69501=CARTESIAN_POINT('Ctrl Pts',(-0.689903274611894,-0.374028887441819,
-0.0793358731827455));
#69502=CARTESIAN_POINT('Ctrl Pts',(-0.427629588929981,-0.65801278284077,
-0.0634937597545103));
#69503=CARTESIAN_POINT('Ctrl Pts',(-0.0616486583102524,-0.782340136422,
-0.0476516463262753));
#69504=CARTESIAN_POINT('Ctrl Pts',(0.319388156045572,-0.71685708433609,
-0.0318095328980398));
#69505=CARTESIAN_POINT('Ctrl Pts',(0.521593541223493,-0.557227910382347,
-0.0212481239458828));
#69506=CARTESIAN_POINT('Ctrl Pts',(0.597589667152306,-0.458088845993774,
-0.0159674194698044));
#69507=CARTESIAN_POINT('Ctrl Pts',(-0.342067962509744,0.713322310757509,
-2.9089));
#69508=CARTESIAN_POINT('Ctrl Pts',(-0.460406866917156,0.656573843331485,
-2.90361929552392));
#69509=CARTESIAN_POINT('Ctrl Pts',(-0.66818005485177,0.483105216441118,
-2.89305788657176));
#69510=CARTESIAN_POINT('Ctrl Pts',(-0.817739637008241,0.105437811674842,
-2.87721577314354));
#69511=CARTESIAN_POINT('Ctrl Pts',(-0.768878917407871,-0.297709234697778,
-2.86137365971529));
#69512=CARTESIAN_POINT('Ctrl Pts',(-0.533472594856222,-0.628673607988602,
-2.84553154628707));
#69513=CARTESIAN_POINT('Ctrl Pts',(-0.16862683527399,-0.807078059683254,
-2.82968943285882));
#69514=CARTESIAN_POINT('Ctrl Pts',(0.237130924373097,-0.78967485289565,
-2.81384731943059));
#69515=CARTESIAN_POINT('Ctrl Pts',(0.585354731164429,-0.580666968551218,
-2.79800520600235));
#69516=CARTESIAN_POINT('Ctrl Pts',(0.79155399973086,-0.230775758073293,
-2.78216309257412));
#69517=CARTESIAN_POINT('Ctrl Pts',(0.805699488103364,0.175110076068112,
-2.76632097914588));
#69518=CARTESIAN_POINT('Ctrl Pts',(0.624358734712405,0.538508240090762,
-2.75047886571765));
#69519=CARTESIAN_POINT('Ctrl Pts',(0.291530459794522,0.77124909335653,-2.73463675228941));
#69520=CARTESIAN_POINT('Ctrl Pts',(-0.112031612212736,0.816862264866122,
-2.71879463886118));
#69521=CARTESIAN_POINT('Ctrl Pts',(-0.488411541842896,0.664281016055754,
-2.70295252543294));
#69522=CARTESIAN_POINT('Ctrl Pts',(-0.746288638688284,0.350525819364675,
-2.68711041200471));
#69523=CARTESIAN_POINT('Ctrl Pts',(-0.823094408919947,-0.0482771027207467,
-2.67126829857647));
#69524=CARTESIAN_POINT('Ctrl Pts',(-0.700193545740531,-0.43536661135378,
-2.65542618514824));
#69525=CARTESIAN_POINT('Ctrl Pts',(-0.407405368789744,-0.716823513729212,
-2.63958407172));
#69526=CARTESIAN_POINT('Ctrl Pts',(-0.015768804388061,-0.824358193636169,
-2.62374195829176));
#69527=CARTESIAN_POINT('Ctrl Pts',(0.379693730723338,-0.731879605077058,
-2.60789984486353));
#69528=CARTESIAN_POINT('Ctrl Pts',(0.683031526820612,-0.461825745571817,
-2.59205773143529));
#69529=CARTESIAN_POINT('Ctrl Pts',(0.820646015076266,-0.0797195318313355,
-2.57621561800706));
#69530=CARTESIAN_POINT('Ctrl Pts',(0.759147919315163,0.32172895794998,-2.56037350457882));
#69531=CARTESIAN_POINT('Ctrl Pts',(0.513458465714772,0.645116648228309,
-2.54453139115059));
#69532=CARTESIAN_POINT('Ctrl Pts',(0.143189059242546,0.811980282464406,
-2.52868927772235));
#69533=CARTESIAN_POINT('Ctrl Pts',(-0.261822176295599,0.78183389144885,
-2.51284716429412));
#69534=CARTESIAN_POINT('Ctrl Pts',(-0.603307739246953,0.561991866110547,
-2.49700505086588));
#69535=CARTESIAN_POINT('Ctrl Pts',(-0.798413303160151,0.205794273848672,
-2.48116293743765));
#69536=CARTESIAN_POINT('Ctrl Pts',(-0.799800585433026,-0.200334992832333,
-2.46532082400941));
#69537=CARTESIAN_POINT('Ctrl Pts',(-0.607132991049227,-0.557857165402611,
-2.44947871058118));
#69538=CARTESIAN_POINT('Ctrl Pts',(-0.267157280320236,-0.780026969651644,
-2.43363659715294));
#69539=CARTESIAN_POINT('Ctrl Pts',(0.137638554355512,-0.812939551360736,
-2.41779448372471));
#69540=CARTESIAN_POINT('Ctrl Pts',(0.509039273829898,-0.64860936125727,
-2.40195237029647));
#69541=CARTESIAN_POINT('Ctrl Pts',(0.756932264883711,-0.326907681448137,
-2.38611025686824));
#69542=CARTESIAN_POINT('Ctrl Pts',(0.821171480265806,0.0741113068961196,
-2.37026814344));
#69543=CARTESIAN_POINT('Ctrl Pts',(0.686170618534919,0.457148737361488,
-2.35442603001176));
#69544=CARTESIAN_POINT('Ctrl Pts',(0.384684813969298,0.729268592298606,
-2.33858391658353));
#69545=CARTESIAN_POINT('Ctrl Pts',(-0.0101367113822268,0.824446682869273,
-2.32274180315529));
#69546=CARTESIAN_POINT('Ctrl Pts',(-0.402498775822114,0.719590036947071,
-2.30689968972706));
#69547=CARTESIAN_POINT('Ctrl Pts',(-0.697202934380121,0.440139925595871,
-2.29105757629882));
#69548=CARTESIAN_POINT('Ctrl Pts',(-0.822745389508861,0.0538990709910901,
-2.27521546287059));
#69549=CARTESIAN_POINT('Ctrl Pts',(-0.748665891379994,-0.345419265380477,
-2.25937334944235));
#69550=CARTESIAN_POINT('Ctrl Pts',(-0.492938280140658,-0.660928844720641,
-2.24353123601412));
#69551=CARTESIAN_POINT('Ctrl Pts',(-0.117609509694749,-0.816077869471505,
-2.22768912258588));
#69552=CARTESIAN_POINT('Ctrl Pts',(0.286254747362578,-0.77322267518754,
-2.21184700915765));
#69553=CARTESIAN_POINT('Ctrl Pts',(0.620665279699681,-0.542761178039759,
-2.19600489572941));
#69554=CARTESIAN_POINT('Ctrl Pts',(0.804484369006286,-0.180610038027646,
-2.18016278230118));
#69555=CARTESIAN_POINT('Ctrl Pts',(0.793112159578158,0.225362348543543,
-2.16432066887294));
#69556=CARTESIAN_POINT('Ctrl Pts',(0.589307880075637,0.576655276827108,
-2.14847855544471));
#69557=CARTESIAN_POINT('Ctrl Pts',(0.242520374424596,0.788034868391458,
-2.13263644201647));
#69558=CARTESIAN_POINT('Ctrl Pts',(-0.163109625471599,0.808214288348271,
-2.11679432858824));
#69559=CARTESIAN_POINT('Ctrl Pts',(-0.529164487728682,0.632297422688588,
-2.10095221516));
#69560=CARTESIAN_POINT('Ctrl Pts',(-0.766828659521958,0.302966817898509,
-2.08511010173177));
#69561=CARTESIAN_POINT('Ctrl Pts',(-0.818437902561313,-0.0998723458362106,
-2.06926798830353));
#69562=CARTESIAN_POINT('Ctrl Pts',(-0.671470313919026,-0.478479574629131,
-2.05342587487529));
#69563=CARTESIAN_POINT('Ctrl Pts',(-0.361584503761051,-0.740993746567179,
-2.03758376144706));
#69564=CARTESIAN_POINT('Ctrl Pts',(0.0360322202724218,-0.823721290798065,
-2.02174164801882));
#69565=CARTESIAN_POINT('Ctrl Pts',(0.424906480011704,-0.706590099743728,
-2.00589953459059));
#69566=CARTESIAN_POINT('Ctrl Pts',(0.710686073316714,-0.418019606006058,
-1.99005742116235));
#69567=CARTESIAN_POINT('Ctrl Pts',(0.824032561656957,-0.0280254017074349,
-1.97421530773412));
#69568=CARTESIAN_POINT('Ctrl Pts',(0.737444791351247,0.368768579898975,
-1.95837319430588));
#69569=CARTESIAN_POINT('Ctrl Pts',(0.471931473061532,0.676088581877968,
-1.94253108087765));
#69570=CARTESIAN_POINT('Ctrl Pts',(0.0919138577468047,0.819369836255821,
-1.92668896744941));
#69571=CARTESIAN_POINT('Ctrl Pts',(-0.310404731901931,0.76384814474127,
-1.91084685402118));
#69572=CARTESIAN_POINT('Ctrl Pts',(-0.637410108407462,0.522994684018659,
-1.89500474059294));
#69573=CARTESIAN_POINT('Ctrl Pts',(-0.809761259573127,0.155247506602632,
-1.87916262716471));
#69574=CARTESIAN_POINT('Ctrl Pts',(-0.78564078492412,-0.250167229819576,
-1.86332051373647));
#69575=CARTESIAN_POINT('Ctrl Pts',(-0.570901012926016,-0.594884122541389,
-1.84747840030824));
#69576=CARTESIAN_POINT('Ctrl Pts',(-0.217644055939408,-0.795264830560256,
-1.83163628688));
#69577=CARTESIAN_POINT('Ctrl Pts',(0.18841967713557,-0.802691167934417,
-1.81579417345177));
#69578=CARTESIAN_POINT('Ctrl Pts',(0.548767318134455,-0.615361289292159,
-1.79995206002353));
#69579=CARTESIAN_POINT('Ctrl Pts',(0.775968052050294,-0.278726869908628,
-1.78410994659529));
#69580=CARTESIAN_POINT('Ctrl Pts',(0.81489637485211,0.12553479224773,-1.76826783316706));
#69581=CARTESIAN_POINT('Ctrl Pts',(0.656107143566346,0.499338063813484,
-1.75242571973882));
#69582=CARTESIAN_POINT('Ctrl Pts',(0.338127242584864,0.751987402576497,
-1.73658360631059));
#69583=CARTESIAN_POINT('Ctrl Pts',(-0.0618921586783426,0.822182733038054,
-1.72074149288235));
#69584=CARTESIAN_POINT('Ctrl Pts',(-0.446894722698526,0.692892627061363,
-1.70489937945412));
#69585=CARTESIAN_POINT('Ctrl Pts',(-0.72346763328869,0.395486623535428,
-1.68905726602588));
#69586=CARTESIAN_POINT('Ctrl Pts',(-0.82450626083418,0.00212406615444509,
-1.67321515259765));
#69587=CARTESIAN_POINT('Ctrl Pts',(-0.725495696540265,-0.391753851433967,
-1.65737303916941));
#69588=CARTESIAN_POINT('Ctrl Pts',(-0.450458782089819,-0.690580894211494,
-1.64153092574118));
#69589=CARTESIAN_POINT('Ctrl Pts',(-0.0661274697740855,-0.821852933044026,
-1.62568881231294));
#69590=CARTESIAN_POINT('Ctrl Pts',(0.334248289400433,-0.753719554505967,
-1.60984669888471));
#69591=CARTESIAN_POINT('Ctrl Pts',(0.653525695118409,-0.502711897245121,
-1.59400458545647));
#69592=CARTESIAN_POINT('Ctrl Pts',(0.814238765591132,-0.129731717095008,
-1.57816247202824));
#69593=CARTESIAN_POINT('Ctrl Pts',(0.777393837103336,0.274725149641497,
-1.5623203586));
#69594=CARTESIAN_POINT('Ctrl Pts',(0.551930560592181,0.612525707294143,
-1.54647824517177));
#69595=CARTESIAN_POINT('Ctrl Pts',(0.192552882404771,0.801709718844298,
-1.53063613174353));
#69596=CARTESIAN_POINT('Ctrl Pts',(-0.2135437236322,0.796375642463458,-1.51479401831529));
#69597=CARTESIAN_POINT('Ctrl Pts',(-0.567828413417889,0.597817680172738,
-1.49895190488706));
#69598=CARTESIAN_POINT('Ctrl Pts',(-0.784341420193217,0.254211766802947,
-1.48310979145882));
#69599=CARTESIAN_POINT('Ctrl Pts',(-0.810550393282888,-0.15107331253648,
-1.46726767803059));
#69600=CARTESIAN_POINT('Ctrl Pts',(-0.64009627377542,-0.519703613717099,
-1.45142556460236));
#69601=CARTESIAN_POINT('Ctrl Pts',(-0.314336187108121,-0.762238707549098,
-1.43558345117412));
#69602=CARTESIAN_POINT('Ctrl Pts',(0.0876909980445682,-0.819832528431104,
-1.41974133774588));
#69603=CARTESIAN_POINT('Ctrl Pts',(0.468441797408921,-0.678511140845962,
-1.40389922431765));
#69604=CARTESIAN_POINT('Ctrl Pts',(0.735534996525771,-0.372563222416845,
-1.38805711088941));
#69605=CARTESIAN_POINT('Ctrl Pts',(0.824166019411586,0.0237793662457898,
-1.37221499746118));
#69606=CARTESIAN_POINT('Ctrl Pts',(0.712830402919816,0.414352389259386,
-1.35637288403294));
#69607=CARTESIAN_POINT('Ctrl Pts',(0.428541404754035,0.704391475121063,
-1.34053077060471));
#69608=CARTESIAN_POINT('Ctrl Pts',(0.0402758017241118,0.823524708559051,
-1.32468865717647));
#69609=CARTESIAN_POINT('Ctrl Pts',(-0.357761881844586,0.742846903278738,
-1.30884654374824));
#69610=CARTESIAN_POINT('Ctrl Pts',(-0.668996130759501,0.481932840591515,
-1.29300443032));
#69611=CARTESIAN_POINT('Ctrl Pts',(-0.817912466931429,0.104087858321388,
-1.27716231689177));
#69612=CARTESIAN_POINT('Ctrl Pts',(-0.768379457382846,-0.299011864787725,
-1.26132020346353));
#69613=CARTESIAN_POINT('Ctrl Pts',(-0.532415250429014,-0.629562615569254,
-1.2454780900353));
#69614=CARTESIAN_POINT('Ctrl Pts',(-0.167271623462604,-0.807363170943519,
-1.22963597660706));
#69615=CARTESIAN_POINT('Ctrl Pts',(0.238456962867854,-0.789273946530371,
-1.21379386317883));
#69616=CARTESIAN_POINT('Ctrl Pts',(0.586328956742687,-0.57968391412633,
-1.19795174975059));
#69617=CARTESIAN_POINT('Ctrl Pts',(0.791940497883369,-0.22944570953503,
-1.18210963632235));
#69618=CARTESIAN_POINT('Ctrl Pts',(0.805404248143504,0.176462695446335,
-1.16626752289412));
#69619=CARTESIAN_POINT('Ctrl Pts',(0.62345351024424,0.539556119765059,-1.15042540946588));
#69620=CARTESIAN_POINT('Ctrl Pts',(0.290234823515067,0.771737541545678,
-1.13458329603765));
#69621=CARTESIAN_POINT('Ctrl Pts',(-0.113403270131766,0.81667299706505,
-1.11874118260941));
#69622=CARTESIAN_POINT('Ctrl Pts',(-0.489526433183827,0.663459838291745,
-1.10289906918118));
#69623=CARTESIAN_POINT('Ctrl Pts',(-0.746876250302318,0.349272032298804,
-1.08705695575294));
#69624=CARTESIAN_POINT('Ctrl Pts',(-0.823012173270564,-0.0496593240011921,
-1.07121484232471));
#69625=CARTESIAN_POINT('Ctrl Pts',(-0.699461413483729,-0.436541884427066,
-1.05537272889647));
#69626=CARTESIAN_POINT('Ctrl Pts',(-0.406200977570603,-0.717506691001887,
-1.03953061546824));
#69627=CARTESIAN_POINT('Ctrl Pts',(-0.0143843739879145,-0.824383512448402,
-1.02368850204));
#69628=CARTESIAN_POINT('Ctrl Pts',(0.380922296957617,-0.731240924382876,
-1.00784638861177));
#69629=CARTESIAN_POINT('Ctrl Pts',(0.683806143141474,-0.460678026840626,
-0.99200427518353));
#69630=CARTESIAN_POINT('Ctrl Pts',(0.820778736969435,-0.078341245526529,
-0.976162161755294));
#69631=CARTESIAN_POINT('Ctrl Pts',(0.758606544627331,0.323003399765964,
-0.96032004832706));
#69632=CARTESIAN_POINT('Ctrl Pts',(0.51237434766714,0.645978028778427,-0.944477934898824));
#69633=CARTESIAN_POINT('Ctrl Pts',(0.141825236404382,0.812219605852155,
-0.928635821470589));
#69634=CARTESIAN_POINT('Ctrl Pts',(-0.263134800854775,0.781393090826191,
-0.912793708042353));
#69635=CARTESIAN_POINT('Ctrl Pts',(-0.604250684641326,0.56097789254326,
-0.896951594614119));
#69636=CARTESIAN_POINT('Ctrl Pts',(-0.798757783421676,0.20445314679672,
-0.881109481185882));
#69637=CARTESIAN_POINT('Ctrl Pts',(-0.799463019633659,-0.201677876947427,
-0.865267367757648));
#69638=CARTESIAN_POINT('Ctrl Pts',(-0.606195282467129,-0.558875983851863,
-0.849425254329413));
#69639=CARTESIAN_POINT('Ctrl Pts',(-0.265846944321634,-0.780474527455342,
-0.833583140901176));
#69640=CARTESIAN_POINT('Ctrl Pts',(0.139003592158546,-0.812707257983346,
-0.817741027472943));
#69641=CARTESIAN_POINT('Ctrl Pts',(0.510127815577188,-0.647753577825886,
-0.801898914044706));
#69642=CARTESIAN_POINT('Ctrl Pts',(0.75748019869741,-0.325636045905737,
-0.786056800616472));
#69643=CARTESIAN_POINT('Ctrl Pts',(0.821045861471253,0.0754902587935505,
-0.770214687188235));
#69644=CARTESIAN_POINT('Ctrl Pts',(0.685401925904101,0.458300431789825,
-0.754372573760001));
#69645=CARTESIAN_POINT('Ctrl Pts',(0.383459554684601,0.729913594703426,
-0.738530460331766));
#69646=CARTESIAN_POINT('Ctrl Pts',(-0.0115212537932657,0.824428496913359,
-0.722688346903529));
#69647=CARTESIAN_POINT('Ctrl Pts',(-0.403706671114261,0.718913075072106,
-0.706846233475295));
#69648=CARTESIAN_POINT('Ctrl Pts',(-0.6979411120353,0.438968438435745,-0.691004120047059));
#69649=CARTESIAN_POINT('Ctrl Pts',(-0.822834746165019,0.0525172953924725,
-0.675162006618824));
#69650=CARTESIAN_POINT('Ctrl Pts',(-0.748084746514252,-0.346676070481504,
-0.659319893190589));
#69651=CARTESIAN_POINT('Ctrl Pts',(-0.491827636394545,-0.661755741864282,
-0.643477779762354));
#69652=CARTESIAN_POINT('Ctrl Pts',(-0.11623884153363,-0.816274229368237,
-0.627635666334118));
#69653=CARTESIAN_POINT('Ctrl Pts',(0.287552875989903,-0.772740855217146,
-0.611793552905883));
#69654=CARTESIAN_POINT('Ctrl Pts',(0.621575905044439,-0.541718081736226,
-0.595951439477648));
#69655=CARTESIAN_POINT('Ctrl Pts',(0.804786546882918,-0.179258750882796,
-0.580109326049412));
#69656=CARTESIAN_POINT('Ctrl Pts',(0.792732572847805,0.226693964978968,
-0.564267212621177));
#69657=CARTESIAN_POINT('Ctrl Pts',(0.588338627515784,0.577644133688412,
-0.548425099192942));
#69658=CARTESIAN_POINT('Ctrl Pts',(0.241196624887782,0.788441040252554,
-0.532582985764707));
#69659=CARTESIAN_POINT('Ctrl Pts',(-0.164466691858981,0.807939226105988,
-0.516740872336471));
#69660=CARTESIAN_POINT('Ctrl Pts',(-0.530225607203705,0.631407864440488,
-0.500898758908237));
#69661=CARTESIAN_POINT('Ctrl Pts',(-0.767336373647194,0.301678596339951,
-0.48505664548));
#69662=CARTESIAN_POINT('Ctrl Pts',(-0.818269025128244,-0.101246670699364,
-0.469214532051766));
#69663=CARTESIAN_POINT('Ctrl Pts',(-0.670665819502484,-0.479606551625889,
-0.453372418623529));
#69664=CARTESIAN_POINT('Ctrl Pts',(-0.360339586098838,-0.741599938310583,
-0.437530305195295));
#69665=CARTESIAN_POINT('Ctrl Pts',(0.0374155079612326,-0.823659617545991,
-0.42168819176706));
#69666=CARTESIAN_POINT('Ctrl Pts',(0.426092511909218,-0.705875525219977,
-0.405846078338824));
#69667=CARTESIAN_POINT('Ctrl Pts',(0.711387083609428,-0.416825506767385,
-0.390003964910589));
#69668=CARTESIAN_POINT('Ctrl Pts',(0.824078464847273,-0.0266415009469172,
-0.374161851482353));
#69669=CARTESIAN_POINT('Ctrl Pts',(0.73682445002649,0.370006507616631,-0.358319738054118));
#69670=CARTESIAN_POINT('Ctrl Pts',(0.470795399993314,0.676880179300043,
-0.342477624625883));
#69671=CARTESIAN_POINT('Ctrl Pts',(0.0905376974317523,0.8195230388218,-0.326635511197647));
#69672=CARTESIAN_POINT('Ctrl Pts',(-0.311687083230146,0.763325781073419,
-0.310793397769413));
#69673=CARTESIAN_POINT('Ctrl Pts',(-0.638287514499288,0.521923494693118,
-0.294951284341177));
#69674=CARTESIAN_POINT('Ctrl Pts',(-0.810020837243697,0.153887393369101,
-0.279109170912942));
#69675=CARTESIAN_POINT('Ctrl Pts',(-0.785219551035283,-0.251486264089612,
-0.263267057484706));
#69676=CARTESIAN_POINT('Ctrl Pts',(-0.569901175083765,-0.595842041498009,
-0.247424944056471));
#69677=CARTESIAN_POINT('Ctrl Pts',(-0.21630819599585,-0.79562921577039,
-0.231582830628236));
#69678=CARTESIAN_POINT('Ctrl Pts',(0.189767425262224,-0.802373607857236,
-0.2157407172));
#69679=CARTESIAN_POINT('Ctrl Pts',(0.549799981877126,-0.614438835381788,
-0.199898603771766));
#69680=CARTESIAN_POINT('Ctrl Pts',(0.776435017697278,-0.277423332094875,
-0.18405649034353));
#69681=CARTESIAN_POINT('Ctrl Pts',(0.814684459595264,0.126903129532913,
-0.168214376915295));
#69682=CARTESIAN_POINT('Ctrl Pts',(0.655267535429932,0.500439218356143,
-0.152372263487059));
#69683=CARTESIAN_POINT('Ctrl Pts',(0.336864103661856,0.752554170498509,
-0.136530150058825));
#69684=CARTESIAN_POINT('Ctrl Pts',(-0.0632732343719237,0.822077662277926,
-0.120688036630589));
#69685=CARTESIAN_POINT('Ctrl Pts',(-0.448056919512178,0.692141088608601,
-0.104845923202354));
#69686=CARTESIAN_POINT('Ctrl Pts',(-0.724132355083295,0.394271202234359,
-0.0890038097741183));
#69687=CARTESIAN_POINT('Ctrl Pts',(-0.824505583727274,0.000739188172099202,
-0.0731616963458828));
#69688=CARTESIAN_POINT('Ctrl Pts',(-0.724842818024885,-0.392971250859118,
-0.0573195829176476));
#69689=CARTESIAN_POINT('Ctrl Pts',(-0.449286512642228,-0.691337260399308,
-0.0414774694894125));
#69690=CARTESIAN_POINT('Ctrl Pts',(-0.0647708002867455,-0.821961063247746,
-0.0256353560611774));
#69691=CARTESIAN_POINT('Ctrl Pts',(0.335563287769688,-0.753161679691374,
-0.00979324263294204));
#69692=CARTESIAN_POINT('Ctrl Pts',(0.548009186500381,-0.585448226884957,
0.000768166319215033));
#69693=CARTESIAN_POINT('Ctrl Pts',(0.627854069260509,-0.481288351939895,
0.00604887079529348));
#69694=CARTESIAN_POINT('Ctrl Pts',(-0.79116656670867,1.93884184799344E-7,
-0.0731331508237035));
#69695=CARTESIAN_POINT('Ctrl Pts',(-0.791165138234783,-0.108770838987923,
-0.068755433882469));
#69696=CARTESIAN_POINT('Ctrl Pts',(-0.768256400998376,-0.217542593998915,
-0.0643777169412344));
#69697=CARTESIAN_POINT('Ctrl Pts',(-0.724732793080687,-0.317244732932517,
-0.0599999999999999));
#69698=CARTESIAN_POINT('',(-0.392913737924004,-0.550974480436018,-2.9089));
#69699=CARTESIAN_POINT('Ctrl Pts',(-0.392913737924002,-0.550974480436019,
-2.9089));
#69700=CARTESIAN_POINT('Ctrl Pts',(-0.409359766126388,-0.541179376730804,
-2.9089));
#69701=CARTESIAN_POINT('Ctrl Pts',(-0.425363363493956,-0.530696820512708,
-2.9089));
#69702=CARTESIAN_POINT('Ctrl Pts',(-0.440878330451655,-0.51955234426649,
-2.9089));
#69703=CARTESIAN_POINT('Ctrl Pts',(-0.464344956425318,-0.502696152664185,
-2.9089));
#69704=CARTESIAN_POINT('Ctrl Pts',(-0.486694654013419,-0.484326991024549,
-2.9089));
#69705=CARTESIAN_POINT('Ctrl Pts',(-0.507833441829143,-0.464597152324595,
-2.9089));
#69706=CARTESIAN_POINT('Ctrl Pts',(-0.515025378158515,-0.457884575191231,
-2.9089));
#69707=CARTESIAN_POINT('Ctrl Pts',(-0.522077024083522,-0.451014259706751,
-2.9089));
#69708=CARTESIAN_POINT('Ctrl Pts',(-0.528984244396564,-0.44399152039105,
-2.9089));
#69709=CARTESIAN_POINT('Ctrl Pts',(-0.534887861339321,-0.437989169093459,
-2.9089));
#69710=CARTESIAN_POINT('Ctrl Pts',(-0.540684793267629,-0.431876452002257,
-2.9089));
#69711=CARTESIAN_POINT('Ctrl Pts',(-0.546364587743398,-0.425665844041185,
-2.9089));
#69712=CARTESIAN_POINT('Ctrl Pts',(-0.569500373077027,-0.400367870110675,
-2.9089));
#69713=CARTESIAN_POINT('Ctrl Pts',(-0.590733194895916,-0.373411181702835,
-2.9089));
#69714=CARTESIAN_POINT('Ctrl Pts',(-0.609906853654402,-0.345037909562405,
-2.9089));
#69715=CARTESIAN_POINT('Ctrl Pts',(-0.61723018226465,-0.334200812780321,
-2.9089));
#69716=CARTESIAN_POINT('Ctrl Pts',(-0.624252776542584,-0.323156582520568,
-2.9089));
#69717=CARTESIAN_POINT('Ctrl Pts',(-0.630964508213922,-0.311917121560154,
-2.9089));
#69718=CARTESIAN_POINT('Ctrl Pts',(-0.635277847467634,-0.304694006792599,
-2.9089));
#69719=CARTESIAN_POINT('Ctrl Pts',(-0.639463497654007,-0.297388934158588,
-2.9089));
#69720=CARTESIAN_POINT('Ctrl Pts',(-0.643516328199236,-0.290008987870708,
-2.9089));
#69721=CARTESIAN_POINT('Ctrl Pts',(-0.649668223487523,-0.278806778380437,
-2.9089));
#69722=CARTESIAN_POINT('Ctrl Pts',(-0.655504229181834,-0.267450350249753,
-2.9089));
#69723=CARTESIAN_POINT('Ctrl Pts',(-0.661017337842235,-0.25595243742994,
-2.9089));
#69724=CARTESIAN_POINT('Ctrl Pts',(-0.67572645112639,-0.225275715345224,
-2.9089));
#69725=CARTESIAN_POINT('Ctrl Pts',(-0.688140193377098,-0.193594372368486,
-2.9089));
#69726=CARTESIAN_POINT('Ctrl Pts',(-0.698261510376344,-0.161185561047533,
-2.9089));
#69727=CARTESIAN_POINT('Ctrl Pts',(-0.705141449214773,-0.139155756059611,
-2.9089));
#69728=CARTESIAN_POINT('Ctrl Pts',(-0.710961336057706,-0.116788935860317,
-2.9089));
#69729=CARTESIAN_POINT('Ctrl Pts',(-0.715710431828713,-0.0941649192640481,
-2.9089));
#69730=CARTESIAN_POINT('Ctrl Pts',(-0.719357292099036,-0.0767917957773035,
-2.9089));
#69731=CARTESIAN_POINT('Ctrl Pts',(-0.722372543094714,-0.0592668759475071,
-2.9089));
#69732=CARTESIAN_POINT('Ctrl Pts',(-0.72474721180396,-0.041625047399535,
-2.9089));
#69733=CARTESIAN_POINT('Ctrl Pts',(-0.726025787999834,-0.0321262815526122,
-2.9089));
#69734=CARTESIAN_POINT('Ctrl Pts',(-0.727118789016985,-0.0225894136711933,
-2.9089));
#69735=CARTESIAN_POINT('Ctrl Pts',(-0.728022317948154,-0.0130479136047751,
-2.9089));
#69736=CARTESIAN_POINT('Ctrl Pts',(-0.731403409697682,0.0226572929910528,
-2.9089));
#69737=CARTESIAN_POINT('Ctrl Pts',(-0.732147066811708,0.0584956871592241,
-2.9089));
#69738=CARTESIAN_POINT('Ctrl Pts',(-0.730236974451504,0.0941715601595828,
-2.9089));
#69739=CARTESIAN_POINT('Ctrl Pts',(-0.728572567971089,0.125258619326665,
-2.9089));
#69740=CARTESIAN_POINT('Ctrl Pts',(-0.72489265561043,0.156223354823441,
-2.9089));
#69741=CARTESIAN_POINT('Ctrl Pts',(-0.719274620967193,0.186892382374801,
-2.9089));
#69742=CARTESIAN_POINT('Ctrl Pts',(-0.71600434450303,0.204744924295439,
-2.9089));
#69743=CARTESIAN_POINT('Ctrl Pts',(-0.712076711511137,0.222497338567289,
-2.9089));
#69744=CARTESIAN_POINT('Ctrl Pts',(-0.707501869156712,0.240115064096392,
-2.9089));
#69745=CARTESIAN_POINT('Ctrl Pts',(-0.70486229707856,0.250280060567185,
-2.9089));
#69746=CARTESIAN_POINT('Ctrl Pts',(-0.702005320648755,0.260405624416952,
-2.9089));
#69747=CARTESIAN_POINT('Ctrl Pts',(-0.69894255661829,0.270453695927041,
-2.9089));
#69748=CARTESIAN_POINT('Ctrl Pts',(-0.688468965167679,0.304814617896998,
-2.9089));
#69749=CARTESIAN_POINT('Ctrl Pts',(-0.675580529064114,0.33832823878394,
-2.9089));
#69750=CARTESIAN_POINT('Ctrl Pts',(-0.660407686502252,0.370740116386383,
-2.9089));
#69751=CARTESIAN_POINT('Ctrl Pts',(-0.648075258027009,0.397084366690881,
-2.9089));
#69752=CARTESIAN_POINT('Ctrl Pts',(-0.634232555647159,0.422701237310616,
-2.9089));
#69753=CARTESIAN_POINT('Ctrl Pts',(-0.618924570005842,0.447450319236685,
-2.9089));
#69754=CARTESIAN_POINT('Ctrl Pts',(-0.610065535171487,0.461773103699558,
-2.9089));
#69755=CARTESIAN_POINT('Ctrl Pts',(-0.600715341027939,0.475805141443812,
-2.9089));
#69756=CARTESIAN_POINT('Ctrl Pts',(-0.590894184902779,0.489528828314774,
-2.9089));
#69757=CARTESIAN_POINT('Ctrl Pts',(-0.585545297999762,0.497003146819615,
-2.9089));
#69758=CARTESIAN_POINT('Ctrl Pts',(-0.580056674884228,0.504385979354654,
-2.9089));
#69759=CARTESIAN_POINT('Ctrl Pts',(-0.574431315468417,0.511674297783051,
-2.9089));
#69760=CARTESIAN_POINT('Ctrl Pts',(-0.569921668564276,0.517517078698459,
-2.9089));
#69761=CARTESIAN_POINT('Ctrl Pts',(-0.565324592131169,0.523298328689192,
-2.9089));
#69762=CARTESIAN_POINT('Ctrl Pts',(-0.560650192799266,0.529006583378885,
-2.9089));
#69763=CARTESIAN_POINT('Ctrl Pts',(-0.537633044250205,0.557114525559133,
-2.9089));
#69764=CARTESIAN_POINT('Ctrl Pts',(-0.512694828279584,0.583520233685232,
-2.9089));
#69765=CARTESIAN_POINT('Ctrl Pts',(-0.486073668914314,0.608074069631979,
-2.9089));
#69766=CARTESIAN_POINT('Ctrl Pts',(-0.45923537508389,0.632828177999722,
-2.9089));
#69767=CARTESIAN_POINT('Ctrl Pts',(-0.43068580735773,0.655701030012639,
-2.9089));
#69768=CARTESIAN_POINT('Ctrl Pts',(-0.400624822626115,0.676511476791734,
-2.9089));
#69769=CARTESIAN_POINT('Ctrl Pts',(-0.381691858478924,0.689618281052249,
-2.9089));
#69770=CARTESIAN_POINT('Ctrl Pts',(-0.362158516231663,0.701906388619064,
-2.9089));
#69771=CARTESIAN_POINT('Ctrl Pts',(-0.342067962509744,0.713322310757509,
-2.9089));
#69772=CARTESIAN_POINT('Ctrl Pts',(-0.392913737924004,-0.550974480436018,
-2.9089));
#69773=CARTESIAN_POINT('Ctrl Pts',(-0.316929799842835,-0.605044757612097,
-2.90451276788471));
#69774=CARTESIAN_POINT('Ctrl Pts',(-0.124667012097903,-0.689527912099726,
-2.89484483129333));
#69775=CARTESIAN_POINT('Ctrl Pts',(0.202839712455166,-0.675480941669175,
-2.87989619022589));
#69776=CARTESIAN_POINT('Ctrl Pts',(0.500707301958,-0.496697430942489,-2.86405407679764));
#69777=CARTESIAN_POINT('Ctrl Pts',(0.677088347387025,-0.197403558953597,
-2.84821196336941));
#69778=CARTESIAN_POINT('Ctrl Pts',(0.689188274048217,0.149787622898873,
-2.83236984994118));
#69779=CARTESIAN_POINT('Ctrl Pts',(0.534070984426596,0.460635224458885,
-2.81652773651294));
#69780=CARTESIAN_POINT('Ctrl Pts',(0.249372597829536,0.659719708601146,
-2.80068562308471));
#69781=CARTESIAN_POINT('Ctrl Pts',(-0.095830858278809,0.69873681536456,
-2.78484350965647));
#69782=CARTESIAN_POINT('Ctrl Pts',(-0.417782948255712,0.568220153665686,
-2.76900139622824));
#69783=CARTESIAN_POINT('Ctrl Pts',(-0.629713345155285,0.31036761779697,
-2.75378090021574));
#69784=CARTESIAN_POINT('Ctrl Pts',(-0.676654539125682,0.099017931234991,
-2.74384110867933));
#69785=CARTESIAN_POINT('Ctrl Pts',(-0.676738003850817,-1.23232206217291E-5,
-2.739182021619));
#69786=CARTESIAN_POINT('Origin',(-1.87869726832665E-16,-4.25270154953079E-17,
-2.9089));
#69787=CARTESIAN_POINT('',(-0.7911,-9.68818082805471E-17,-2.9089));
#69788=CARTESIAN_POINT('Origin',(0.,0.,-2.9089));
#69789=CARTESIAN_POINT('Origin',(0.,0.,-2.9089));
#69790=CARTESIAN_POINT('',(0.392888236737279,-0.550964357679762,-2.9089));
#69791=CARTESIAN_POINT('Ctrl Pts',(0.342095308501471,0.713339076749545,
-2.9089));
#69792=CARTESIAN_POINT('Ctrl Pts',(0.361421457667255,0.702382391769599,
-2.9089));
#69793=CARTESIAN_POINT('Ctrl Pts',(0.380253116542679,0.690624130244962,
-2.9089));
#69794=CARTESIAN_POINT('Ctrl Pts',(0.398533666067781,0.67808073602098,-2.9089));
#69795=CARTESIAN_POINT('Ctrl Pts',(0.425013708871964,0.659911171943888,
-2.9089));
#69796=CARTESIAN_POINT('Ctrl Pts',(0.450338555601534,0.640094850049735,
-2.9089));
#69797=CARTESIAN_POINT('Ctrl Pts',(0.474378541812238,0.618766150097485,
-2.9089));
#69798=CARTESIAN_POINT('Ctrl Pts',(0.484755880862577,0.609559191783637,
-2.9089));
#69799=CARTESIAN_POINT('Ctrl Pts',(0.494893503862243,0.600070177957475,
-2.9089));
#69800=CARTESIAN_POINT('Ctrl Pts',(0.504779505517662,0.590308982482977,
-2.9089));
#69801=CARTESIAN_POINT('Ctrl Pts',(0.511746361070153,0.58343008024719,-2.9089));
#69802=CARTESIAN_POINT('Ctrl Pts',(0.518582035916023,0.576422022636668,
-2.9089));
#69803=CARTESIAN_POINT('Ctrl Pts',(0.525279345939323,0.56929274522698,-2.9089));
#69804=CARTESIAN_POINT('Ctrl Pts',(0.550202482175477,0.54276210060566,-2.9089));
#69805=CARTESIAN_POINT('Ctrl Pts',(0.573230055554725,0.514538002482786,
-2.9089));
#69806=CARTESIAN_POINT('Ctrl Pts',(0.594163530853824,0.484814447194274,
-2.9089));
#69807=CARTESIAN_POINT('Ctrl Pts',(0.601840751795605,0.473913519476122,
-2.9089));
#69808=CARTESIAN_POINT('Ctrl Pts',(0.609235863492435,0.462810666846166,
-2.9089));
#69809=CARTESIAN_POINT('Ctrl Pts',(0.61633739280612,0.451514753928317,-2.9089));
#69810=CARTESIAN_POINT('Ctrl Pts',(0.620979176071088,0.444131389412231,
-2.9089));
#69811=CARTESIAN_POINT('Ctrl Pts',(0.625495511580747,0.436665536531298,
-2.9089));
#69812=CARTESIAN_POINT('Ctrl Pts',(0.629882962628105,0.429119616277332,
-2.9089));
#69813=CARTESIAN_POINT('Ctrl Pts',(0.633948112087592,0.42212801835165,-2.9089));
#69814=CARTESIAN_POINT('Ctrl Pts',(0.637897862824706,0.415075813183006,
-2.9089));
#69815=CARTESIAN_POINT('Ctrl Pts',(0.641729261349816,0.407967103368741,
-2.9089));
#69816=CARTESIAN_POINT('Ctrl Pts',(0.64468657514332,0.402480155078196,-2.9089));
#69817=CARTESIAN_POINT('Ctrl Pts',(0.647573584485386,0.396959182713758,
-2.9089));
#69818=CARTESIAN_POINT('Ctrl Pts',(0.650389374318831,0.391405199216917,
-2.9089));
#69819=CARTESIAN_POINT('Ctrl Pts',(0.666501897875371,0.359624173210447,
-2.9089));
#69820=CARTESIAN_POINT('Ctrl Pts',(0.680286508535265,0.326763593217329,
-2.9089));
#69821=CARTESIAN_POINT('Ctrl Pts',(0.691692293406641,0.293090804439526,
-2.9089));
#69822=CARTESIAN_POINT('Ctrl Pts',(0.702996182480478,0.259718838069524,
-2.9089));
#69823=CARTESIAN_POINT('Ctrl Pts',(0.711963660398992,0.22554786022234,-2.9089));
#69824=CARTESIAN_POINT('Ctrl Pts',(0.718494894315197,0.190832889778513,
-2.9089));
#69825=CARTESIAN_POINT('Ctrl Pts',(0.720554421264328,0.17988604296754,-2.9089));
#69826=CARTESIAN_POINT('Ctrl Pts',(0.722371313086546,0.168885139159948,
-2.9089));
#69827=CARTESIAN_POINT('Ctrl Pts',(0.72394136251251,0.157838367402538,-2.9089));
#69828=CARTESIAN_POINT('Ctrl Pts',(0.724918609600457,0.150962516647377,
-2.9089));
#69829=CARTESIAN_POINT('Ctrl Pts',(0.725799613851594,0.144072570993966,
-2.9089));
#69830=CARTESIAN_POINT('Ctrl Pts',(0.726582863853827,0.137178847898393,
-2.9089));
#69831=CARTESIAN_POINT('Ctrl Pts',(0.730549180008782,0.102269578567019,
-2.9089));
#69832=CARTESIAN_POINT('Ctrl Pts',(0.732022348457187,0.0671998437829258,
-2.9089));
#69833=CARTESIAN_POINT('Ctrl Pts',(0.730931128253835,0.0322245814176823,
-2.9089));
#69834=CARTESIAN_POINT('Ctrl Pts',(0.730000903408154,0.00240946441705488,
-2.9089));
#69835=CARTESIAN_POINT('Ctrl Pts',(0.727206070274835,-0.0273375730699786,
-2.9089));
#69836=CARTESIAN_POINT('Ctrl Pts',(0.722582103198713,-0.0568465663805478,
-2.9089));
#69837=CARTESIAN_POINT('Ctrl Pts',(0.720073144499858,-0.0728581089028451,
-2.9089));
#69838=CARTESIAN_POINT('Ctrl Pts',(0.717025201034188,-0.0887994130225833,
-2.9089));
#69839=CARTESIAN_POINT('Ctrl Pts',(0.713440842181997,-0.104641669857954,
-2.9089));
#69840=CARTESIAN_POINT('Ctrl Pts',(0.711820150259532,-0.111804852660087,
-2.9089));
#69841=CARTESIAN_POINT('Ctrl Pts',(0.710089762375051,-0.118947765994846,
-2.9089));
#69842=CARTESIAN_POINT('Ctrl Pts',(0.708249780343376,-0.126067638780641,
-2.9089));
#69843=CARTESIAN_POINT('Ctrl Pts',(0.706460247497159,-0.132992296734754,
-2.9089));
#69844=CARTESIAN_POINT('Ctrl Pts',(0.704569208219147,-0.139886700115112,
-2.9089));
#69845=CARTESIAN_POINT('Ctrl Pts',(0.702578191106992,-0.146746082325932,
-2.9089));
#69846=CARTESIAN_POINT('Ctrl Pts',(0.693113370508214,-0.179353949755858,
-2.9089));
#69847=CARTESIAN_POINT('Ctrl Pts',(0.681388128385,-0.21119079851327,-2.9089));
#69848=CARTESIAN_POINT('Ctrl Pts',(0.667466886654037,-0.242007940169088,
-2.9089));
#69849=CARTESIAN_POINT('Ctrl Pts',(0.657168215657122,-0.264805877961715,
-2.9089));
#69850=CARTESIAN_POINT('Ctrl Pts',(0.64566666415709,-0.287045565613572,
-2.9089));
#69851=CARTESIAN_POINT('Ctrl Pts',(0.632973022387535,-0.308616041115058,
-2.9089));
#69852=CARTESIAN_POINT('Ctrl Pts',(0.624870735660704,-0.322384365487209,
-2.9089));
#69853=CARTESIAN_POINT('Ctrl Pts',(0.616282481939985,-0.335879827360128,
-2.9089));
#69854=CARTESIAN_POINT('Ctrl Pts',(0.607225187511364,-0.349079425631144,
-2.9089));
#69855=CARTESIAN_POINT('Ctrl Pts',(0.602385167740514,-0.356133001851115,
-2.9089));
#69856=CARTESIAN_POINT('Ctrl Pts',(0.597411183937436,-0.363102055610617,
-2.9089));
#69857=CARTESIAN_POINT('Ctrl Pts',(0.592305668509312,-0.369982813438398,
-2.9089));
#69858=CARTESIAN_POINT('Ctrl Pts',(0.58851755331426,-0.375088096861362,
-2.9089));
#69859=CARTESIAN_POINT('Ctrl Pts',(0.584658275650617,-0.380142949743923,
-2.9089));
#69860=CARTESIAN_POINT('Ctrl Pts',(0.580734572874794,-0.385139090101267,
-2.9089));
#69861=CARTESIAN_POINT('Ctrl Pts',(0.560140903620934,-0.411361479498082,
-2.9089));
#69862=CARTESIAN_POINT('Ctrl Pts',(0.537733933544869,-0.43602603165254,
-2.9089));
#69863=CARTESIAN_POINT('Ctrl Pts',(0.513699242000695,-0.458953879868942,
-2.9089));
#69864=CARTESIAN_POINT('Ctrl Pts',(0.490112295372544,-0.481454602675586,
-2.9089));
#69865=CARTESIAN_POINT('Ctrl Pts',(0.464956687258441,-0.502283358877662,
-2.9089));
#69866=CARTESIAN_POINT('Ctrl Pts',(0.43838137497774,-0.52122970548998,-2.9089));
#69867=CARTESIAN_POINT('Ctrl Pts',(0.423646031374266,-0.53173497912192,
-2.9089));
#69868=CARTESIAN_POINT('Ctrl Pts',(0.408473826265608,-0.541660727795806,
-2.9089));
#69869=CARTESIAN_POINT('Ctrl Pts',(0.392888236737283,-0.550964357679758,
-2.9089));
#69870=CARTESIAN_POINT('Origin',(0.,0.,-2.9089));
#69871=CARTESIAN_POINT('Origin',(0.,0.,-3.278617978381));
#69872=CARTESIAN_POINT('Ctrl Pts',(0.392888236737278,-0.550964357679762,
-2.9089));
#69873=CARTESIAN_POINT('Ctrl Pts',(0.484292245096581,-0.485784897022383,
-2.90361929552392));
#69874=CARTESIAN_POINT('Ctrl Pts',(0.633945837478465,-0.309125594940106,
-2.89305788657177));
#69875=CARTESIAN_POINT('Ctrl Pts',(0.704592787855342,0.0310787463577468,
-2.87721577314353));
#69876=CARTESIAN_POINT('Ctrl Pts',(0.604289094090405,0.363654317141465,
-2.8613736597153));
#69877=CARTESIAN_POINT('Ctrl Pts',(0.357365708044879,0.608039989146884,
-2.84553154628705));
#69878=CARTESIAN_POINT('Ctrl Pts',(0.0237357764082632,0.704875616667608,
-2.82968943285883));
#69879=CARTESIAN_POINT('Ctrl Pts',(-0.315653531008585,0.630699052042456,
-2.81384731943059));
#69880=CARTESIAN_POINT('Ctrl Pts',(-0.578455917520507,0.403490890783857,
-2.79800520600235));
#69881=CARTESIAN_POINT('Ctrl Pts',(-0.669224793849843,0.162504610084219,
-2.78626209231916));
#69882=CARTESIAN_POINT('Ctrl Pts',(-0.676728171233119,0.0251386911605121,
-2.77979968311204));
#69883=CARTESIAN_POINT('Ctrl Pts',(-0.676702457484846,1.74000875470086E-5,
-2.778617978381));
#69884=CARTESIAN_POINT('Ctrl Pts',(0.459308237155098,-0.644108029201217,
-2.97494887079529));
#69885=CARTESIAN_POINT('Ctrl Pts',(0.566164615185311,-0.567909608444529,
-2.96966816631922));
#69886=CARTESIAN_POINT('Ctrl Pts',(0.74111800211203,-0.361385042348344,
-2.95910675736706));
#69887=CARTESIAN_POINT('Ctrl Pts',(0.823708222953097,0.0363327859370564,
-2.94326464393882));
#69888=CARTESIAN_POINT('Ctrl Pts',(0.706447616868514,0.425132156480872,
-2.9274225305106));
#69889=CARTESIAN_POINT('Ctrl Pts',(0.417780422098877,0.710832622157672,
-2.91158041708234));
#69890=CARTESIAN_POINT('Ctrl Pts',(0.0277484449779586,0.824038865591465,
-2.89573830365413));
#69891=CARTESIAN_POINT('Ctrl Pts',(-0.369016563293757,0.737322329053924,
-2.87989619022588));
#69892=CARTESIAN_POINT('Ctrl Pts',(-0.676247194252207,0.471703330425765,
-2.86405407679765));
#69893=CARTESIAN_POINT('Ctrl Pts',(-0.819400710647197,0.0916387655639853,
-2.84821196336941));
#69894=CARTESIAN_POINT('Ctrl Pts',(-0.763743730503373,-0.310661748928857,
-2.83236984994118));
#69895=CARTESIAN_POINT('Ctrl Pts',(-0.522780345462078,-0.637585813690765,
-2.81652773651294));
#69896=CARTESIAN_POINT('Ctrl Pts',(-0.154975233012397,-0.80981346867949,
-2.80068562308471));
#69897=CARTESIAN_POINT('Ctrl Pts',(0.250431369065524,-0.785556602744988,
-2.78484350965647));
#69898=CARTESIAN_POINT('Ctrl Pts',(0.595076043601661,-0.570700980513612,
-2.76900139622823));
#69899=CARTESIAN_POINT('Ctrl Pts',(0.795337965757144,-0.217376647859616,
-2.7531592828));
#69900=CARTESIAN_POINT('Ctrl Pts',(0.802627773586437,0.188689549785515,
-2.73731716937176));
#69901=CARTESIAN_POINT('Ctrl Pts',(0.61517674617951,0.548974191752079,-2.72147505594353));
#69902=CARTESIAN_POINT('Ctrl Pts',(0.27846595382714,0.776061725259662,-2.7056329425153));
#69903=CARTESIAN_POINT('Ctrl Pts',(-0.125808775608511,0.814854123794499,
-2.68979082908706));
#69904=CARTESIAN_POINT('Ctrl Pts',(-0.499558638053648,0.65593921754596,
-2.67394871565883));
#69905=CARTESIAN_POINT('Ctrl Pts',(-0.752101050007928,0.33787438637163,
-2.65810660223059));
#69906=CARTESIAN_POINT('Ctrl Pts',(-0.822161879471254,-0.0621685953424848,
-2.64226448880235));
#69907=CARTESIAN_POINT('Ctrl Pts',(-0.692742332187273,-0.447127667972609,
-2.62642237537412));
#69908=CARTESIAN_POINT('Ctrl Pts',(-0.395243353255664,-0.723600568013129,
-2.61058026194588));
#69909=CARTESIAN_POINT('Ctrl Pts',(-0.00184684491450912,-0.824506931109911,
-2.59473814851765));
#69910=CARTESIAN_POINT('Ctrl Pts',(0.391997761702142,-0.725363939774458,
-2.57889603508941));
#69911=CARTESIAN_POINT('Ctrl Pts',(0.6907323137844,-0.450226566286644,-2.56305392166118));
#69912=CARTESIAN_POINT('Ctrl Pts',(0.821875123130991,-0.0658511372484234,
-2.54721180823294));
#69913=CARTESIAN_POINT('Ctrl Pts',(0.753607131146545,0.334501692348047,
-2.53136969480471));
#69914=CARTESIAN_POINT('Ctrl Pts',(0.502492137615154,0.653694685562662,
-2.51552758137647));
#69915=CARTESIAN_POINT('Ctrl Pts',(0.129457941270315,0.814282341537978,
-2.49968546794824));
#69916=CARTESIAN_POINT('Ctrl Pts',(-0.274986515685645,0.777301425760453,
-2.48384335452));
#69917=CARTESIAN_POINT('Ctrl Pts',(-0.612711248556089,0.551724583638581,
-2.46800124109177));
#69918=CARTESIAN_POINT('Ctrl Pts',(-0.801774417619176,0.192283315838124,
-2.45215912766353));
#69919=CARTESIAN_POINT('Ctrl Pts',(-0.796303800947335,-0.21381147512495,
-2.4363170142353));
#69920=CARTESIAN_POINT('Ctrl Pts',(-0.597626729206255,-0.568029385539622,
-2.42047490080706));
#69921=CARTESIAN_POINT('Ctrl Pts',(-0.253948036642577,-0.784426851263813,
-2.40463278737882));
#69922=CARTESIAN_POINT('Ctrl Pts',(0.151345833285741,-0.810499555240673,
-2.38879067395059));
#69923=CARTESIAN_POINT('Ctrl Pts',(0.519918803597792,-0.639921501407573,
-2.37294856052235));
#69924=CARTESIAN_POINT('Ctrl Pts',(0.762344355239403,-0.314079885272683,
-2.35710644709412));
#69925=CARTESIAN_POINT('Ctrl Pts',(0.819803000729591,0.0879666430702042,
-2.34126433366588));
#69926=CARTESIAN_POINT('Ctrl Pts',(0.678353602031553,0.468669906127011,
-2.32542222023765));
#69927=CARTESIAN_POINT('Ctrl Pts',(0.37231589598644,0.735660223128922,-2.30958010680941));
#69928=CARTESIAN_POINT('Ctrl Pts',(-0.0240564717090212,0.824157980284845,
-2.29373799338118));
#69929=CARTESIAN_POINT('Ctrl Pts',(-0.41459203991308,0.712691048589075,
-2.27789587995294));
#69930=CARTESIAN_POINT('Ctrl Pts',(-0.704535524748661,0.428304546631728,
-2.2620537665247));
#69931=CARTESIAN_POINT('Ctrl Pts',(-0.823538206532577,0.0399989084774863,
-2.24621165309647));
#69932=CARTESIAN_POINT('Ctrl Pts',(-0.74272657459735,-0.358011627863076,
-2.23036953966823));
#69933=CARTESIAN_POINT('Ctrl Pts',(-0.481707880491941,-0.669158133904268,
-2.21452742624));
#69934=CARTESIAN_POINT('Ctrl Pts',(-0.103812848664622,-0.81794742052923,
-2.19868531281176));
#69935=CARTESIAN_POINT('Ctrl Pts',(0.2992701986629,-0.768278880674557,-2.18284319938353));
#69936=CARTESIAN_POINT('Ctrl Pts',(0.629741594353524,-0.532203546248392,
-2.1670010859553));
#69937=CARTESIAN_POINT('Ctrl Pts',(0.80741936917992,-0.167000157399278,
-2.15115897252706));
#69938=CARTESIAN_POINT('Ctrl Pts',(0.789193728892756,0.238722325253902,
-2.13531685909882));
#69939=CARTESIAN_POINT('Ctrl Pts',(0.57948674374595,0.58652383082105,-2.11947474567059));
#69940=CARTESIAN_POINT('Ctrl Pts',(0.229179425679003,0.792017601536559,
-2.10363263224235));
#69941=CARTESIAN_POINT('Ctrl Pts',(-0.17673348457219,0.805344873783433,
-2.08779051881412));
#69942=CARTESIAN_POINT('Ctrl Pts',(-0.539765712845471,0.623272063817001,
-2.07194840538588));
#69943=CARTESIAN_POINT('Ctrl Pts',(-0.771835085205309,0.289975329199564,
-2.05610629195765));
#69944=CARTESIAN_POINT('Ctrl Pts',(-0.816634824375942,-0.113677851469657,
-2.04026417852941));
#69945=CARTESIAN_POINT('Ctrl Pts',(-0.663295211058166,-0.489749480127937,
-2.02442206510118));
#69946=CARTESIAN_POINT('Ctrl Pts',(-0.349020893874242,-0.746993645178798,
-2.00857995167294));
#69947=CARTESIAN_POINT('Ctrl Pts',(0.0499360401329562,-0.822995432669054,
-1.99273783824471));
#69948=CARTESIAN_POINT('Ctrl Pts',(0.43677703888679,-0.699314599160899,
-1.97689572481647));
#69949=CARTESIAN_POINT('Ctrl Pts',(0.717643228480402,-0.405959710949878,
-1.96105361138824));
#69950=CARTESIAN_POINT('Ctrl Pts',(0.824388304983522,-0.01410719336644,
-1.94521149796));
#69951=CARTESIAN_POINT('Ctrl Pts',(0.731112809166235,0.3811681395019,-1.92936938453177));
#69952=CARTESIAN_POINT('Ctrl Pts',(0.4604480883488,0.683960999059316,-1.91352727110353));
#69953=CARTESIAN_POINT('Ctrl Pts',(0.0780652735232223,0.820805033712652,
-1.8976851576753));
#69954=CARTESIAN_POINT('Ctrl Pts',(-0.32325844644872,0.758497901841424,
-1.88184304424706));
#69955=CARTESIAN_POINT('Ctrl Pts',(-0.646150268399774,0.512157125250817,
-1.86600093081883));
#69956=CARTESIAN_POINT('Ctrl Pts',(-0.812267248071997,0.141552138831698,
-1.85015881739059));
#69957=CARTESIAN_POINT('Ctrl Pts',(-0.781304576256766,-0.263397512172226,
-1.83431670396235));
#69958=CARTESIAN_POINT('Ctrl Pts',(-0.560774697392722,-0.604439268299457,
-1.81847459053412));
#69959=CARTESIAN_POINT('Ctrl Pts',(-0.204184572116599,-0.798826483541854,
-1.80263247710588));
#69960=CARTESIAN_POINT('Ctrl Pts',(0.201946667130782,-0.799395167569239,
-1.78679036367765));
#69961=CARTESIAN_POINT('Ctrl Pts',(0.55907977322475,-0.606007341101776,
-1.77094825024941));
#69962=CARTESIAN_POINT('Ctrl Pts',(0.780563870790618,-0.26558451369508,
-1.75510613682118));
#69963=CARTESIAN_POINT('Ctrl Pts',(0.812660477990166,0.139276838745992,
-1.73926402339294));
#69964=CARTESIAN_POINT('Ctrl Pts',(0.647582024690746,0.510345580558623,
-1.72342190996471));
#69965=CARTESIAN_POINT('Ctrl Pts',(0.325381343407219,0.757589645956699,
-1.70757979653647));
#69966=CARTESIAN_POINT('Ctrl Pts',(-0.07576631242369,0.821020435921054,
-1.69173768310823));
#69967=CARTESIAN_POINT('Ctrl Pts',(-0.458530857914507,0.685247796522155,
-1.67589556968));
#69968=CARTESIAN_POINT('Ctrl Pts',(-0.730042485245041,0.383214117740366,
-1.66005345625176));
#69969=CARTESIAN_POINT('Ctrl Pts',(-0.824424579278952,-0.0117984481609103,
-1.64421134282353));
#69970=CARTESIAN_POINT('Ctrl Pts',(-0.71877729979369,-0.403948367492151,
-1.6283692293953));
#69971=CARTESIAN_POINT('Ctrl Pts',(-0.438733748543603,-0.698088667854708,
-1.61252711596706));
#69972=CARTESIAN_POINT('Ctrl Pts',(-0.0522406334781668,-0.822852360093889,
-1.59668500253882));
#69973=CARTESIAN_POINT('Ctrl Pts',(0.346927578193464,-0.747968144901305,
-1.58084288911059));
#69974=CARTESIAN_POINT('Ctrl Pts',(0.661921072290253,-0.491605110181337,
-1.56500077568235));
#69975=CARTESIAN_POINT('Ctrl Pts',(0.816313268539809,-0.115964382049556,
-1.54915866225412));
#69976=CARTESIAN_POINT('Ctrl Pts',(0.772644131096213,0.28781267689395,-1.53331654882588));
#69977=CARTESIAN_POINT('Ctrl Pts',(0.541509062406833,0.621758012115288,
-1.51747443539765));
#69978=CARTESIAN_POINT('Ctrl Pts',(0.178988150511605,0.80484677565032,-1.50163232196941));
#69979=CARTESIAN_POINT('Ctrl Pts',(-0.226960490874059,0.792656310061612,
-1.48579020854118));
#69980=CARTESIAN_POINT('Ctrl Pts',(-0.577841918175875,0.588144376745292,
-1.46994809511294));
#69981=CARTESIAN_POINT('Ctrl Pts',(-0.788522095065032,0.240931517017877,
-1.45410598168471));
#69982=CARTESIAN_POINT('Ctrl Pts',(-0.807883884989266,-0.164738333950945,
-1.43826386825647));
#69983=CARTESIAN_POINT('Ctrl Pts',(-0.631229554758549,-0.530437875247995,
-1.42242175482823));
#69984=CARTESIAN_POINT('Ctrl Pts',(-0.301420581206097,-0.767437765244623,
-1.4065796414));
#69985=CARTESIAN_POINT('Ctrl Pts',(0.101521789311754,-0.818234939728941,
-1.39073752797176));
#69986=CARTESIAN_POINT('Ctrl Pts',(0.479832021942188,-0.670504527216002,
-1.37489541454353));
#69987=CARTESIAN_POINT('Ctrl Pts',(0.741721054676472,-0.360090221122297,
-1.35905330111529));
#69988=CARTESIAN_POINT('Ctrl Pts',(0.823646993609409,0.0376924424316771,
-1.34321118768706));
#69989=CARTESIAN_POINT('Ctrl Pts',(0.705732223915323,0.426329823523777,
-1.32736907425882));
#69990=CARTESIAN_POINT('Ctrl Pts',(0.416586297157071,0.711527193661101,
-1.31152696083059));
#69991=CARTESIAN_POINT('Ctrl Pts',(0.0263644222388554,0.824087378582086,
-1.29568484740235));
#69992=CARTESIAN_POINT('Ctrl Pts',(-0.370254228074203,0.736700004677249,
-1.27984273397412));
#69993=CARTESIAN_POINT('Ctrl Pts',(-0.677038437316519,0.470567789690592,
-1.26400062054588));
#69994=CARTESIAN_POINT('Ctrl Pts',(-0.819553436410745,0.090262146914535,
-1.24815850711765));
#69995=CARTESIAN_POINT('Ctrl Pts',(-0.763220942876712,-0.311943717123242,
-1.23231639368941));
#69996=CARTESIAN_POINT('Ctrl Pts',(-0.521708857543189,-0.63846296545631,
-1.21647428026118));
#69997=CARTESIAN_POINT('Ctrl Pts',(-0.153615034405297,-0.810072534717071,
-1.20063216683294));
#69998=CARTESIAN_POINT('Ctrl Pts',(0.251750262518701,-0.785134953762758,
-1.18479005340471));
#69999=CARTESIAN_POINT('Ctrl Pts',(0.596033625981975,-0.569700804806402,
-1.16894793997647));
#70000=CARTESIAN_POINT('Ctrl Pts',(0.79570190178519,-0.216040676248052,
-1.15310582654824));
#70001=CARTESIAN_POINT('Ctrl Pts',(0.802309760756444,0.190037201866422,
-1.13726371312));
#70002=CARTESIAN_POINT('Ctrl Pts',(0.614253944182277,0.550006529374697,
-1.12142159969176));
#70003=CARTESIAN_POINT('Ctrl Pts',(0.277162260987144,0.776528281122316,
-1.10557948626353));
#70004=CARTESIAN_POINT('Ctrl Pts',(-0.127177045364621,0.814641693894075,
-1.08973737283529));
#70005=CARTESIAN_POINT('Ctrl Pts',(-0.500659502770236,0.655099345583663,
-1.07389525940706));
#70006=CARTESIAN_POINT('Ctrl Pts',(-0.752667407860654,0.336610848670395,
-1.05805314597882));
#70007=CARTESIAN_POINT('Ctrl Pts',(-0.822056315596167,-0.0635492272709786,
-1.04221103255059));
#70008=CARTESIAN_POINT('Ctrl Pts',(-0.691990459440485,-0.448290412948603,
-1.02636891912235));
#70009=CARTESIAN_POINT('Ctrl Pts',(-0.394027597831391,-0.724263310161095,
-1.01052680569412));
#70010=CARTESIAN_POINT('Ctrl Pts',(-0.000462184425002042,-0.824508869984938,
-0.994684692265883));
#70011=CARTESIAN_POINT('Ctrl Pts',(0.393215368361151,-0.724704604913538,
-0.978842578837647));
#70012=CARTESIAN_POINT('Ctrl Pts',(0.691487439835499,-0.449065931515664,
-0.963000465409414));
#70013=CARTESIAN_POINT('Ctrl Pts',(0.821984553038164,-0.0644708062996728,
-0.947158351981175));
#70014=CARTESIAN_POINT('Ctrl Pts',(0.753044314032747,0.335766811047835,
-0.931316238552943));
#70015=CARTESIAN_POINT('Ctrl Pts',(0.50139362927632,0.654537637435314,-0.915474125124704));
#70016=CARTESIAN_POINT('Ctrl Pts',(0.128090271769204,0.814498601948693,
-0.899632011696473));
#70017=CARTESIAN_POINT('Ctrl Pts',(-0.276291509962364,0.776838523646324,
-0.883789898268234));
#70018=CARTESIAN_POINT('Ctrl Pts',(-0.613636938053462,0.550694832511305,
-0.867947784840001));
#70019=CARTESIAN_POINT('Ctrl Pts',(-0.802096203150231,0.190936563261905,
-0.852105671411765));
#70020=CARTESIAN_POINT('Ctrl Pts',(-0.795943607986144,-0.21514846781765,
-0.83626355798353));
#70021=CARTESIAN_POINT('Ctrl Pts',(-0.59667195103801,-0.569032225047738,
-0.820421444555294));
#70022=CARTESIAN_POINT('Ctrl Pts',(-0.252630330211578,-0.784852219564593,
-0.804579331127059));
#70023=CARTESIAN_POINT('Ctrl Pts',(0.152706754086307,-0.810244245616536,
-0.788737217698825));
#70024=CARTESIAN_POINT('Ctrl Pts',(0.520992739812211,-0.639047459396599,
-0.772895104270588));
#70025=CARTESIAN_POINT('Ctrl Pts',(0.762870738716788,-0.312799178879975,
-0.757052990842355));
#70026=CARTESIAN_POINT('Ctrl Pts',(0.819654115533445,0.0893432772365556,
-0.741210877414117));
#70027=CARTESIAN_POINT('Ctrl Pts',(0.677565572039378,0.469808456591869,
-0.725368763985883));
#70028=CARTESIAN_POINT('Ctrl Pts',(0.371079920186729,0.736284444445551,
-0.709526650557647));
#70029=CARTESIAN_POINT('Ctrl Pts',(-0.0254405096505967,0.824116418212256,
-0.693684537129412));
#70030=CARTESIAN_POINT('Ctrl Pts',(-0.415788332150249,0.711993787294522,
-0.677842423701178));
#70031=CARTESIAN_POINT('Ctrl Pts',(-0.70525381600185,0.427120761978518,
-0.662000310272941));
#70032=CARTESIAN_POINT('Ctrl Pts',(-0.823604218459063,0.0386158210416587,
-0.646158196844706));
#70033=CARTESIAN_POINT('Ctrl Pts',(-0.742124290784431,-0.359258440855583,
-0.630316083416471));
#70034=CARTESIAN_POINT('Ctrl Pts',(-0.480583432504365,-0.669966159369718,
-0.614473969988236));
#70035=CARTESIAN_POINT('Ctrl Pts',(-0.102439060278077,-0.818120607995927,
-0.598631856560001));
#70036=CARTESIAN_POINT('Ctrl Pts',(0.30056000644216,-0.767775209827565,
-0.582789743131765));
#70037=CARTESIAN_POINT('Ctrl Pts',(0.630634476656484,-0.53114522227968,
-0.566947629703531));
#70038=CARTESIAN_POINT('Ctrl Pts',(0.807698686798682,-0.165643960475012,
-0.551105516275293));
#70039=CARTESIAN_POINT('Ctrl Pts',(0.788791711252022,0.240047342327775,
-0.53526340284706));
#70040=CARTESIAN_POINT('Ctrl Pts',(0.578500932013622,0.587496180376762,
-0.519421289418824));
#70041=CARTESIAN_POINT('Ctrl Pts',(0.227849006445562,0.792401363300445,
-0.503579175990589));
#70042=CARTESIAN_POINT('Ctrl Pts',(-0.178085712920448,0.805046935993242,
-0.487737062562353));
#70043=CARTESIAN_POINT('Ctrl Pts',(-0.540811660389811,0.62236471484382,
-0.471894949134118));
#70044=CARTESIAN_POINT('Ctrl Pts',(-0.772320974669179,0.28867871828499,
-0.456052835705883));
#70045=CARTESIAN_POINT('Ctrl Pts',(-0.816442764829873,-0.115049128816222,
-0.440210722277647));
#70046=CARTESIAN_POINT('Ctrl Pts',(-0.662471801767662,-0.490862712155255,
-0.424368608849413));
#70047=CARTESIAN_POINT('Ctrl Pts',(-0.347765917804802,-0.747578729422039,
-0.408526495421177));
#70048=CARTESIAN_POINT('Ctrl Pts',(0.0513180891615079,-0.822910410693275,
-0.392684381992942));
#70049=CARTESIAN_POINT('Ctrl Pts',(0.437950835863752,-0.698580099741808,
-0.376842268564706));
#70050=CARTESIAN_POINT('Ctrl Pts',(0.71832397560555,-0.40475394505682,-0.361000155136471));
#70051=CARTESIAN_POINT('Ctrl Pts',(0.824410834241176,-0.0127227147567732,
-0.345158041708236));
#70052=CARTESIAN_POINT('Ctrl Pts',(0.730471652282162,0.38239541585384,-0.32931592828));
#70053=CARTESIAN_POINT('Ctrl Pts',(0.459298812591734,0.684733300637323,
-0.313473814851765));
#70054=CARTESIAN_POINT('Ctrl Pts',(0.0766867188231743,0.820934976893245,
-0.29763170142353));
#70055=CARTESIAN_POINT('Ctrl Pts',(-0.324531787362575,0.757953960211733,
-0.281789587995295));
#70056=CARTESIAN_POINT('Ctrl Pts',(-0.647009475978688,0.511071271763133,
-0.265947474567059));
#70057=CARTESIAN_POINT('Ctrl Pts',(-0.812503794740706,0.140187839202379,
-0.250105361138824));
#70058=CARTESIAN_POINT('Ctrl Pts',(-0.780861184376679,-0.264709251133773,
-0.234263247710588));
#70059=CARTESIAN_POINT('Ctrl Pts',(-0.559758720137868,-0.605380157133335,
-0.218421134282353));
#70060=CARTESIAN_POINT('Ctrl Pts',(-0.202842959779694,-0.799168281276578,
-0.202579020854118));
#70061=CARTESIAN_POINT('Ctrl Pts',(0.203289273038814,-0.799054853830805,
-0.186736907425883));
#70062=CARTESIAN_POINT('Ctrl Pts',(0.560095904927298,-0.605067663119104,
-0.170894793997648));
#70063=CARTESIAN_POINT('Ctrl Pts',(0.781010346026423,-0.264273116881618,
-0.155052680569412));
#70064=CARTESIAN_POINT('Ctrl Pts',(0.812422373100201,0.140641088911458,
-0.139210567141177));
#70065=CARTESIAN_POINT('Ctrl Pts',(0.646730057822694,0.51143301626051,-0.123368453712942));
#70066=CARTESIAN_POINT('Ctrl Pts',(0.32409678542623,0.758133800545566,-0.107526340284707));
#70067=CARTESIAN_POINT('Ctrl Pts',(-0.0771214967823103,0.820894379703354,
-0.0916842268564712));
#70068=CARTESIAN_POINT('Ctrl Pts',(-0.459730603216706,0.684472654204421,
-0.0758421134282357));
#70069=CARTESIAN_POINT('Ctrl Pts',(-0.640274482293033,0.4828170276367,-0.0652807044760789));
#70070=CARTESIAN_POINT('Ctrl Pts',(-0.701077753000059,0.366509473613423,
-0.0600000000000005));
#70071=CARTESIAN_POINT('Ctrl Pts',(0.437168237015825,-0.613060138694066,
-2.9529325805302));
#70072=CARTESIAN_POINT('Ctrl Pts',(0.538873825155734,-0.540534704637147,
-2.94765187605412));
#70073=CARTESIAN_POINT('Ctrl Pts',(0.705393947234175,-0.343965226545598,
-2.93709046710196));
#70074=CARTESIAN_POINT('Ctrl Pts',(0.784003077920512,0.0345814394106197,
-2.92124835367372));
#70075=CARTESIAN_POINT('Ctrl Pts',(0.672394775942478,0.404639543367737,
-2.90540624024549));
#70076=CARTESIAN_POINT('Ctrl Pts',(0.397642184080878,0.676568411154076,
-2.88956412681725));
#70077=CARTESIAN_POINT('Ctrl Pts',(0.02641088878806,0.784317782616846,-2.87372201338902));
#70078=CARTESIAN_POINT('Ctrl Pts',(-0.351228885865366,0.701781236716768,
-2.85787989996078));
#70079=CARTESIAN_POINT('Ctrl Pts',(-0.643650102008308,0.448965850545129,
-2.84203778653255));
#70080=CARTESIAN_POINT('Ctrl Pts',(-0.779903200303776,0.0872215090938687,
-2.82619567310431));
#70081=CARTESIAN_POINT('Ctrl Pts',(-0.726929049354935,-0.295686944193908,
-2.81035355967608));
#70082=CARTESIAN_POINT('Ctrl Pts',(-0.497580804097368,-0.606852313043473,
-2.79451144624784));
#70083=CARTESIAN_POINT('Ctrl Pts',(-0.147504973602872,-0.770778091433911,
-2.77866933281961));
#70084=CARTESIAN_POINT('Ctrl Pts',(0.238359844765566,-0.747690477369339,
-2.76282721939137));
#70085=CARTESIAN_POINT('Ctrl Pts',(0.566391638179665,-0.543191524409974,
-2.74698510596314));
#70086=CARTESIAN_POINT('Ctrl Pts',(0.757000350081665,-0.20689845778034,
-2.7311429925349));
#70087=CARTESIAN_POINT('Ctrl Pts',(0.763938767856739,0.179594161720182,
-2.71530087910667));
#70088=CARTESIAN_POINT('Ctrl Pts',(0.585523428114815,0.522512030400192,
-2.69945876567843));
#70089=CARTESIAN_POINT('Ctrl Pts',(0.265043080562979,0.738653280743715,
-2.6836166522502));
#70090=CARTESIAN_POINT('Ctrl Pts',(-0.119744424734367,0.775575772232499,
-2.66777453882196));
#70091=CARTESIAN_POINT('Ctrl Pts',(-0.475478450890907,0.624321029163851,
-2.65193242539373));
#70092=CARTESIAN_POINT('Ctrl Pts',(-0.715847580104881,0.321587852936783,
-2.63609031196549));
#70093=CARTESIAN_POINT('Ctrl Pts',(-0.782531272716308,-0.059171887253674,
-2.62024819853726));
#70094=CARTESIAN_POINT('Ctrl Pts',(-0.659350126059844,-0.425574806886333,
-2.60440608510902));
#70095=CARTESIAN_POINT('Ctrl Pts',(-0.376191467858767,-0.688720904683293,
-2.58856397168079));
#70096=CARTESIAN_POINT('Ctrl Pts',(-0.00175782158908592,-0.784763286008587,
-2.57272185825255));
#70097=CARTESIAN_POINT('Ctrl Pts',(0.373102323308885,-0.690399276769274,
-2.55687974482431));
#70098=CARTESIAN_POINT('Ctrl Pts',(0.657436996421685,-0.428524329239833,
-2.54103763139608));
#70099=CARTESIAN_POINT('Ctrl Pts',(0.782258338870179,-0.0626769198712575,
-2.52519551796784));
#70100=CARTESIAN_POINT('Ctrl Pts',(0.717281063728533,0.318377732627569,
-2.50935340453961));
#70101=CARTESIAN_POINT('Ctrl Pts',(0.47827054719541,0.622184690185607,-2.49351129111137));
#70102=CARTESIAN_POINT('Ctrl Pts',(0.123217689940382,0.775031551552749,
-2.47766917768314));
#70103=CARTESIAN_POINT('Ctrl Pts',(-0.261731361514479,0.739833224055233,
-2.4618270642549));
#70104=CARTESIAN_POINT('Ctrl Pts',(-0.58317677468645,0.525129845355069,
-2.44598495082667));
#70105=CARTESIAN_POINT('Ctrl Pts',(-0.763126546142486,0.183014697740164,
-2.43014283739843));
#70106=CARTESIAN_POINT('Ctrl Pts',(-0.757919629191393,-0.203505136796763,
-2.41430072397019));
#70107=CARTESIAN_POINT('Ctrl Pts',(-0.568819373279402,-0.540648708126009,
-2.39845861054196));
#70108=CARTESIAN_POINT('Ctrl Pts',(-0.241706998681967,-0.746615183213176,
-2.38261649711372));
#70109=CARTESIAN_POINT('Ctrl Pts',(0.144050521556132,-0.771431106616591,
-2.36677438368549));
#70110=CARTESIAN_POINT('Ctrl Pts',(0.494857196918661,-0.609075413782312,
-2.35093227025725));
#70111=CARTESIAN_POINT('Ctrl Pts',(0.725597128070741,-0.298940316370648,
-2.33509015682902));
#70112=CARTESIAN_POINT('Ctrl Pts',(0.780286098827823,0.083726393642309,
-2.31924804340078));
#70113=CARTESIAN_POINT('Ctrl Pts',(0.645654974773131,0.446078646167914,
-2.30340592997255));
#70114=CARTESIAN_POINT('Ctrl Pts',(0.354369181074354,0.700199249157682,
-2.28756381654431));
#70115=CARTESIAN_POINT('Ctrl Pts',(-0.0228968794267542,0.784431155633691,
-2.27172170311608));
#70116=CARTESIAN_POINT('Ctrl Pts',(-0.394607491239903,0.678337255997074,
-2.25587958968784));
#70117=CARTESIAN_POINT('Ctrl Pts',(-0.670574852254142,0.407659015036618,
-2.24003747625961));
#70118=CARTESIAN_POINT('Ctrl Pts',(-0.783841256788622,0.0380708441241249,
-2.22419536283137));
#70119=CARTESIAN_POINT('Ctrl Pts',(-0.706924981821915,-0.340754420503058,
-2.20835324940314));
#70120=CARTESIAN_POINT('Ctrl Pts',(-0.458488152042827,-0.636902755098958,
-2.1925111359749));
#70121=CARTESIAN_POINT('Ctrl Pts',(-0.0988087657896205,-0.778519963019204,
-2.17666902254667));
#70122=CARTESIAN_POINT('Ctrl Pts',(0.284844499961923,-0.73124559202619,
-2.16082690911843));
#70123=CARTESIAN_POINT('Ctrl Pts',(0.599386208016341,-0.506549779050472,
-2.1449847956902));
#70124=CARTESIAN_POINT('Ctrl Pts',(0.768499394531042,-0.158950261471042,
-2.12914268226196));
#70125=CARTESIAN_POINT('Ctrl Pts',(0.751152283401107,0.227215211105232,
-2.11330056883372));
#70126=CARTESIAN_POINT('Ctrl Pts',(0.551553788163199,0.558251667063445,
-2.09745845540549));
#70127=CARTESIAN_POINT('Ctrl Pts',(0.218132307195168,0.753840037125916,
-2.08161634197725));
#70128=CARTESIAN_POINT('Ctrl Pts',(-0.168214413812045,0.7665248958789,-2.06577422854902));
#70129=CARTESIAN_POINT('Ctrl Pts',(-0.513747427104302,0.593228527769866,
-2.04993211512079));
#70130=CARTESIAN_POINT('Ctrl Pts',(-0.734630377099514,0.275997670386755,
-2.03409000169254));
#70131=CARTESIAN_POINT('Ctrl Pts',(-0.777270637838795,-0.108198246612234,
-2.01824788826432));
#70132=CARTESIAN_POINT('Ctrl Pts',(-0.631322442278385,-0.46614212306114,
-2.00240577483608));
#70133=CARTESIAN_POINT('Ctrl Pts',(-0.33219706618317,-0.710986367123579,
-1.98656366140784));
#70134=CARTESIAN_POINT('Ctrl Pts',(0.0475289769756635,-0.7833246462125,
-1.97072154797961));
#70135=CARTESIAN_POINT('Ctrl Pts',(0.415723108389742,-0.665605590546729,
-1.95487943455137));
#70136=CARTESIAN_POINT('Ctrl Pts',(0.683050726336488,-0.386391265775365,
-1.93903732112314));
#70137=CARTESIAN_POINT('Ctrl Pts',(0.784650378008375,-0.0134271853939425,
-1.9231952076949));
#70138=CARTESIAN_POINT('Ctrl Pts',(0.695871033845534,0.362794720566657,
-1.90735309426667));
#70139=CARTESIAN_POINT('Ctrl Pts',(0.438253144048835,0.650992078867018,
-1.89151098083843));
#70140=CARTESIAN_POINT('Ctrl Pts',(0.0743022990610538,0.781239830890958,
-1.8756688674102));
#70141=CARTESIAN_POINT('Ctrl Pts',(-0.30767644405807,0.721936084974336,
-1.85982675398196));
#70142=CARTESIAN_POINT('Ctrl Pts',(-0.615003935991344,0.487469654164693,
-1.84398464055373));
#70143=CARTESIAN_POINT('Ctrl Pts',(-0.773113591484361,0.134728911813473,
-1.82814252712549));
#70144=CARTESIAN_POINT('Ctrl Pts',(-0.743643410991619,-0.250700981858951,
-1.81230041369726));
#70145=CARTESIAN_POINT('Ctrl Pts',(-0.533743717161932,-0.5753035280671,
-1.79645830026902));
#70146=CARTESIAN_POINT('Ctrl Pts',(-0.194342278664382,-0.760320711108034,
-1.78061618684078));
#70147=CARTESIAN_POINT('Ctrl Pts',(0.192212247242966,-0.760861982902353,
-1.76477407341255));
#70148=CARTESIAN_POINT('Ctrl Pts',(0.532130493295156,-0.576796015174987,
-1.74893195998431));
#70149=CARTESIAN_POINT('Ctrl Pts',(0.742938409694909,-0.252782563513171,
-1.73308984655608));
#70150=CARTESIAN_POINT('Ctrl Pts',(0.773487866570592,0.132563287845333,
-1.71724773312784));
#70151=CARTESIAN_POINT('Ctrl Pts',(0.616366677442347,0.485745431223982,
-1.70140561969961));
#70152=CARTESIAN_POINT('Ctrl Pts',(0.309697011175393,0.721071609679177,
-1.68556350627137));
#70153=CARTESIAN_POINT('Ctrl Pts',(-0.0721141546091439,0.781444850083036,
-1.66972139284314));
#70154=CARTESIAN_POINT('Ctrl Pts',(-0.436428329727842,0.652216848929293,
-1.6538792794149));
#70155=CARTESIAN_POINT('Ctrl Pts',(-0.694852302667184,0.364742076671178,
-1.63803716598667));
#70156=CARTESIAN_POINT('Ctrl Pts',(-0.784684903776692,-0.0112297284585551,
-1.62219505255843));
#70157=CARTESIAN_POINT('Ctrl Pts',(-0.684130132096222,-0.384476874953873,
-1.6063529391302));
#70158=CARTESIAN_POINT('Ctrl Pts',(-0.417585498919284,-0.664438752714366,
-1.59051082570196));
#70159=CARTESIAN_POINT('Ctrl Pts',(-0.0497224821825411,-0.783188470153831,
-1.57466871227372));
#70160=CARTESIAN_POINT('Ctrl Pts',(0.330204654439483,-0.711913893109829,
-1.55882659884549));
#70161=CARTESIAN_POINT('Ctrl Pts',(0.630014541017341,-0.46790830631973,
-1.54298448541725));
#70162=CARTESIAN_POINT('Ctrl Pts',(0.776964581934259,-0.110374559731907,
-1.52714237198902));
#70163=CARTESIAN_POINT('Ctrl Pts',(0.735400424612663,0.273939264246303,
-1.51130025856078));
#70164=CARTESIAN_POINT('Ctrl Pts',(0.515406742118902,0.591787457787566,
-1.49545814513255));
#70165=CARTESIAN_POINT('Ctrl Pts',(0.170360398260084,0.766050807532343,
-1.47961603170431));
#70166=CARTESIAN_POINT('Ctrl Pts',(-0.216020331536435,0.754447958032348,
-1.46377391827608));
#70167=CARTESIAN_POINT('Ctrl Pts',(-0.549988247995402,0.559794097935337,
-1.44793180484784));
#70168=CARTESIAN_POINT('Ctrl Pts',(-0.750513024287871,0.229317913366062,
-1.43208969141961));
#70169=CARTESIAN_POINT('Ctrl Pts',(-0.76894151932004,-0.156797464526944,
-1.41624757799137));
#70170=CARTESIAN_POINT('Ctrl Pts',(-0.600802444378748,-0.504869218555471,
-1.40040546456314));
#70171=CARTESIAN_POINT('Ctrl Pts',(-0.286891227778387,-0.730445020819569,
-1.3845633511349));
#70172=CARTESIAN_POINT('Ctrl Pts',(0.0966281421970794,-0.778793622952724,
-1.36872123770667));
#70173=CARTESIAN_POINT('Ctrl Pts',(0.456702715360558,-0.638184248315942,
-1.35287912427843));
#70174=CARTESIAN_POINT('Ctrl Pts',(0.705967930901566,-0.34273281948896,
-1.3370370108502));
#70175=CARTESIAN_POINT('Ctrl Pts',(0.783944800010236,0.0358755564862942,
-1.32119489742196));
#70176=CARTESIAN_POINT('Ctrl Pts',(0.671713867021582,0.405779479356957,
-1.30535278399373));
#70177=CARTESIAN_POINT('Ctrl Pts',(0.396505619453125,0.677229502279976,
-1.28951067056549));
#70178=CARTESIAN_POINT('Ctrl Pts',(0.0250935799921388,0.784363957139456,
-1.27366855713726));
#70179=CARTESIAN_POINT('Ctrl Pts',(-0.352406891584218,0.70118891019485,
-1.25782644370902));
#70180=CARTESIAN_POINT('Ctrl Pts',(-0.644403204843168,0.447885046193937,
-1.24198433028078));
#70181=CARTESIAN_POINT('Ctrl Pts',(-0.780048564238921,0.0859112474888284,
-1.22614221685255));
#70182=CARTESIAN_POINT('Ctrl Pts',(-0.726431461620614,-0.296907117772595,
-1.21030010342431));
#70183=CARTESIAN_POINT('Ctrl Pts',(-0.496560965029412,-0.607687183528952,
-1.19445798999608));
#70184=CARTESIAN_POINT('Ctrl Pts',(-0.146210340546125,-0.77102466973092,
-1.17861587656784));
#70185=CARTESIAN_POINT('Ctrl Pts',(0.239615163697594,-0.747289153101038,
-1.16277376313961));
#70186=CARTESIAN_POINT('Ctrl Pts',(0.567303062289086,-0.542239560096563,
-1.14693164971137));
#70187=CARTESIAN_POINT('Ctrl Pts',(0.757346743328938,-0.205626883907099,
-1.13108953628314));
#70188=CARTESIAN_POINT('Ctrl Pts',(0.763636084175085,0.180876853029987,
-1.1152474228549));
#70189=CARTESIAN_POINT('Ctrl Pts',(0.584645107872305,0.52349460633064,-1.09940530942667));
#70190=CARTESIAN_POINT('Ctrl Pts',(0.263802229530127,0.739097347249484,
-1.08356319599843));
#70191=CARTESIAN_POINT('Ctrl Pts',(-0.12104673988714,0.775373582074464,
-1.0677210825702));
#70192=CARTESIAN_POINT('Ctrl Pts',(-0.47652625070901,0.623521641486088,
-1.05187896914196));
#70193=CARTESIAN_POINT('Ctrl Pts',(-0.716386637852962,0.320385221447583,
-1.03603685571372));
#70194=CARTESIAN_POINT('Ctrl Pts',(-0.78243079732869,-0.0604859686859734,
-1.02019474228549));
#70195=CARTESIAN_POINT('Ctrl Pts',(-0.658634495778076,-0.426681504154387,
-1.00435262885725));
#70196=CARTESIAN_POINT('Ctrl Pts',(-0.375034315401055,-0.689351700721738,
-0.988510515429021));
#70197=CARTESIAN_POINT('Ctrl Pts',(-0.000439905784195014,-0.784765131424169,
-0.972668402000785));
#70198=CARTESIAN_POINT('Ctrl Pts',(0.374261237766406,-0.689771723776676,
-0.956826288572549));
#70199=CARTESIAN_POINT('Ctrl Pts',(0.658155723188982,-0.42741964045874,
-0.940984175144316));
#70200=CARTESIAN_POINT('Ctrl Pts',(0.782362493935833,-0.0613631249105981,
-0.925142061716077));
#70201=CARTESIAN_POINT('Ctrl Pts',(0.716745376045408,0.31958186890657,-0.909299948287845));
#70202=CARTESIAN_POINT('Ctrl Pts',(0.477224990170764,0.622987009313038,
-0.893457834859608));
#70203=CARTESIAN_POINT('Ctrl Pts',(0.12191594610856,0.77523738757928,-0.877615721431374));
#70204=CARTESIAN_POINT('Ctrl Pts',(-0.262973451250997,0.739392635176622,
-0.861773608003137));
#70205=CARTESIAN_POINT('Ctrl Pts',(-0.584057843243151,0.524149731243324,
-0.845931494574904));
#70206=CARTESIAN_POINT('Ctrl Pts',(-0.763432820669978,0.181732862576291,
-0.830089381146666));
#70207=CARTESIAN_POINT('Ctrl Pts',(-0.757576798584207,-0.204777682532043,
-0.814247267718432));
#70208=CARTESIAN_POINT('Ctrl Pts',(-0.567910618210827,-0.541603207837332,
-0.798405154290196));
#70209=CARTESIAN_POINT('Ctrl Pts',(-0.240452809554177,-0.747020047517997,
-0.782563040861961));
#70210=CARTESIAN_POINT('Ctrl Pts',(0.145345841994508,-0.771188103662912,
-0.766720927433726));
#70211=CARTESIAN_POINT('Ctrl Pts',(0.495879366267142,-0.60824350315214,
-0.750878814005491));
#70212=CARTESIAN_POINT('Ctrl Pts',(0.726098138325266,-0.297721343771107,
-0.735036700577256));
#70213=CARTESIAN_POINT('Ctrl Pts',(0.780144390333501,0.0850366700162907,
-0.71919458714902));
#70214=CARTESIAN_POINT('Ctrl Pts',(0.644904930130934,0.447162315171019,
-0.703352473720785));
#70215=CARTESIAN_POINT('Ctrl Pts',(0.353192782922427,0.700793381181502,
-0.68751036029255));
#70216=CARTESIAN_POINT('Ctrl Pts',(-0.0242142026923446,0.784391596974536,
-0.671668246864314));
#70217=CARTESIAN_POINT('Ctrl Pts',(-0.395746118693045,0.67767360473585,
-0.655826133436079));
#70218=CARTESIAN_POINT('Ctrl Pts',(-0.671258519768501,0.406532292265314,
-0.639984020007844));
#70219=CARTESIAN_POINT('Ctrl Pts',(-0.78390408674722,0.0367544255471266,
-0.624141906579608));
#70220=CARTESIAN_POINT('Ctrl Pts',(-0.706351729849976,-0.341941133463399,
-0.608299793151373));
#70221=CARTESIAN_POINT('Ctrl Pts',(-0.457417905736359,-0.637671831374146,
-0.592457679723138));
#70222=CARTESIAN_POINT('Ctrl Pts',(-0.0975011980205375,-0.778684802343572,
-0.576615566294902));
#70223=CARTESIAN_POINT('Ctrl Pts',(0.28607213523457,-0.730766199586856,
-0.560773452866667));
#70224=CARTESIAN_POINT('Ctrl Pts',(0.600236050781331,-0.505542469391802,
-0.544931339438432));
#70225=CARTESIAN_POINT('Ctrl Pts',(0.7687652482238,-0.157659437204313,-0.529089226010197));
#70226=CARTESIAN_POINT('Ctrl Pts',(0.750769644186234,0.228476358481531,
-0.513247112581962));
#70227=CARTESIAN_POINT('Ctrl Pts',(0.550615495439079,0.55917714652723,-0.497404999153727));
#70228=CARTESIAN_POINT('Ctrl Pts',(0.216866018059188,0.754205300450586,
-0.481562885725491));
#70229=CARTESIAN_POINT('Ctrl Pts',(-0.169501460799733,0.766241319561427,
-0.465720772297256));
#70230=CARTESIAN_POINT('Ctrl Pts',(-0.514742956918447,0.592364915670458,
-0.44987865886902));
#70231=CARTESIAN_POINT('Ctrl Pts',(-0.735092845270387,0.274763559909812,
-0.434036545440785));
#70232=CARTESIAN_POINT('Ctrl Pts',(-0.777087836124468,-0.109503424380808,
-0.418194432012549));
#70233=CARTESIAN_POINT('Ctrl Pts',(-0.630538723723493,-0.467201694049429,
-0.402352318584315));
#70234=CARTESIAN_POINT('Ctrl Pts',(-0.331002583630077,-0.711543248595394,
-0.386510205156079));
#70235=CARTESIAN_POINT('Ctrl Pts',(0.0488444071996538,-0.783243722544574,
-0.370668091727844));
#70236=CARTESIAN_POINT('Ctrl Pts',(0.41684032492,-0.66490649614746,-0.354825978299608));
#70237=CARTESIAN_POINT('Ctrl Pts',(0.683698659459563,-0.385243621324251,
-0.338983864871373));
#70238=CARTESIAN_POINT('Ctrl Pts',(0.784671821289931,-0.0121094427017519,
-0.323141751443138));
#70239=CARTESIAN_POINT('Ctrl Pts',(0.695260782598142,0.363962838609635,
-0.307299638014903));
#70240=CARTESIAN_POINT('Ctrl Pts',(0.43715926674397,0.651727153250601,-0.291457524586667));
#70241=CARTESIAN_POINT('Ctrl Pts',(0.0729901947287151,0.781363510430267,
-0.275615411158432));
#70242=CARTESIAN_POINT('Ctrl Pts',(-0.308888406216377,0.721418362921788,
-0.259773297730197));
#70243=CARTESIAN_POINT('Ctrl Pts',(-0.61582172725246,0.486436141990367,
-0.243931184301961));
#70244=CARTESIAN_POINT('Ctrl Pts',(-0.77333873591193,0.133430375415769,
-0.228089070873726));
#70245=CARTESIAN_POINT('Ctrl Pts',(-0.743221391896717,-0.251949491166766,
-0.212246957445491));
#70246=CARTESIAN_POINT('Ctrl Pts',(-0.532776712981681,-0.57619906330784,
-0.196404844017256));
#70247=CARTESIAN_POINT('Ctrl Pts',(-0.193065335965257,-0.760646033192459,
-0.18056273058902));
#70248=CARTESIAN_POINT('Ctrl Pts',(0.193490135620185,-0.760538073281255,
-0.164720617160785));
#70249=CARTESIAN_POINT('Ctrl Pts',(0.53309764447827,-0.575901632418885,
-0.14887850373255));
#70250=CARTESIAN_POINT('Ctrl Pts',(0.743363363518767,-0.251534379860902,
-0.133036390304315));
#70251=CARTESIAN_POINT('Ctrl Pts',(0.773261239032588,0.133861777163485,
-0.117194276876079));
#70252=CARTESIAN_POINT('Ctrl Pts',(0.615555777868655,0.486780449345162,
-0.101352163447844));
#70253=CARTESIAN_POINT('Ctrl Pts',(0.308474372645389,0.721589534425644,
-0.0855100500196088));
#70254=CARTESIAN_POINT('Ctrl Pts',(-0.0734040151188502,0.781324870143642,
-0.0696679365913733));
#70255=CARTESIAN_POINT('Ctrl Pts',(-0.437570243798181,0.651479070737944,
-0.0538258231631379));
#70256=CARTESIAN_POINT('Ctrl Pts',(-0.609411379956911,0.459543835051841,
-0.0432644142109811));
#70257=CARTESIAN_POINT('Ctrl Pts',(-0.667283755215033,0.348842645238846,
-0.0379837097349027));
#70258=CARTESIAN_POINT('Ctrl Pts',(0.415028236876551,-0.582012248186914,
-2.9309162902651));
#70259=CARTESIAN_POINT('Ctrl Pts',(0.511583035126158,-0.513159800829765,
-2.92563558578902));
#70260=CARTESIAN_POINT('Ctrl Pts',(0.669669892356321,-0.326545410742852,
-2.91507417683687));
#70261=CARTESIAN_POINT('Ctrl Pts',(0.744297932887927,0.0328300928841836,
-2.89923206340863));
#70262=CARTESIAN_POINT('Ctrl Pts',(0.638341935016441,0.3841469302546,-2.88338994998039));
#70263=CARTESIAN_POINT('Ctrl Pts',(0.377503946062879,0.642304200150481,
-2.86754783655216));
#70264=CARTESIAN_POINT('Ctrl Pts',(0.0250733325981615,0.744596699642227,
-2.85170572312392));
#70265=CARTESIAN_POINT('Ctrl Pts',(-0.333441208436975,0.666240144379612,
-2.83586360969569));
#70266=CARTESIAN_POINT('Ctrl Pts',(-0.611053009764407,0.426228370664493,
-2.82002149626745));
#70267=CARTESIAN_POINT('Ctrl Pts',(-0.740405689960357,0.0828042526237523,
-2.80417938283922));
#70268=CARTESIAN_POINT('Ctrl Pts',(-0.690114368206497,-0.280712139458959,
-2.78833726941098));
#70269=CARTESIAN_POINT('Ctrl Pts',(-0.472381262732657,-0.576118812396181,
-2.77249515598275));
#70270=CARTESIAN_POINT('Ctrl Pts',(-0.140034714193347,-0.731742714188332,
-2.75665304255451));
#70271=CARTESIAN_POINT('Ctrl Pts',(0.226288320465609,-0.709824351993689,
-2.74081092912627));
#70272=CARTESIAN_POINT('Ctrl Pts',(0.537707232757668,-0.515682068306337,
-2.72496881569804));
#70273=CARTESIAN_POINT('Ctrl Pts',(0.718662734406186,-0.196420267701063,
-2.7091267022698));
#70274=CARTESIAN_POINT('Ctrl Pts',(0.725249762127042,0.170498773654849,
-2.69328458884157));
#70275=CARTESIAN_POINT('Ctrl Pts',(0.555870110050121,0.496049869048306,
-2.67744247541333));
#70276=CARTESIAN_POINT('Ctrl Pts',(0.251620207298818,0.701244836227764,
-2.6616003619851));
#70277=CARTESIAN_POINT('Ctrl Pts',(-0.113680073860222,0.736297420670501,
-2.64575824855686));
#70278=CARTESIAN_POINT('Ctrl Pts',(-0.451398263728168,0.59270284078174,
-2.62991613512863));
#70279=CARTESIAN_POINT('Ctrl Pts',(-0.679594110201831,0.305301319501937,
-2.61407402170039));
#70280=CARTESIAN_POINT('Ctrl Pts',(-0.742900665961364,-0.0561751791648646,
-2.59823190827216));
#70281=CARTESIAN_POINT('Ctrl Pts',(-0.625957919932414,-0.404021945800056,
-2.58238979484392));
#70282=CARTESIAN_POINT('Ctrl Pts',(-0.357139582461871,-0.653841241353458,
-2.56654768141569));
#70283=CARTESIAN_POINT('Ctrl Pts',(-0.00166879826366219,-0.745019640907262,
-2.55070556798745));
#70284=CARTESIAN_POINT('Ctrl Pts',(0.354206884915627,-0.655434613764092,
-2.53486345455922));
#70285=CARTESIAN_POINT('Ctrl Pts',(0.62414167905897,-0.40682209219302,-2.51902134113098));
#70286=CARTESIAN_POINT('Ctrl Pts',(0.742641554609368,-0.0595027024940923,
-2.50317922770275));
#70287=CARTESIAN_POINT('Ctrl Pts',(0.68095499631052,0.302253772907092,-2.48733711427451));
#70288=CARTESIAN_POINT('Ctrl Pts',(0.454048956775666,0.590674694808553,
-2.47149500084627));
#70289=CARTESIAN_POINT('Ctrl Pts',(0.116977438610447,0.73578076156752,-2.45565288741804));
#70290=CARTESIAN_POINT('Ctrl Pts',(-0.248476207343311,0.702365022350014,
-2.43981077398981));
#70291=CARTESIAN_POINT('Ctrl Pts',(-0.553642300816813,0.498535107071557,
-2.42396866056157));
#70292=CARTESIAN_POINT('Ctrl Pts',(-0.724478674665794,0.173746079642204,
-2.40812654713333));
#70293=CARTESIAN_POINT('Ctrl Pts',(-0.719535457435451,-0.193198798468575,
-2.3922844337051));
#70294=CARTESIAN_POINT('Ctrl Pts',(-0.540012017352549,-0.513268030712396,
-2.37644232027686));
#70295=CARTESIAN_POINT('Ctrl Pts',(-0.229465960721355,-0.708803515162537,
-2.36060020684863));
#70296=CARTESIAN_POINT('Ctrl Pts',(0.136755209826522,-0.73236265799251,
-2.34475809342039));
#70297=CARTESIAN_POINT('Ctrl Pts',(0.46979559023953,-0.578229326157051,
-2.32891597999216));
#70298=CARTESIAN_POINT('Ctrl Pts',(0.68884990090208,-0.283800747468612,
-2.31307386656392));
#70299=CARTESIAN_POINT('Ctrl Pts',(0.740769196926055,0.0794861442144139,
-2.29723175313569));
#70300=CARTESIAN_POINT('Ctrl Pts',(0.612956347514708,0.423487386208817,
-2.28138963970745));
#70301=CARTESIAN_POINT('Ctrl Pts',(0.336422466162267,0.664738275186441,
-2.26554752627922));
#70302=CARTESIAN_POINT('Ctrl Pts',(-0.0217372871444871,0.744704330982535,
-2.24970541285098));
#70303=CARTESIAN_POINT('Ctrl Pts',(-0.374622942566726,0.643983463405074,
-2.23386329942275));
#70304=CARTESIAN_POINT('Ctrl Pts',(-0.636614179759623,0.387013483441507,
-2.21802118599451));
#70305=CARTESIAN_POINT('Ctrl Pts',(-0.744144307044669,0.0361427797707638,
-2.20217907256628));
#70306=CARTESIAN_POINT('Ctrl Pts',(-0.67112338904648,-0.32349721314304,
-2.18633695913804));
#70307=CARTESIAN_POINT('Ctrl Pts',(-0.435268423593712,-0.604647376293648,
-2.17049484570981));
#70308=CARTESIAN_POINT('Ctrl Pts',(-0.0938046829146193,-0.739092505509178,
-2.15465273228157));
#70309=CARTESIAN_POINT('Ctrl Pts',(0.270418801260945,-0.694212303377822,
-2.13881061885333));
#70310=CARTESIAN_POINT('Ctrl Pts',(0.569030821679157,-0.480896011852553,
-2.1229685054251));
#70311=CARTESIAN_POINT('Ctrl Pts',(0.729579419882164,-0.150900365542804,
-2.10712639199686));
#70312=CARTESIAN_POINT('Ctrl Pts',(0.713110837909455,0.215708096956561,
-2.09128427856863));
#70313=CARTESIAN_POINT('Ctrl Pts',(0.523620832580449,0.529979503305841,
-2.07544216514039));
#70314=CARTESIAN_POINT('Ctrl Pts',(0.207085188711333,0.715662472715273,
-2.05960005171216));
#70315=CARTESIAN_POINT('Ctrl Pts',(-0.159695343051901,0.727704917974369,
-2.04375793828392));
#70316=CARTESIAN_POINT('Ctrl Pts',(-0.487729141363133,0.563184991722728,
-2.02791582485569));
#70317=CARTESIAN_POINT('Ctrl Pts',(-0.697425668993718,0.262020011573948,
-2.01207371142745));
#70318=CARTESIAN_POINT('Ctrl Pts',(-0.73790645130165,-0.102718641754811,
-1.99623159799922));
#70319=CARTESIAN_POINT('Ctrl Pts',(-0.599349673498601,-0.442534765994343,
-1.98038948457098));
#70320=CARTESIAN_POINT('Ctrl Pts',(-0.315373238492099,-0.674979089068359,
-1.96454737114274));
#70321=CARTESIAN_POINT('Ctrl Pts',(0.0451219138183706,-0.743653859755946,
-1.94870525771451));
#70322=CARTESIAN_POINT('Ctrl Pts',(0.394669177892695,-0.631896581932559,
-1.93286314428627));
#70323=CARTESIAN_POINT('Ctrl Pts',(0.648458224192572,-0.366822820600851,
-1.91702103085804));
#70324=CARTESIAN_POINT('Ctrl Pts',(0.744912451033229,-0.0127471774214454,
-1.90117891742981));
#70325=CARTESIAN_POINT('Ctrl Pts',(0.660629258524832,0.344421301631415,
-1.88533680400157));
#70326=CARTESIAN_POINT('Ctrl Pts',(0.416058199748869,0.618023158674719,
-1.86949469057334));
#70327=CARTESIAN_POINT('Ctrl Pts',(0.0705393245988857,0.741674628069264,
-1.8536525771451));
#70328=CARTESIAN_POINT('Ctrl Pts',(-0.292094441667422,0.685374268107247,
-1.83781046371687));
#70329=CARTESIAN_POINT('Ctrl Pts',(-0.583857603582913,0.462782183078569,
-1.82196835028863));
#70330=CARTESIAN_POINT('Ctrl Pts',(-0.733959934896726,0.127905684795247,
-1.80612623686039));
#70331=CARTESIAN_POINT('Ctrl Pts',(-0.705982245726471,-0.238004451545676,
-1.79028412343216));
#70332=CARTESIAN_POINT('Ctrl Pts',(-0.506712736931143,-0.546167787834743,
-1.77444201000392));
#70333=CARTESIAN_POINT('Ctrl Pts',(-0.184499985212165,-0.721814938674213,
-1.75859989657569));
#70334=CARTESIAN_POINT('Ctrl Pts',(0.182477827355149,-0.722328798235466,
-1.74275778314745));
#70335=CARTESIAN_POINT('Ctrl Pts',(0.505181213365562,-0.547584689248198,
-1.72691566971922));
#70336=CARTESIAN_POINT('Ctrl Pts',(0.7053129485992,-0.239980613331262,-1.71107355629098));
#70337=CARTESIAN_POINT('Ctrl Pts',(0.734315255151018,0.125849736944674,
-1.69523144286275));
#70338=CARTESIAN_POINT('Ctrl Pts',(0.585151330193947,0.461145281889343,
-1.67938932943451));
#70339=CARTESIAN_POINT('Ctrl Pts',(0.294012678943567,0.684553573401655,
-1.66354721600628));
#70340=CARTESIAN_POINT('Ctrl Pts',(-0.0684619967945975,0.741869264245018,
-1.64770510257804));
#70341=CARTESIAN_POINT('Ctrl Pts',(-0.414325801541176,0.619185901336431,
-1.6318629891498));
#70342=CARTESIAN_POINT('Ctrl Pts',(-0.659662120089326,0.346270035601989,
-1.61602087572157));
#70343=CARTESIAN_POINT('Ctrl Pts',(-0.744945228274433,-0.0106610087561992,
-1.60017876229333));
#70344=CARTESIAN_POINT('Ctrl Pts',(-0.649482964398754,-0.365005382415594,
-1.5843366488651));
#70345=CARTESIAN_POINT('Ctrl Pts',(-0.396437249294967,-0.630788837574024,
-1.56849453543686));
#70346=CARTESIAN_POINT('Ctrl Pts',(-0.0472043308869144,-0.743524580213772,
-1.55265242200863));
#70347=CARTESIAN_POINT('Ctrl Pts',(0.3134817306855,-0.675859641318353,-1.53681030858039));
#70348=CARTESIAN_POINT('Ctrl Pts',(0.59810800974443,-0.444211502458123,
-1.52096819515216));
#70349=CARTESIAN_POINT('Ctrl Pts',(0.737615895328708,-0.104784737414259,
-1.50512608172392));
#70350=CARTESIAN_POINT('Ctrl Pts',(0.698156718129113,0.260065851598656,
-1.48928396829569));
#70351=CARTESIAN_POINT('Ctrl Pts',(0.489304421830971,0.561816903459843,
-1.47344185486745));
#70352=CARTESIAN_POINT('Ctrl Pts',(0.161732646008563,0.727254839414366,
-1.45759974143922));
#70353=CARTESIAN_POINT('Ctrl Pts',(-0.20508017219881,0.716239606003086,
-1.44175762801098));
#70354=CARTESIAN_POINT('Ctrl Pts',(-0.52213457781493,0.531443819125382,
-1.42591551458275));
#70355=CARTESIAN_POINT('Ctrl Pts',(-0.712503953510709,0.217704309714247,
-1.41007340115451));
#70356=CARTESIAN_POINT('Ctrl Pts',(-0.729999153650814,-0.148856595102944,
-1.39423128772627));
#70357=CARTESIAN_POINT('Ctrl Pts',(-0.570375333998946,-0.479300561862948,
-1.37838917429804));
#70358=CARTESIAN_POINT('Ctrl Pts',(-0.272361874350678,-0.693452276394514,
-1.3625470608698));
#70359=CARTESIAN_POINT('Ctrl Pts',(0.091734495082405,-0.739352306176509,
-1.34670494744157));
#70360=CARTESIAN_POINT('Ctrl Pts',(0.433573408778929,-0.60586396941588,
-1.33086283401333));
#70361=CARTESIAN_POINT('Ctrl Pts',(0.67021480712666,-0.325375417855625,
-1.3150207205851));
#70362=CARTESIAN_POINT('Ctrl Pts',(0.744242606411063,0.0340586705409123,
-1.29917860715686));
#70363=CARTESIAN_POINT('Ctrl Pts',(0.63769551012784,0.385229135190137,-1.28333649372863));
#70364=CARTESIAN_POINT('Ctrl Pts',(0.376424941749179,0.64293181089885,-1.26749438030039));
#70365=CARTESIAN_POINT('Ctrl Pts',(0.0238227377454225,0.744640535696828,
-1.25165226687216));
#70366=CARTESIAN_POINT('Ctrl Pts',(-0.334559555094233,0.665677815712449,
-1.23581015344392));
#70367=CARTESIAN_POINT('Ctrl Pts',(-0.611767972369815,0.425202302697283,
-1.21996804001569));
#70368=CARTESIAN_POINT('Ctrl Pts',(-0.740543692067099,0.0815603480631216,
-1.20412592658745));
#70369=CARTESIAN_POINT('Ctrl Pts',(-0.689641980364514,-0.281870518421948,
-1.18828381315922));
#70370=CARTESIAN_POINT('Ctrl Pts',(-0.471413072515636,-0.576911401601594,
-1.17244169973098));
#70371=CARTESIAN_POINT('Ctrl Pts',(-0.138805646686953,-0.731976804744769,
-1.15659958630274));
#70372=CARTESIAN_POINT('Ctrl Pts',(0.227480064876487,-0.709443352439317,
-1.14075747287451));
#70373=CARTESIAN_POINT('Ctrl Pts',(0.538572498596197,-0.514778315386726,
-1.12491535944627));
#70374=CARTESIAN_POINT('Ctrl Pts',(0.718991584872685,-0.195213091566146,
-1.10907324601804));
#70375=CARTESIAN_POINT('Ctrl Pts',(0.724962407593727,0.171716504193551,
-1.0932311325898));
#70376=CARTESIAN_POINT('Ctrl Pts',(0.555036271562332,0.496982683286584,
-1.07738901916157));
#70377=CARTESIAN_POINT('Ctrl Pts',(0.250442198073112,0.701666413376653,
-1.06154690573333));
#70378=CARTESIAN_POINT('Ctrl Pts',(-0.11491643440966,0.736105470254853,
-1.0457047923051));
#70379=CARTESIAN_POINT('Ctrl Pts',(-0.452392998647782,0.591943937388512,
-1.02986267887686));
#70380=CARTESIAN_POINT('Ctrl Pts',(-0.680105867845271,0.304159594224771,
-1.01402056544863));
#70381=CARTESIAN_POINT('Ctrl Pts',(-0.742805279061213,-0.0574227101009686,
-0.998178452020394));
#70382=CARTESIAN_POINT('Ctrl Pts',(-0.625278532115667,-0.40507259536017,
-0.982336338592156));
#70383=CARTESIAN_POINT('Ctrl Pts',(-0.356041032970718,-0.654440091282382,
-0.966494225163925));
#70384=CARTESIAN_POINT('Ctrl Pts',(-0.000417627143387664,-0.745021392863397,
-0.950652111735685));
#70385=CARTESIAN_POINT('Ctrl Pts',(0.355307107171661,-0.654838842639816,
-0.934809998307453));
#70386=CARTESIAN_POINT('Ctrl Pts',(0.624824006542467,-0.405773349401816,
-0.918967884879216));
#70387=CARTESIAN_POINT('Ctrl Pts',(0.742740434833499,-0.0582554435215241,
-0.903125771450982));
#70388=CARTESIAN_POINT('Ctrl Pts',(0.680446438058071,0.303396926765304,
-0.887283658022746));
#70389=CARTESIAN_POINT('Ctrl Pts',(0.453056351065208,0.591436381190763,
-0.871441544594511));
#70390=CARTESIAN_POINT('Ctrl Pts',(0.115741620447917,0.735976173209866,
-0.855599431166276));
#70391=CARTESIAN_POINT('Ctrl Pts',(-0.24965539253963,0.701946746706922,
-0.839757317738039));
#70392=CARTESIAN_POINT('Ctrl Pts',(-0.55447874843284,0.497604629975343,
-0.823915204309805));
#70393=CARTESIAN_POINT('Ctrl Pts',(-0.724769438189725,0.172529161890676,
-0.808073090881569));
#70394=CARTESIAN_POINT('Ctrl Pts',(-0.71920998918227,-0.194406897246436,
-0.792230977453334));
#70395=CARTESIAN_POINT('Ctrl Pts',(-0.539149285383643,-0.514174190626926,
-0.776388864025099));
#70396=CARTESIAN_POINT('Ctrl Pts',(-0.228275288896775,-0.709187875471401,
-0.760546750596862));
#70397=CARTESIAN_POINT('Ctrl Pts',(0.13798492990271,-0.732131961709289,
-0.74470463716863));
#70398=CARTESIAN_POINT('Ctrl Pts',(0.470765992722073,-0.577439546907681,
-0.728862523740392));
#70399=CARTESIAN_POINT('Ctrl Pts',(0.689325537933745,-0.282643508662239,
-0.713020410312158));
#70400=CARTESIAN_POINT('Ctrl Pts',(0.740634665133557,0.0807300627960256,
-0.697178296883922));
#70401=CARTESIAN_POINT('Ctrl Pts',(0.61224428822249,0.424516173750169,-0.681336183455687));
#70402=CARTESIAN_POINT('Ctrl Pts',(0.335305645658125,0.665302317917453,
-0.665494070027452));
#70403=CARTESIAN_POINT('Ctrl Pts',(-0.022987895734092,0.744666775736816,
-0.649651956599217));
#70404=CARTESIAN_POINT('Ctrl Pts',(-0.375703905235841,0.643353422177177,
-0.633809843170981));
#70405=CARTESIAN_POINT('Ctrl Pts',(-0.637263223535151,0.38594382255211,
-0.617967729742746));
#70406=CARTESIAN_POINT('Ctrl Pts',(-0.744203955035377,0.0348930300525936,
-0.602125616314511));
#70407=CARTESIAN_POINT('Ctrl Pts',(-0.670579168915521,-0.324623826071213,
-0.586283502886275));
#70408=CARTESIAN_POINT('Ctrl Pts',(-0.434252378968355,-0.605377503378576,
-0.570441389458041));
#70409=CARTESIAN_POINT('Ctrl Pts',(-0.0925633357629972,-0.739248996691216,
-0.554599276029804));
#70410=CARTESIAN_POINT('Ctrl Pts',(0.271584264026978,-0.693757189346148,
-0.53875716260157));
#70411=CARTESIAN_POINT('Ctrl Pts',(0.569837624906181,-0.479939716503923,
-0.522915049173334));
#70412=CARTESIAN_POINT('Ctrl Pts',(0.729831809648918,-0.149674913933615,
-0.507072935745098));
#70413=CARTESIAN_POINT('Ctrl Pts',(0.712747577120447,0.216905374635287,
-0.491230822316864));
#70414=CARTESIAN_POINT('Ctrl Pts',(0.522730058864535,0.530858112677697,
-0.475388708888629));
#70415=CARTESIAN_POINT('Ctrl Pts',(0.205883029672815,0.716009237600728,
-0.459546595460393));
#70416=CARTESIAN_POINT('Ctrl Pts',(-0.160917208679019,0.727435703129611,
-0.443704482032157));
#70417=CARTESIAN_POINT('Ctrl Pts',(-0.488674253447083,0.562365116497098,
-0.427862368603923));
#70418=CARTESIAN_POINT('Ctrl Pts',(-0.697864715871596,0.260848401534634,
-0.412020255175687));
#70419=CARTESIAN_POINT('Ctrl Pts',(-0.737732907419063,-0.103957719945394,
-0.396178141747452));
#70420=CARTESIAN_POINT('Ctrl Pts',(-0.598605645679325,-0.443540675943605,
-0.380336028319217));
#70421=CARTESIAN_POINT('Ctrl Pts',(-0.314239249455351,-0.675507767768747,
-0.364493914890981));
#70422=CARTESIAN_POINT('Ctrl Pts',(0.0463707252377993,-0.743577034395874,
-0.348651801462746));
#70423=CARTESIAN_POINT('Ctrl Pts',(0.395729813976248,-0.631232892553112,
-0.33280968803451));
#70424=CARTESIAN_POINT('Ctrl Pts',(0.649073343313576,-0.365733297591681,
-0.316967574606276));
#70425=CARTESIAN_POINT('Ctrl Pts',(0.744932808338686,-0.0114961706467306,
-0.30112546117804));
#70426=CARTESIAN_POINT('Ctrl Pts',(0.660049912914123,0.345530261365429,
-0.285283347749805));
#70427=CARTESIAN_POINT('Ctrl Pts',(0.415019720896205,0.61872100586388,-0.269441234321569));
#70428=CARTESIAN_POINT('Ctrl Pts',(0.0692936706342567,0.741792043967289,
-0.253599120893334));
#70429=CARTESIAN_POINT('Ctrl Pts',(-0.293245025070179,0.684882765631844,
-0.237757007465099));
#70430=CARTESIAN_POINT('Ctrl Pts',(-0.584633978526232,0.461801012217599,
-0.221914894036864));
#70431=CARTESIAN_POINT('Ctrl Pts',(-0.734173677083153,0.12667291162916,
-0.206072780608629));
#70432=CARTESIAN_POINT('Ctrl Pts',(-0.705581599416755,-0.23918973119976,
-0.190230667180393));
#70433=CARTESIAN_POINT('Ctrl Pts',(-0.505794705825495,-0.547017969482345,
-0.174388553752158));
#70434=CARTESIAN_POINT('Ctrl Pts',(-0.183287712150819,-0.72212378510834,
-0.158546440323923));
#70435=CARTESIAN_POINT('Ctrl Pts',(0.183690998201556,-0.722021292731707,
-0.142704326895687));
#70436=CARTESIAN_POINT('Ctrl Pts',(0.506099384029242,-0.546735601718665,
-0.126862213467452));
#70437=CARTESIAN_POINT('Ctrl Pts',(0.705716381011111,-0.238795642840187,
-0.111020100039217));
#70438=CARTESIAN_POINT('Ctrl Pts',(0.734100104964976,0.127082465415513,
-0.0951779866109815));
#70439=CARTESIAN_POINT('Ctrl Pts',(0.584381497914616,0.462127882429814,
-0.0793358731827458));
#70440=CARTESIAN_POINT('Ctrl Pts',(0.29285195986455,0.685045268305722,-0.063493759754511));
#70441=CARTESIAN_POINT('Ctrl Pts',(-0.0696865334553906,0.741755360583931,
-0.0476516463262754));
#70442=CARTESIAN_POINT('Ctrl Pts',(-0.415409884379656,0.618485487271467,
-0.03180953289804));
#70443=CARTESIAN_POINT('Ctrl Pts',(-0.578548277620789,0.436270642466983,
-0.0212481239458833));
#70444=CARTESIAN_POINT('Ctrl Pts',(-0.633489757430006,0.33117581686427,
-0.0159674194698048));
#70445=CARTESIAN_POINT('Ctrl Pts',(0.392888236737278,-0.550964357679762,
-2.9089));
#70446=CARTESIAN_POINT('Ctrl Pts',(0.484292245096581,-0.485784897022383,
-2.90361929552392));
#70447=CARTESIAN_POINT('Ctrl Pts',(0.633945837478465,-0.309125594940106,
-2.89305788657177));
#70448=CARTESIAN_POINT('Ctrl Pts',(0.704592787855342,0.0310787463577468,
-2.87721577314353));
#70449=CARTESIAN_POINT('Ctrl Pts',(0.604289094090405,0.363654317141465,
-2.8613736597153));
#70450=CARTESIAN_POINT('Ctrl Pts',(0.357365708044879,0.608039989146884,
-2.84553154628705));
#70451=CARTESIAN_POINT('Ctrl Pts',(0.0237357764082632,0.704875616667608,
-2.82968943285883));
#70452=CARTESIAN_POINT('Ctrl Pts',(-0.315653531008585,0.630699052042456,
-2.81384731943059));
#70453=CARTESIAN_POINT('Ctrl Pts',(-0.578455917520507,0.403490890783857,
-2.79800520600235));
#70454=CARTESIAN_POINT('Ctrl Pts',(-0.700908179616937,0.0783869961536362,
-2.78216309257412));
#70455=CARTESIAN_POINT('Ctrl Pts',(-0.653299687058058,-0.26573733472401,
-2.76632097914588));
#70456=CARTESIAN_POINT('Ctrl Pts',(-0.447181721367947,-0.545385311748889,
-2.75047886571765));
#70457=CARTESIAN_POINT('Ctrl Pts',(-0.132564454783822,-0.692707336942753,
-2.73463675228941));
#70458=CARTESIAN_POINT('Ctrl Pts',(0.214216796165651,-0.67195822661804,
-2.71879463886118));
#70459=CARTESIAN_POINT('Ctrl Pts',(0.509022827335671,-0.488172612202699,
-2.70295252543294));
#70460=CARTESIAN_POINT('Ctrl Pts',(0.680325118730706,-0.185942077621786,
-2.68711041200471));
#70461=CARTESIAN_POINT('Ctrl Pts',(0.686560756397345,0.161403385589515,
-2.67126829857647));
#70462=CARTESIAN_POINT('Ctrl Pts',(0.526216791985425,0.469587707696419,
-2.65542618514823));
#70463=CARTESIAN_POINT('Ctrl Pts',(0.238197334034658,0.663836391711814,
-2.63958407172001));
#70464=CARTESIAN_POINT('Ctrl Pts',(-0.107615722986078,0.697019069108502,
-2.62374195829176));
#70465=CARTESIAN_POINT('Ctrl Pts',(-0.427318076565427,0.561084652399629,
-2.60789984486353));
#70466=CARTESIAN_POINT('Ctrl Pts',(-0.643340640298785,0.28901478606709,
-2.59205773143529));
#70467=CARTESIAN_POINT('Ctrl Pts',(-0.703270059206417,-0.0531784710760548,
-2.57621561800706));
#70468=CARTESIAN_POINT('Ctrl Pts',(-0.592565713804986,-0.382469084713778,
-2.56037350457882));
#70469=CARTESIAN_POINT('Ctrl Pts',(-0.338087697064974,-0.618961578023624,
-2.54453139115059));
#70470=CARTESIAN_POINT('Ctrl Pts',(-0.00157977493823928,-0.705275995805936,
-2.52868927772235));
#70471=CARTESIAN_POINT('Ctrl Pts',(0.335311446522369,-0.62046995075891,
-2.51284716429412));
#70472=CARTESIAN_POINT('Ctrl Pts',(0.590846361696255,-0.385119855146208,
-2.49700505086588));
#70473=CARTESIAN_POINT('Ctrl Pts',(0.703024770348556,-0.0563284851169273,
-2.48116293743765));
#70474=CARTESIAN_POINT('Ctrl Pts',(0.644628928892509,0.286129813186614,
-2.46532082400941));
#70475=CARTESIAN_POINT('Ctrl Pts',(0.429827366355921,0.559164699431498,
-2.44947871058118));
#70476=CARTESIAN_POINT('Ctrl Pts',(0.110737187280514,0.696529971582292,
-2.43363659715294));
#70477=CARTESIAN_POINT('Ctrl Pts',(-0.235221053172144,0.664896820644794,
-2.41779448372471));
#70478=CARTESIAN_POINT('Ctrl Pts',(-0.524107826947175,0.471940368788045,
-2.40195237029647));
#70479=CARTESIAN_POINT('Ctrl Pts',(-0.685830803189103,0.164477461544244,
-2.38611025686824));
#70480=CARTESIAN_POINT('Ctrl Pts',(-0.681151285679508,-0.182892460140387,
-2.37026814344));
#70481=CARTESIAN_POINT('Ctrl Pts',(-0.511204661425697,-0.485887353298784,
-2.35442603001177));
#70482=CARTESIAN_POINT('Ctrl Pts',(-0.217224922760744,-0.6709918471119,
-2.33858391658353));
#70483=CARTESIAN_POINT('Ctrl Pts',(0.129459898096913,-0.693294209368428,
-2.32274180315529));
#70484=CARTESIAN_POINT('Ctrl Pts',(0.4447339835604,-0.54738323853179,-2.30689968972706));
#70485=CARTESIAN_POINT('Ctrl Pts',(0.652102673733417,-0.268661178566577,
-2.29105757629882));
#70486=CARTESIAN_POINT('Ctrl Pts',(0.701252295024287,0.0752458947865185,
-2.27521546287059));
#70487=CARTESIAN_POINT('Ctrl Pts',(0.580257720256285,0.400896126249721,
-2.25937334944235));
#70488=CARTESIAN_POINT('Ctrl Pts',(0.318475751250181,0.629277301215201,
-2.24353123601412));
#70489=CARTESIAN_POINT('Ctrl Pts',(-0.0205776948622204,0.70497750633138,
-2.22768912258588));
#70490=CARTESIAN_POINT('Ctrl Pts',(-0.354638393893549,0.609629670813075,
-2.21184700915765));
#70491=CARTESIAN_POINT('Ctrl Pts',(-0.602653507265104,0.366367951846396,
-2.19600489572941));
#70492=CARTESIAN_POINT('Ctrl Pts',(-0.704447357300714,0.0342147154174032,
-2.18016278230118));
#70493=CARTESIAN_POINT('Ctrl Pts',(-0.635321796271045,-0.306240005783024,
-2.16432066887294));
#70494=CARTESIAN_POINT('Ctrl Pts',(-0.412048695144598,-0.572391997488336,
-2.14847855544471));
#70495=CARTESIAN_POINT('Ctrl Pts',(-0.0888006000396183,-0.699665047999155,
-2.13263644201647));
#70496=CARTESIAN_POINT('Ctrl Pts',(0.255993102559969,-0.657179014729453,
-2.11679432858824));
#70497=CARTESIAN_POINT('Ctrl Pts',(0.538675435341973,-0.455242244654634,
-2.10095221516));
#70498=CARTESIAN_POINT('Ctrl Pts',(0.690659445233286,-0.142850469614568,
-2.08511010173177));
#70499=CARTESIAN_POINT('Ctrl Pts',(0.675069392417806,0.204200982807891,
-2.06926798830353));
#70500=CARTESIAN_POINT('Ctrl Pts',(0.495687876997698,0.501707339548235,
-2.0534258748753));
#70501=CARTESIAN_POINT('Ctrl Pts',(0.196038070227499,0.67748490830463,-2.03758376144706));
#70502=CARTESIAN_POINT('Ctrl Pts',(-0.151176272291756,0.688884940069836,
-2.02174164801882));
#70503=CARTESIAN_POINT('Ctrl Pts',(-0.461710855621964,0.533141455675591,
-2.00589953459059));
#70504=CARTESIAN_POINT('Ctrl Pts',(-0.660220960887921,0.24804235276114,
-1.99005742116235));
#70505=CARTESIAN_POINT('Ctrl Pts',(-0.698542264764505,-0.0972390368973889,
-1.97421530773412));
#70506=CARTESIAN_POINT('Ctrl Pts',(-0.567376904718818,-0.418927408927545,
-1.95837319430588));
#70507=CARTESIAN_POINT('Ctrl Pts',(-0.298549410801028,-0.638971811013141,
-1.94253108087765));
#70508=CARTESIAN_POINT('Ctrl Pts',(0.0427148506610781,-0.703983073299391,
-1.92668896744941));
#70509=CARTESIAN_POINT('Ctrl Pts',(0.373615247395648,-0.598187573318388,
-1.91084685402117));
#70510=CARTESIAN_POINT('Ctrl Pts',(0.613865722048657,-0.347254375426338,
-1.89500474059294));
#70511=CARTESIAN_POINT('Ctrl Pts',(0.705174524058082,-0.0120671694489478,
-1.87916262716471));
#70512=CARTESIAN_POINT('Ctrl Pts',(0.625387483204131,0.326047882696172,
-1.86332051373647));
#70513=CARTESIAN_POINT('Ctrl Pts',(0.393863255448903,0.585054238482422,
-1.84747840030823));
#70514=CARTESIAN_POINT('Ctrl Pts',(0.0667763501367175,0.702109425247569,
-1.83163628688));
#70515=CARTESIAN_POINT('Ctrl Pts',(-0.276512439276773,0.648812451240159,
-1.81579417345177));
#70516=CARTESIAN_POINT('Ctrl Pts',(-0.552711271174482,0.438094711992443,
-1.79995206002353));
#70517=CARTESIAN_POINT('Ctrl Pts',(-0.69480627830909,0.121082457777023,
-1.78410994659529));
#70518=CARTESIAN_POINT('Ctrl Pts',(-0.668321080461322,-0.225307921232401,
-1.76826783316706));
#70519=CARTESIAN_POINT('Ctrl Pts',(-0.479681756700353,-0.517032047602386,
-1.75242571973882));
#70520=CARTESIAN_POINT('Ctrl Pts',(-0.174657691759948,-0.683309166240393,
-1.73658360631059));
#70521=CARTESIAN_POINT('Ctrl Pts',(0.172743407467333,-0.683795613568578,
-1.72074149288235));
#70522=CARTESIAN_POINT('Ctrl Pts',(0.478231933435968,-0.518373363321409,
-1.70489937945412));
#70523=CARTESIAN_POINT('Ctrl Pts',(0.667687487503493,-0.227178663149353,
-1.68905726602588));
#70524=CARTESIAN_POINT('Ctrl Pts',(0.695142643731443,0.119136186044015,
-1.67321515259765));
#70525=CARTESIAN_POINT('Ctrl Pts',(0.553935982945549,0.436545132554703,
-1.65737303916941));
#70526=CARTESIAN_POINT('Ctrl Pts',(0.278328346711741,0.648035537124133,
-1.64153092574118));
#70527=CARTESIAN_POINT('Ctrl Pts',(-0.0648098389800511,0.702293678406998,
-1.62568881231294));
#70528=CARTESIAN_POINT('Ctrl Pts',(-0.392223273354511,0.58615495374357,
-1.60984669888471));
#70529=CARTESIAN_POINT('Ctrl Pts',(-0.624471937511469,0.327797994532801,
-1.59400458545647));
#70530=CARTESIAN_POINT('Ctrl Pts',(-0.705205552772174,-0.0100922890538433,
-1.57816247202824));
#70531=CARTESIAN_POINT('Ctrl Pts',(-0.614835796701285,-0.345533889877317,
-1.5623203586));
#70532=CARTESIAN_POINT('Ctrl Pts',(-0.375288999670649,-0.597138922433682,
-1.54647824517177));
#70533=CARTESIAN_POINT('Ctrl Pts',(-0.0446861795912879,-0.703860690273713,
-1.53063613174353));
#70534=CARTESIAN_POINT('Ctrl Pts',(0.296758806931518,-0.639805389526875,
-1.5147940183153));
#70535=CARTESIAN_POINT('Ctrl Pts',(0.566201478471519,-0.420514698596517,
-1.49895190488706));
#70536=CARTESIAN_POINT('Ctrl Pts',(0.698267208723158,-0.0991949150966095,
-1.48310979145883));
#70537=CARTESIAN_POINT('Ctrl Pts',(0.660913011645563,0.246192438951009,
-1.46726767803059));
#70538=CARTESIAN_POINT('Ctrl Pts',(0.46320210154304,0.53184634913212,-1.45142556460235));
#70539=CARTESIAN_POINT('Ctrl Pts',(0.153104893757042,0.688458871296389,
-1.43558345117412));
#70540=CARTESIAN_POINT('Ctrl Pts',(-0.194140012861185,0.678031253973823,
-1.41974133774588));
#70541=CARTESIAN_POINT('Ctrl Pts',(-0.494280907634458,0.503093540315427,
-1.40389922431765));
#70542=CARTESIAN_POINT('Ctrl Pts',(-0.674494882733548,0.206090706062433,
-1.38805711088941));
#70543=CARTESIAN_POINT('Ctrl Pts',(-0.691056787981589,-0.140915725678943,
-1.37221499746118));
#70544=CARTESIAN_POINT('Ctrl Pts',(-0.539948223619144,-0.453731905170425,
-1.35637288403294));
#70545=CARTESIAN_POINT('Ctrl Pts',(-0.257832520922968,-0.65645953196946,
-1.34053077060471));
#70546=CARTESIAN_POINT('Ctrl Pts',(0.0868408479677307,-0.699910989400294,
-1.32468865717647));
#70547=CARTESIAN_POINT('Ctrl Pts',(0.4104441021973,-0.57354369051582,-1.30884654374824));
#70548=CARTESIAN_POINT('Ctrl Pts',(0.634461683351754,-0.308018016222288,
-1.29300443032));
#70549=CARTESIAN_POINT('Ctrl Pts',(0.70454041281189,0.0322417845955294,
-1.27716231689176));
#70550=CARTESIAN_POINT('Ctrl Pts',(0.603677153234099,0.364678791023317,
-1.26132020346353));
#70551=CARTESIAN_POINT('Ctrl Pts',(0.356344264045233,0.608634119517723,
-1.2454780900353));
#70552=CARTESIAN_POINT('Ctrl Pts',(0.022551895498706,0.7049171142542,-1.22963597660706));
#70553=CARTESIAN_POINT('Ctrl Pts',(-0.316712218604248,0.630166721230049,
-1.21379386317883));
#70554=CARTESIAN_POINT('Ctrl Pts',(-0.579132739896463,0.402519559200629,
-1.19795174975059));
#70555=CARTESIAN_POINT('Ctrl Pts',(-0.701038819895276,0.0772094486374146,
-1.18210963632235));
#70556=CARTESIAN_POINT('Ctrl Pts',(-0.652852499108416,-0.2668339190713,
-1.16626752289412));
#70557=CARTESIAN_POINT('Ctrl Pts',(-0.446265180001859,-0.546135619674237,
-1.15042540946588));
#70558=CARTESIAN_POINT('Ctrl Pts',(-0.13140095282778,-0.692928939758619,
-1.13458329603765));
#70559=CARTESIAN_POINT('Ctrl Pts',(0.215344966055381,-0.671597551777596,
-1.11874118260941));
#70560=CARTESIAN_POINT('Ctrl Pts',(0.509841934903309,-0.487317070676889,
-1.10289906918118));
#70561=CARTESIAN_POINT('Ctrl Pts',(0.680636426416433,-0.184799299225192,
-1.08705695575294));
#70562=CARTESIAN_POINT('Ctrl Pts',(0.686288731012368,0.162556155357116,
-1.07121484232471));
#70563=CARTESIAN_POINT('Ctrl Pts',(0.52542743525236,0.470470760242527,-1.05537272889647));
#70564=CARTESIAN_POINT('Ctrl Pts',(0.237082166616096,0.664235479503821,
-1.03953061546824));
#70565=CARTESIAN_POINT('Ctrl Pts',(-0.108786128932179,0.696837358435242,
-1.02368850204));
#70566=CARTESIAN_POINT('Ctrl Pts',(-0.428259746586556,0.560366233290937,
-1.00784638861177));
#70567=CARTESIAN_POINT('Ctrl Pts',(-0.643825097837578,0.287933967001959,
-0.99200427518353));
#70568=CARTESIAN_POINT('Ctrl Pts',(-0.703179760793738,-0.0543594515159633,
-0.976162161755296));
#70569=CARTESIAN_POINT('Ctrl Pts',(-0.591922568453257,-0.383463686565954,
-0.960320048327059));
#70570=CARTESIAN_POINT('Ctrl Pts',(-0.337047750540382,-0.619528481843024,
-0.944477934898826));
#70571=CARTESIAN_POINT('Ctrl Pts',(-0.000395348502580347,-0.705277654302627,
-0.928635821470588));
#70572=CARTESIAN_POINT('Ctrl Pts',(0.336352976576915,-0.619905961502954,
-0.912793708042355));
#70573=CARTESIAN_POINT('Ctrl Pts',(0.59149228989595,-0.384127058344892,
-0.896951594614118));
#70574=CARTESIAN_POINT('Ctrl Pts',(0.703118375731167,-0.0551477621324492,
-0.881109481185884));
#70575=CARTESIAN_POINT('Ctrl Pts',(0.644147500070733,0.287211984624038,
-0.865267367757648));
#70576=CARTESIAN_POINT('Ctrl Pts',(0.428887711959651,0.559885753068489,
-0.849425254329413));
#70577=CARTESIAN_POINT('Ctrl Pts',(0.109567294787274,0.696714958840452,
-0.833583140901177));
#70578=CARTESIAN_POINT('Ctrl Pts',(-0.236337333828263,0.664500858237221,
-0.817741027472942));
#70579=CARTESIAN_POINT('Ctrl Pts',(-0.524899653622529,0.471059528707363,
-0.801898914044707));
#70580=CARTESIAN_POINT('Ctrl Pts',(-0.686106055709472,0.163325461205062,
-0.786056800616471));
#70581=CARTESIAN_POINT('Ctrl Pts',(-0.680843179780333,-0.184036111960829,
-0.770214687188236));
#70582=CARTESIAN_POINT('Ctrl Pts',(-0.510387952556461,-0.48674517341652,
-0.754372573760001));
#70583=CARTESIAN_POINT('Ctrl Pts',(-0.216097768239373,-0.671355703424805,
-0.738530460331765));
#70584=CARTESIAN_POINT('Ctrl Pts',(0.13062401781091,-0.693075819755666,
-0.722688346903532));
#70585=CARTESIAN_POINT('Ctrl Pts',(0.445652619177005,-0.546635590663221,
-0.706846233475294));
#70586=CARTESIAN_POINT('Ctrl Pts',(0.652552937542223,-0.267565673553371,
-0.69100412004706));
#70587=CARTESIAN_POINT('Ctrl Pts',(0.701124939933614,0.0764234555757611,
-0.675162006618824));
#70588=CARTESIAN_POINT('Ctrl Pts',(0.579583646314047,0.401870032329318,
-0.659319893190589));
#70589=CARTESIAN_POINT('Ctrl Pts',(0.317418508393823,0.629811254653404,
-0.643477779762354));
#70590=CARTESIAN_POINT('Ctrl Pts',(-0.0217615887758392,0.704941954499094,
-0.627635666334118));
#70591=CARTESIAN_POINT('Ctrl Pts',(-0.355661691778637,0.609033239618506,
-0.611793552905885));
#70592=CARTESIAN_POINT('Ctrl Pts',(-0.603267927301802,0.365355352838904,
-0.595951439477647));
#70593=CARTESIAN_POINT('Ctrl Pts',(-0.704503823323535,0.0330316345580622,
-0.580109326049413));
#70594=CARTESIAN_POINT('Ctrl Pts',(-0.634806607981066,-0.307306518679029,
-0.564267212621177));
#70595=CARTESIAN_POINT('Ctrl Pts',(-0.411086852200351,-0.573083175383003,
-0.548425099192943));
#70596=CARTESIAN_POINT('Ctrl Pts',(-0.0876254735054571,-0.699813191038862,
-0.532582985764706));
#70597=CARTESIAN_POINT('Ctrl Pts',(0.257096392819387,-0.656748179105437,
-0.516740872336472));
#70598=CARTESIAN_POINT('Ctrl Pts',(0.539439199031029,-0.454336963616046,
-0.500898758908236));
#70599=CARTESIAN_POINT('Ctrl Pts',(0.690898371074035,-0.141690390662916,
-0.485056645480001));
#70600=CARTESIAN_POINT('Ctrl Pts',(0.67472551005466,0.205334390789043,-0.469214532051766));
#70601=CARTESIAN_POINT('Ctrl Pts',(0.494844622289992,0.502539078828164,
-0.45337241862353));
#70602=CARTESIAN_POINT('Ctrl Pts',(0.194900041286442,0.67781317475087,-0.437530305195295));
#70603=CARTESIAN_POINT('Ctrl Pts',(-0.152332956558304,0.688630086697795,
-0.42168819176706));
#70604=CARTESIAN_POINT('Ctrl Pts',(-0.462605549975718,0.532365317323737,
-0.405846078338825));
#70605=CARTESIAN_POINT('Ctrl Pts',(-0.660636586472805,0.246933243159456,
-0.390003964910589));
#70606=CARTESIAN_POINT('Ctrl Pts',(-0.698377978713657,-0.0984120155099795,
-0.374161851482354));
#70607=CARTESIAN_POINT('Ctrl Pts',(-0.566672567635157,-0.419879657837779,
-0.358319738054119));
#70608=CARTESIAN_POINT('Ctrl Pts',(-0.297475915280626,-0.639472286942102,
-0.342477624625884));
#70609=CARTESIAN_POINT('Ctrl Pts',(0.043897043275945,-0.703910346247173,
-0.326635511197648));
#70610=CARTESIAN_POINT('Ctrl Pts',(0.374619303032495,-0.597559288958764,
-0.310793397769413));
#70611=CARTESIAN_POINT('Ctrl Pts',(0.614448027167589,-0.346222973859112,
-0.294951284341178));
#70612=CARTESIAN_POINT('Ctrl Pts',(0.70519379538744,-0.0108828985917093,
-0.279109170912942));
#70613=CARTESIAN_POINT('Ctrl Pts',(0.624839043230104,0.327097684121224,
-0.263267057484707));
#70614=CARTESIAN_POINT('Ctrl Pts',(0.392880175048439,0.585714858477159,
-0.247424944056472));
#70615=CARTESIAN_POINT('Ctrl Pts',(0.0655971465397984,0.70222057750431,
-0.231582830628236));
#70616=CARTESIAN_POINT('Ctrl Pts',(-0.277601643923981,0.6483471683419,-0.215740717200002));
#70617=CARTESIAN_POINT('Ctrl Pts',(-0.553446229800004,0.437165882444832,
-0.199898603771766));
#70618=CARTESIAN_POINT('Ctrl Pts',(-0.695008618254376,0.119915447842551,
-0.184056490343531));
#70619=CARTESIAN_POINT('Ctrl Pts',(-0.667941806936793,-0.226429971232753,
-0.168214376915295));
#70620=CARTESIAN_POINT('Ctrl Pts',(-0.478812698669308,-0.517836875656849,
-0.15237226348706));
#70621=CARTESIAN_POINT('Ctrl Pts',(-0.173510088336382,-0.683601537024222,
-0.136530150058825));
#70622=CARTESIAN_POINT('Ctrl Pts',(0.173891860782926,-0.683504512182157,
-0.120688036630589));
#70623=CARTESIAN_POINT('Ctrl Pts',(0.479101123580215,-0.517569571018445,
-0.104845923202354));
#70624=CARTESIAN_POINT('Ctrl Pts',(0.668069398503454,-0.226056905819471,
-0.0890038097741189));
#70625=CARTESIAN_POINT('Ctrl Pts',(0.694938970897365,0.12030315366754,-0.0731616963458836));
#70626=CARTESIAN_POINT('Ctrl Pts',(0.553207217960577,0.437475315514465,
-0.057319582917648));
#70627=CARTESIAN_POINT('Ctrl Pts',(0.27722954708371,0.648501002185801,-0.0414774694894131));
#70628=CARTESIAN_POINT('Ctrl Pts',(-0.0659690517919311,0.702185851024218,
-0.0256353560611776));
#70629=CARTESIAN_POINT('Ctrl Pts',(-0.393249524961131,0.58549190380499,
-0.0097932426329422));
#70630=CARTESIAN_POINT('Ctrl Pts',(-0.547685175284667,0.412997449882125,
0.000768166319214589));
#70631=CARTESIAN_POINT('Ctrl Pts',(-0.59969575964498,0.313508988489694,
0.00604887079529304));
#70632=CARTESIAN_POINT('Origin',(0.,0.,-0.0600000000000001));
#70633=CARTESIAN_POINT('',(0.8511,-1.04229689075431E-16,0.));
#70634=CARTESIAN_POINT('Origin',(0.,0.,0.));
#70635=CARTESIAN_POINT('Origin',(0.8511,-1.04229689075431E-16,-0.0600000000000001));
#70636=CARTESIAN_POINT('Origin',(0.,0.,-0.0600000000000001));
#70637=CARTESIAN_POINT('Origin',(0.,0.,0.));
#70638=CARTESIAN_POINT('',(1.2,-0.692820323027552,0.));
#70639=CARTESIAN_POINT('',(1.2,0.692820323027551,0.));
#70640=CARTESIAN_POINT('',(1.2,-0.692820323027552,0.));
#70641=CARTESIAN_POINT('',(-2.54538057293978E-16,-1.3856406460551,0.));
#70642=CARTESIAN_POINT('',(-2.54538057293978E-16,-1.3856406460551,0.));
#70643=CARTESIAN_POINT('',(-1.2,-0.692820323027551,0.));
#70644=CARTESIAN_POINT('',(-1.2,-0.692820323027551,0.));
#70645=CARTESIAN_POINT('',(-1.2,0.692820323027551,0.));
#70646=CARTESIAN_POINT('',(-1.2,0.692820323027551,0.));
#70647=CARTESIAN_POINT('',(8.48460190979926E-17,1.3856406460551,0.));
#70648=CARTESIAN_POINT('',(8.48460190979926E-17,1.3856406460551,0.));
#70649=CARTESIAN_POINT('',(1.2,0.692820323027551,0.));
#70650=CARTESIAN_POINT('Origin',(0.,0.,-1.425));
#70651=CARTESIAN_POINT('Origin',(0.,0.,0.914655896708346));
#70652=CARTESIAN_POINT('',(1.2,-0.692820323027552,0.858179306876173));
#70653=CARTESIAN_POINT('',(-2.54538057293978E-16,-1.3856406460551,0.858179306876173));
#70654=CARTESIAN_POINT('Ctrl Pts',(1.2,-0.692820323027552,0.858179306876173));
#70655=CARTESIAN_POINT('Ctrl Pts',(0.599999999999999,-1.03923048454133,
1.05817930687617));
#70656=CARTESIAN_POINT('Ctrl Pts',(-2.54538057293978E-16,-1.3856406460551,
0.858179306876173));
#70657=CARTESIAN_POINT('',(1.2,0.692820323027551,0.858179306876173));
#70658=CARTESIAN_POINT('Ctrl Pts',(1.2,0.692820323027551,0.858179306876173));
#70659=CARTESIAN_POINT('Ctrl Pts',(1.2,-6.66133814775094E-16,1.05817930687617));
#70660=CARTESIAN_POINT('Ctrl Pts',(1.2,-0.692820323027552,0.858179306876173));
#70661=CARTESIAN_POINT('',(8.48460190979925E-17,1.3856406460551,0.858179306876173));
#70662=CARTESIAN_POINT('Ctrl Pts',(8.48460190979925E-17,1.3856406460551,
0.858179306876173));
#70663=CARTESIAN_POINT('Ctrl Pts',(0.6,1.03923048454133,1.05817930687617));
#70664=CARTESIAN_POINT('Ctrl Pts',(1.2,0.692820323027551,0.858179306876173));
#70665=CARTESIAN_POINT('',(-1.2,0.692820323027551,0.858179306876173));
#70666=CARTESIAN_POINT('Ctrl Pts',(-1.2,0.692820323027551,0.858179306876173));
#70667=CARTESIAN_POINT('Ctrl Pts',(-0.600000000000001,1.03923048454133,
1.05817930687617));
#70668=CARTESIAN_POINT('Ctrl Pts',(8.48460190979925E-17,1.3856406460551,
0.858179306876173));
#70669=CARTESIAN_POINT('',(-1.2,-1.11389921653139E-16,0.965358983848622));
#70670=CARTESIAN_POINT('Ctrl Pts',(-1.2,-7.58222274085957E-17,0.965358983848622));
#70671=CARTESIAN_POINT('Ctrl Pts',(-1.2,0.321539030917347,0.965358983848622));
#70672=CARTESIAN_POINT('Ctrl Pts',(-1.2,0.692820323027551,0.858179306876173));
#70673=CARTESIAN_POINT('',(-1.14,-1.39609735102798E-16,1.));
#70674=CARTESIAN_POINT('',(-1.28782032302755,-1.5771250364726E-16,0.914655896708346));
#70675=CARTESIAN_POINT('Origin',(0.,0.,1.));
#70676=CARTESIAN_POINT('',(-1.2,-0.692820323027551,0.858179306876173));
#70677=CARTESIAN_POINT('Ctrl Pts',(-1.2,-0.692820323027551,0.858179306876173));
#70678=CARTESIAN_POINT('Ctrl Pts',(-1.2,-0.321539030917347,0.965358983848622));
#70679=CARTESIAN_POINT('Ctrl Pts',(-1.2,-7.58222274085957E-17,0.965358983848622));
#70680=CARTESIAN_POINT('Ctrl Pts',(-2.54538057293978E-16,-1.3856406460551,
0.858179306876173));
#70681=CARTESIAN_POINT('Ctrl Pts',(-0.599999999999999,-1.03923048454133,
1.05817930687617));
#70682=CARTESIAN_POINT('Ctrl Pts',(-1.2,-0.692820323027551,0.858179306876173));
#70683=CARTESIAN_POINT('Origin',(8.48460190979926E-17,1.3856406460551,0.));
#70684=CARTESIAN_POINT('',(8.48460190979926E-17,1.3856406460551,0.));
#70685=CARTESIAN_POINT('',(-1.2,0.692820323027551,0.));
#70686=CARTESIAN_POINT('Origin',(1.2,0.692820323027551,0.));
#70687=CARTESIAN_POINT('',(1.2,0.692820323027551,0.));
#70688=CARTESIAN_POINT('Origin',(1.2,-0.692820323027552,0.));
#70689=CARTESIAN_POINT('',(1.2,-0.692820323027552,0.));
#70690=CARTESIAN_POINT('Origin',(-2.54538057293978E-16,-1.3856406460551,
0.));
#70691=CARTESIAN_POINT('',(-2.54538057293978E-16,-1.3856406460551,0.));
#70692=CARTESIAN_POINT('Origin',(-1.2,-0.692820323027551,0.));
#70693=CARTESIAN_POINT('',(-1.2,-0.692820323027551,0.));
#70694=CARTESIAN_POINT('Origin',(-1.2,0.692820323027551,0.));
#70695=CARTESIAN_POINT('Origin',(0.,0.,1.));
#70696=CARTESIAN_POINT('Origin',(0.7,0.,-3.));
#70697=CARTESIAN_POINT('',(-0.7,-8.57252759403147E-17,-3.));
#70698=CARTESIAN_POINT('Origin',(0.,0.,-3.));
#70699=CARTESIAN_POINT('Origin',(0.,0.,-2.95));
#70700=CARTESIAN_POINT('',(-0.75,-9.18485099360515E-17,-2.95));
#70739=UNCERTAINTY_MEASURE_WITH_UNIT(LENGTH_MEASURE(0.001),#70758,
'DISTANCE_ACCURACY_VALUE',
'Maximum model space distance between geometric entities at asserted c
onnectivities');
#70740=UNCERTAINTY_MEASURE_WITH_UNIT(LENGTH_MEASURE(0.001),#70758,
'DISTANCE_ACCURACY_VALUE',
'Maximum model space distance between geometric entities at asserted c
onnectivities');
#70756=(
GEOMETRIC_REPRESENTATION_CONTEXT(3)
GLOBAL_UNCERTAINTY_ASSIGNED_CONTEXT((#70739))
GLOBAL_UNIT_ASSIGNED_CONTEXT((#70758,#70760,#70761))
REPRESENTATION_CONTEXT('','3D')
);
#70757=(
GEOMETRIC_REPRESENTATION_CONTEXT(3)
GLOBAL_UNCERTAINTY_ASSIGNED_CONTEXT((#70740))
GLOBAL_UNIT_ASSIGNED_CONTEXT((#70758,#70760,#70761))
REPRESENTATION_CONTEXT('','3D')
);
#70758=(
LENGTH_UNIT()
NAMED_UNIT(*)
SI_UNIT(.CENTI.,.METRE.)
);
#70760=(
NAMED_UNIT(*)
PLANE_ANGLE_UNIT()
SI_UNIT($,.RADIAN.)
);
#70761=(
NAMED_UNIT(*)
SI_UNIT($,.STERADIAN.)
SOLID_ANGLE_UNIT()
);
#70777=SHAPE_DEFINITION_REPRESENTATION(#70793,#70832);
#70793=PRODUCT_DEFINITION_SHAPE('',$,#70849);
#70832=SHAPE_REPRESENTATION('',(#28892),#70756);
#70833=PRODUCT_DEFINITION_CONTEXT('part definition',#70883,'design');
#70849=PRODUCT_DEFINITION('2026-10-19-03-03-09-768',
'13_ISO_4017_M16x30_Ram_Depth_Stop_Screw',#70865,#70833);
#70865=PRODUCT_DEFINITION_FORMATION('',$,#70900);
#70883=APPLICATION_CONTEXT(
'Core Data for Automotive Mechanical Design Process');
#70884=PRODUCT_CONTEXT('part definition',#70883,'mechanical');
#70900=PRODUCT('2026-10-19-03-03-09-768',
'13_ISO_4017_M16x30_Ram_Depth_Stop_Screw',$,(#70884));
#71048=COLOUR_RGB('Black',0.12,0.14,0.17);
#71049=FILL_AREA_STYLE_COLOUR('',#71048);
#71050=FILL_AREA_STYLE('',(#71049));
#71051=SURFACE_STYLE_FILL_AREA(#71050);
#71052=SURFACE_SIDE_STYLE('',(#71051));
#71053=SURFACE_STYLE_USAGE(.BOTH.,#71052);
#71054=PRESENTATION_STYLE_ASSIGNMENT((#71053));
ENDSEC;
END-ISO-10303-21;
